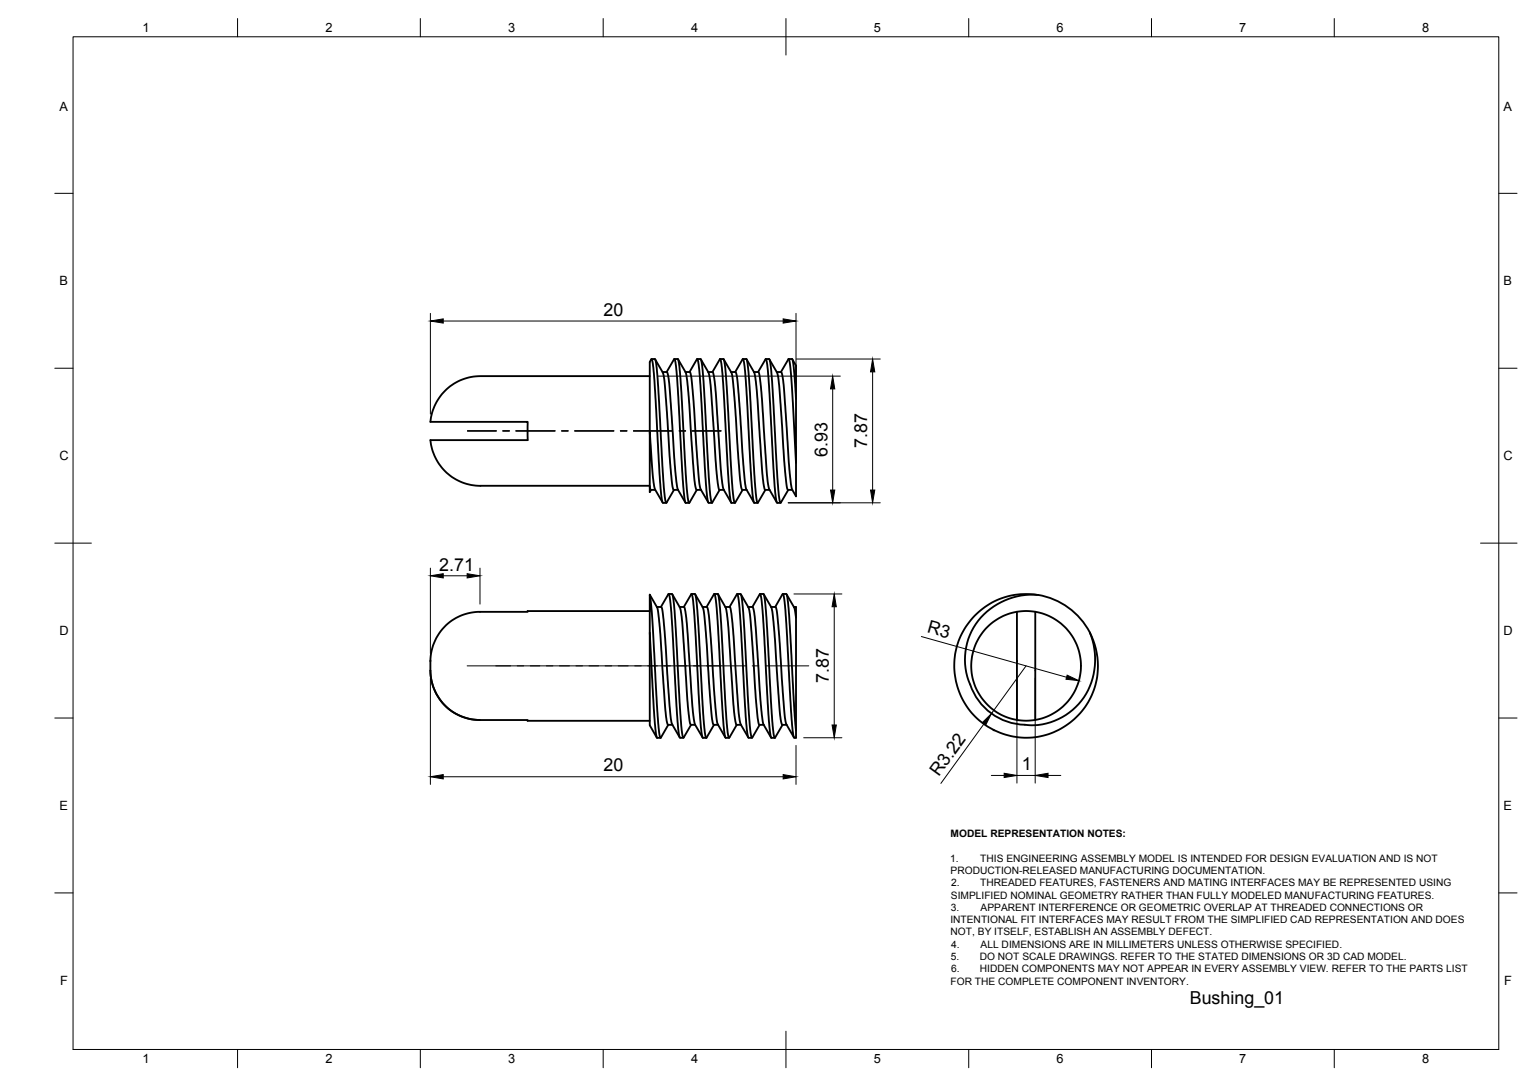
ISO-10303-21;
HEADER;
/* Generated by software containing ST-Developer
 * from STEP Tools, Inc. (www.steptools.com) 
 */

FILE_DESCRIPTION(
/* description */ (''),
/* implementation_level */ '2;1');

FILE_NAME(
/* name */ 'Bushing_01.step',
/* time_stamp */ '2026-10-06T12:52:28-07:00',
/* author */ (''),
/* organization */ (''),
/* preprocessor_version */ 'ST-DEVELOPER v20.2',
/* originating_system */ 'Autodesk Translation Framework v15.15.0.0',
/* authorisation */ '');

FILE_SCHEMA (('AUTOMOTIVE_DESIGN { 1 0 10303 214 3 1 1 }'));
ENDSEC;

DATA;
#10=MECHANICAL_DESIGN_GEOMETRIC_PRESENTATION_REPRESENTATION('',(#77),#34403);
#47=B_SPLINE_SURFACE_WITH_KNOTS('',3,3,((#18145,#18146,#18147,#18148,#18149,
#18150,#18151,#18152,#18153),(#18154,#18155,#18156,#18157,#18158,#18159,
#18160,#18161,#18162),(#18163,#18164,#18165,#18166,#18167,#18168,#18169,
#18170,#18171),(#18172,#18173,#18174,#18175,#18176,#18177,#18178,#18179,
#18180),(#18181,#18182,#18183,#18184,#18185,#18186,#18187,#18188,#18189)),
 .UNSPECIFIED.,.F.,.F.,.F.,(4,1,4),(4,1,1,1,1,1,4),(-2.31295147948379E-5,
0.571428571428571,1.),(-0.0392722280793192,-0.0280568740573752,-0.00562616601348723,
0.00558918800845676,0.0168045420304008,0.0280198960523448,0.0392352500742888),
 .UNSPECIFIED.);
#48=B_SPLINE_SURFACE_WITH_KNOTS('',3,3,((#18360,#18361,#18362,#18363,#18364,
#18365,#18366,#18367,#18368,#18369),(#18370,#18371,#18372,#18373,#18374,
#18375,#18376,#18377,#18378,#18379),(#18380,#18381,#18382,#18383,#18384,
#18385,#18386,#18387,#18388,#18389),(#18390,#18391,#18392,#18393,#18394,
#18395,#18396,#18397,#18398,#18399),(#18400,#18401,#18402,#18403,#18404,
#18405,#18406,#18407,#18408,#18409)),.UNSPECIFIED.,.F.,.F.,.F.,(4,1,4),
(4,1,1,1,1,1,1,4),(-2.35337788502184E-5,0.571428571428571,1.),(-0.0392722280793192,
-0.0280568740573752,-0.0168415200354311,-0.00562616601348712,0.0055891880084569,
0.0168045420304009,0.0280198960523449,0.0392352500742889),.UNSPECIFIED.);
#49=B_SPLINE_SURFACE_WITH_KNOTS('',3,3,((#18444,#18445,#18446,#18447,#18448,
#18449,#18450,#18451,#18452,#18453,#18454,#18455,#18456,#18457,#18458,#18459,
#18460,#18461,#18462,#18463,#18464,#18465,#18466,#18467,#18468,#18469,#18470,
#18471,#18472,#18473,#18474,#18475,#18476,#18477,#18478,#18479,#18480,#18481,
#18482,#18483,#18484,#18485,#18486,#18487,#18488,#18489),(#18490,#18491,
#18492,#18493,#18494,#18495,#18496,#18497,#18498,#18499,#18500,#18501,#18502,
#18503,#18504,#18505,#18506,#18507,#18508,#18509,#18510,#18511,#18512,#18513,
#18514,#18515,#18516,#18517,#18518,#18519,#18520,#18521,#18522,#18523,#18524,
#18525,#18526,#18527,#18528,#18529,#18530,#18531,#18532,#18533,#18534,#18535),
(#18536,#18537,#18538,#18539,#18540,#18541,#18542,#18543,#18544,#18545,
#18546,#18547,#18548,#18549,#18550,#18551,#18552,#18553,#18554,#18555,#18556,
#18557,#18558,#18559,#18560,#18561,#18562,#18563,#18564,#18565,#18566,#18567,
#18568,#18569,#18570,#18571,#18572,#18573,#18574,#18575,#18576,#18577,#18578,
#18579,#18580,#18581),(#18582,#18583,#18584,#18585,#18586,#18587,#18588,
#18589,#18590,#18591,#18592,#18593,#18594,#18595,#18596,#18597,#18598,#18599,
#18600,#18601,#18602,#18603,#18604,#18605,#18606,#18607,#18608,#18609,#18610,
#18611,#18612,#18613,#18614,#18615,#18616,#18617,#18618,#18619,#18620,#18621,
#18622,#18623,#18624,#18625,#18626,#18627)),.UNSPECIFIED.,.F.,.F.,.F.,(4,
4),(4,1,1,1,1,1,1,1,1,1,1,1,1,1,1,1,1,1,1,1,1,1,1,1,1,1,1,1,1,1,1,1,1,1,
1,1,1,1,1,1,1,1,1,4),(-0.000633807887895752,0.0823317564776454),(8.31473274985803,
9.29783943738047,10.2809461249029,11.2640528124254,12.2471594999478,13.2302661874702,
14.2133728749927,15.1964795625151,16.1795862500376,17.16269293756,18.1457996250825,
19.1289063126049,20.1120130001274,21.0951196876498,22.0782263751723,23.0613330626947,
24.0444397502171,25.0275464377396,26.010653125262,26.9937598127845,27.9768665003069,
28.9599731878294,29.9430798753518,30.9261865628743,31.9092932503967,32.8923999379191,
33.8755066254416,34.858613312964,35.8417200004865,36.8248266880089,37.8079333755314,
38.7910400630538,39.7741467505763,40.7572534380987,41.7403601256211,42.7234668131436,
43.706573500666,44.6896801881885,45.6727868757109,46.6558935632334,47.6390002507558,
48.6221069382783,49.6052136258007,50.5889541212111),.UNSPECIFIED.);
#50=B_SPLINE_SURFACE_WITH_KNOTS('',3,3,((#18809,#18810,#18811,#18812,#18813,
#18814,#18815,#18816,#18817,#18818,#18819,#18820,#18821,#18822,#18823,#18824,
#18825,#18826,#18827,#18828,#18829,#18830,#18831,#18832,#18833,#18834,#18835,
#18836,#18837,#18838,#18839,#18840,#18841,#18842,#18843,#18844,#18845,#18846,
#18847,#18848,#18849,#18850,#18851,#18852,#18853,#18854),(#18855,#18856,
#18857,#18858,#18859,#18860,#18861,#18862,#18863,#18864,#18865,#18866,#18867,
#18868,#18869,#18870,#18871,#18872,#18873,#18874,#18875,#18876,#18877,#18878,
#18879,#18880,#18881,#18882,#18883,#18884,#18885,#18886,#18887,#18888,#18889,
#18890,#18891,#18892,#18893,#18894,#18895,#18896,#18897,#18898,#18899,#18900),
(#18901,#18902,#18903,#18904,#18905,#18906,#18907,#18908,#18909,#18910,
#18911,#18912,#18913,#18914,#18915,#18916,#18917,#18918,#18919,#18920,#18921,
#18922,#18923,#18924,#18925,#18926,#18927,#18928,#18929,#18930,#18931,#18932,
#18933,#18934,#18935,#18936,#18937,#18938,#18939,#18940,#18941,#18942,#18943,
#18944,#18945,#18946),(#18947,#18948,#18949,#18950,#18951,#18952,#18953,
#18954,#18955,#18956,#18957,#18958,#18959,#18960,#18961,#18962,#18963,#18964,
#18965,#18966,#18967,#18968,#18969,#18970,#18971,#18972,#18973,#18974,#18975,
#18976,#18977,#18978,#18979,#18980,#18981,#18982,#18983,#18984,#18985,#18986,
#18987,#18988,#18989,#18990,#18991,#18992)),.UNSPECIFIED.,.F.,.F.,.F.,(4,
4),(4,1,1,1,1,1,1,1,1,1,1,1,1,1,1,1,1,1,1,1,1,1,1,1,1,1,1,1,1,1,1,1,1,1,
1,1,1,1,1,1,1,1,1,4),(-0.000319018948610172,0.0826465308545402),(11.6145803026385,
12.5983209152772,13.5814276027996,14.564534290322,15.5476409778445,16.5307476653669,
17.5138543528894,18.4969610404118,19.4800677279343,20.4631744154567,21.4462811029792,
22.4293877905016,23.4124944780241,24.3956011655465,25.3787078530689,26.3618145405914,
27.3449212281138,28.3280279156363,29.3111346031587,30.2942412906812,31.2773479782036,
32.2604546657261,33.2435613532485,34.226668040771,35.2097747282934,36.1928814158158,
37.1759881033383,38.1590947908607,39.1422014783832,40.1253081659056,41.1084148534281,
42.0915215409505,43.074628228473,44.0577349159954,45.0408416035178,46.0239482910403,
47.0070549785627,47.9901616660852,48.9732683536076,49.9563750411301,50.9394817286525,
51.922588416175,52.9056951036974,53.8888017912198),.UNSPECIFIED.);
#61=SHAPE_REPRESENTATION_RELATIONSHIP('SRR','None',#34439,#69);
#69=ADVANCED_BREP_SHAPE_REPRESENTATION('',(#85),#34399);
#77=STYLED_ITEM('',(#34484),#85);
#85=MANIFOLD_SOLID_BREP('Body1',#4386);
#100=FACE_BOUND('',#818,.T.);
#135=PLANE('',#4570);
#136=PLANE('',#4574);
#137=PLANE('',#4577);
#138=PLANE('',#4578);
#192=CIRCLE('',#4559,3.22275);
#193=CIRCLE('',#4566,3.933);
#194=CIRCLE('',#4567,3.933);
#195=CIRCLE('',#4569,3.22275);
#196=CIRCLE('',#4571,24.5);
#197=CIRCLE('',#4573,3.);
#198=CIRCLE('',#4575,24.5);
#559=FACE_OUTER_BOUND('',#801,.T.);
#560=FACE_OUTER_BOUND('',#802,.T.);
#561=FACE_OUTER_BOUND('',#803,.T.);
#562=FACE_OUTER_BOUND('',#804,.T.);
#563=FACE_OUTER_BOUND('',#805,.T.);
#564=FACE_OUTER_BOUND('',#806,.T.);
#565=FACE_OUTER_BOUND('',#807,.T.);
#566=FACE_OUTER_BOUND('',#808,.T.);
#567=FACE_OUTER_BOUND('',#809,.T.);
#568=FACE_OUTER_BOUND('',#810,.T.);
#569=FACE_OUTER_BOUND('',#811,.T.);
#570=FACE_OUTER_BOUND('',#812,.T.);
#571=FACE_OUTER_BOUND('',#813,.T.);
#572=FACE_OUTER_BOUND('',#814,.T.);
#573=FACE_OUTER_BOUND('',#815,.T.);
#574=FACE_OUTER_BOUND('',#816,.T.);
#575=FACE_OUTER_BOUND('',#817,.T.);
#576=FACE_OUTER_BOUND('',#819,.T.);
#801=EDGE_LOOP('',(#2953,#2954,#2955,#2956));
#802=EDGE_LOOP('',(#2957,#2958,#2959,#2960));
#803=EDGE_LOOP('',(#2961,#2962,#2963,#2964));
#804=EDGE_LOOP('',(#2965,#2966,#2967,#2968));
#805=EDGE_LOOP('',(#2969,#2970,#2971,#2972));
#806=EDGE_LOOP('',(#2973,#2974,#2975,#2976));
#807=EDGE_LOOP('',(#2977,#2978,#2979,#2980,#2981,#2982,#2983,#2984,#2985,
#2986,#2987,#2988,#2989,#2990,#2991,#2992,#2993,#2994));
#808=EDGE_LOOP('',(#2995,#2996,#2997,#2998));
#809=EDGE_LOOP('',(#2999,#3000,#3001,#3002));
#810=EDGE_LOOP('',(#3003,#3004,#3005,#3006,#3007,#3008));
#811=EDGE_LOOP('',(#3009,#3010,#3011,#3012,#3013,#3014,#3015,#3016,#3017,
#3018,#3019,#3020));
#812=EDGE_LOOP('',(#3021,#3022,#3023,#3024,#3025));
#813=EDGE_LOOP('',(#3026,#3027,#3028,#3029,#3030,#3031));
#814=EDGE_LOOP('',(#3032,#3033,#3034,#3035));
#815=EDGE_LOOP('',(#3036,#3037,#3038,#3039,#3040,#3041,#3042,#3043,#3044,
#3045,#3046,#3047,#3048,#3049,#3050,#3051,#3052,#3053));
#816=EDGE_LOOP('',(#3054,#3055,#3056,#3057,#3058,#3059,#3060,#3061,#3062,
#3063,#3064,#3065,#3066,#3067,#3068,#3069,#3070,#3071));
#817=EDGE_LOOP('',(#3072,#3073,#3074,#3075,#3076));
#818=EDGE_LOOP('',(#3077));
#819=EDGE_LOOP('',(#3078,#3079,#3080,#3081,#3082));
#1040=LINE('',#13648,#1177);
#1041=LINE('',#13847,#1178);
#1042=LINE('',#14169,#1179);
#1043=LINE('',#14491,#1180);
#1044=LINE('',#14817,#1181);
#1045=LINE('',#15137,#1182);
#1046=LINE('',#18231,#1183);
#1047=LINE('',#18234,#1184);
#1048=LINE('',#18237,#1185);
#1049=LINE('',#18291,#1186);
#1050=LINE('',#18307,#1187);
#1051=LINE('',#18358,#1188);
#1052=LINE('',#18440,#1189);
#1177=VECTOR('',#5189,3.22275);
#1178=VECTOR('',#5194,3.22275);
#1179=VECTOR('',#5197,3.22275);
#1180=VECTOR('',#5200,3.22275);
#1181=VECTOR('',#5203,3.22275);
#1182=VECTOR('',#5206,3.22275);
#1183=VECTOR('',#5217,10.);
#1184=VECTOR('',#5220,10.);
#1185=VECTOR('',#5223,10.);
#1186=VECTOR('',#5226,10.);
#1187=VECTOR('',#5227,10.);
#1188=VECTOR('',#5228,3.);
#1189=VECTOR('',#5231,10.);
#1365=B_SPLINE_CURVE_WITH_KNOTS('',3,(#13650,#13651,#13652,#13653,#13654,
#13655,#13656,#13657,#13658,#13659,#13660,#13661,#13662,#13663,#13664,#13665,
#13666,#13667,#13668,#13669,#13670,#13671,#13672,#13673,#13674,#13675,#13676,
#13677,#13678,#13679,#13680,#13681,#13682,#13683,#13684,#13685,#13686,#13687,
#13688,#13689,#13690,#13691,#13692,#13693,#13694,#13695,#13696,#13697,#13698,
#13699,#13700,#13701,#13702,#13703,#13704,#13705,#13706,#13707,#13708,#13709,
#13710,#13711,#13712,#13713,#13714,#13715,#13716,#13717,#13718,#13719,#13720,
#13721,#13722,#13723,#13724,#13725,#13726,#13727,#13728,#13729,#13730,#13731,
#13732,#13733,#13734,#13735,#13736,#13737,#13738,#13739,#13740,#13741,#13742,
#13743,#13744,#13745,#13746,#13747,#13748,#13749,#13750,#13751,#13752,#13753,
#13754,#13755,#13756,#13757,#13758,#13759),.UNSPECIFIED.,.F.,.F.,(4,2,2,
2,2,2,2,2,2,2,2,2,2,2,2,2,2,2,2,2,2,2,2,2,2,2,2,2,2,2,2,2,2,2,2,2,2,2,2,
2,2,2,2,2,2,2,2,2,2,2,2,2,2,2,4),(-1.46839216655186,-1.42833493122557,-1.40983960309952,
-1.39649008476235,-1.38192245258612,-1.35595026682801,-1.32006579388245,
-1.25739415958123,-1.24599994074249,-1.23838263735435,-1.2292335836828,
-1.20895486413597,-1.17609120945209,-1.11172712552003,-1.09300158666968,
-1.07960228916858,-1.06507837657971,-1.03947664653156,-1.00445705495045,
-0.941126403182701,-0.929252655631959,-0.921667552812672,-0.912906557233483,
-0.894754745947669,-0.867289011584784,-0.789797140050929,-0.772858151395854,
-0.759724672664605,-0.744718751329267,-0.715589302934294,-0.671818863481682,
-0.624725490925685,-0.612046960332389,-0.605030943441965,-0.596793484943762,
-0.581814683947116,-0.521809333456173,-0.475770727809289,-0.456880324092417,
-0.443431024636274,-0.428912818539185,-0.40347690482787,-0.368790757052006,
-0.305998460037176,-0.293741810698422,-0.286007401773675,-0.277001834303914,
-0.2582504497825,-0.229364741447431,-0.158963286891711,-0.141351957341446,
-0.127920650801248,-0.112746328135276,-0.0837659472426957,-0.00482640158894297),
 .UNSPECIFIED.);
#1366=B_SPLINE_CURVE_WITH_KNOTS('',3,(#13762,#13763,#13764,#13765,#13766,
#13767,#13768,#13769,#13770,#13771,#13772,#13773,#13774,#13775,#13776,#13777,
#13778,#13779,#13780,#13781,#13782,#13783,#13784,#13785,#13786,#13787,#13788,
#13789,#13790,#13791,#13792,#13793,#13794,#13795,#13796,#13797,#13798,#13799,
#13800,#13801,#13802,#13803,#13804,#13805,#13806,#13807,#13808,#13809,#13810,
#13811,#13812,#13813,#13814,#13815,#13816,#13817,#13818,#13819,#13820,#13821,
#13822,#13823,#13824,#13825,#13826,#13827,#13828,#13829,#13830,#13831,#13832,
#13833,#13834,#13835,#13836,#13837,#13838,#13839,#13840,#13841,#13842,#13843),
 .UNSPECIFIED.,.F.,.F.,(4,2,2,2,2,2,2,2,2,2,2,2,2,2,2,2,2,2,2,2,2,2,2,2,
2,2,2,2,2,2,2,2,2,2,2,2,2,2,2,2,4),(-12.9928680261101,-12.9859224043785,
-12.9767663441379,-12.9317684829387,-12.8787491107298,-12.8585962440726,
-12.843864647075,-12.8272831513426,-12.7952673642781,-12.7272779370865,
-12.7034734144216,-12.6867491934808,-12.6781417326004,-12.6706722689398,
-12.6588036168692,-12.5925791120038,-12.559965517409,-12.5357561764214,
-12.5219312356032,-12.5092183047936,-12.4916768823375,-12.4031982185048,
-12.3811372405126,-12.3655143239889,-12.3574349585401,-12.3497117864246,
-12.3373035405743,-12.2745292128648,-12.239536256517,-12.2138553471672,
-12.1992108316161,-12.185635321062,-12.1695331810739,-12.0996377675633,
-12.0705351122928,-12.0517005184064,-12.0426844314299,-12.034958762972,
-12.0227451090155,-11.9599676349854,-11.9265167435349),.UNSPECIFIED.);
#1367=B_SPLINE_CURVE_WITH_KNOTS('',3,(#13848,#13849,#13850,#13851,#13852,
#13853,#13854,#13855,#13856,#13857,#13858,#13859,#13860,#13861,#13862,#13863,
#13864,#13865,#13866,#13867,#13868,#13869,#13870,#13871,#13872,#13873,#13874,
#13875,#13876,#13877,#13878,#13879,#13880,#13881,#13882,#13883,#13884,#13885,
#13886,#13887,#13888,#13889,#13890,#13891,#13892,#13893,#13894,#13895,#13896,
#13897,#13898,#13899,#13900,#13901,#13902,#13903,#13904,#13905,#13906,#13907,
#13908,#13909,#13910,#13911,#13912,#13913,#13914,#13915,#13916,#13917,#13918,
#13919,#13920,#13921,#13922,#13923,#13924,#13925,#13926,#13927,#13928,#13929,
#13930,#13931,#13932,#13933,#13934,#13935,#13936,#13937,#13938,#13939,#13940,
#13941,#13942,#13943,#13944,#13945,#13946,#13947,#13948,#13949,#13950,#13951,
#13952,#13953,#13954,#13955,#13956,#13957,#13958,#13959,#13960,#13961,#13962,
#13963,#13964,#13965,#13966,#13967,#13968,#13969,#13970,#13971,#13972,#13973,
#13974,#13975,#13976,#13977,#13978,#13979,#13980,#13981,#13982,#13983,#13984,
#13985,#13986,#13987,#13988,#13989,#13990,#13991,#13992,#13993,#13994,#13995,
#13996,#13997,#13998,#13999,#14000,#14001,#14002,#14003,#14004,#14005,#14006,
#14007),.UNSPECIFIED.,.F.,.F.,(4,2,2,2,2,2,2,2,2,2,2,2,2,2,2,2,2,2,2,2,
2,2,2,2,2,2,2,2,2,2,2,2,2,2,2,2,2,2,2,2,2,2,2,2,2,2,2,2,2,2,2,2,2,2,2,2,
2,2,2,2,2,2,2,2,2,2,2,2,2,2,2,2,2,2,2,2,2,2,2,4),(-3.49867878100114,-3.48078195894374,
-3.46955972522698,-3.46197286794586,-3.45277159842556,-3.43205243267988,
-3.39797610063354,-3.33546990288741,-3.31654806244602,-3.30313938427867,
-3.28872610459223,-3.263693666223,-3.22988764964021,-3.16560395356786,-3.15313346501676,
-3.14544256963846,-3.13683534548366,-3.11979450354527,-3.09492308948557,
-3.01527193149294,-2.99739186424985,-2.98411787341524,-2.96928256762587,
-2.94165310746421,-2.90187154715814,-2.84744108782649,-2.83519835180177,
-2.82754492556646,-2.81885783486495,-2.80134935179091,-2.77541919752302,
-2.69874979137671,-2.68038057439865,-2.66704941358868,-2.65243562926348,
-2.6261741549808,-2.58964121940858,-2.52834010486826,-2.51679218417816,
-2.50916638327307,-2.50014259245465,-2.48058056285362,-2.44963644828718,
-2.38085364722827,-2.36257423529482,-2.3492540741215,-2.33460217519332,
-2.30810824640674,-2.27103873044209,-2.21095127043577,-2.19926909881182,
-2.19162334288848,-2.18265751788382,-2.1634770024513,-2.13351351801827,
-2.06259963370997,-2.04459412536108,-2.03130461939912,-2.016525598512,-1.98925576826921,
-1.95035384678123,-1.89421291245162,-1.88210670171816,-1.87447641278316,
-1.86574577853761,-1.84795589000478,-1.82136965309309,-1.74647395934031,
-1.72781643493424,-1.71445588254354,-1.69997280638284,-1.67445876507744,
-1.6395921546019,-1.57666462581832,-1.56449569108919,-1.55685831797228,
-1.54815224960004,-1.53052436699322,-1.50432028007254,-1.46839216655186),
 .UNSPECIFIED.);
#1368=B_SPLINE_CURVE_WITH_KNOTS('',3,(#14008,#14009,#14010,#14011,#14012,
#14013,#14014,#14015,#14016,#14017,#14018,#14019,#14020,#14021,#14022,#14023,
#14024,#14025,#14026,#14027,#14028,#14029,#14030,#14031,#14032,#14033,#14034,
#14035,#14036,#14037,#14038,#14039,#14040,#14041,#14042,#14043,#14044,#14045,
#14046,#14047,#14048,#14049,#14050,#14051,#14052,#14053,#14054,#14055,#14056,
#14057,#14058,#14059,#14060,#14061,#14062,#14063,#14064,#14065,#14066,#14067,
#14068,#14069,#14070,#14071,#14072,#14073,#14074,#14075,#14076,#14077,#14078,
#14079,#14080,#14081,#14082,#14083,#14084,#14085,#14086,#14087,#14088,#14089,
#14090,#14091,#14092,#14093,#14094,#14095,#14096,#14097,#14098,#14099,#14100,
#14101,#14102,#14103,#14104,#14105,#14106,#14107,#14108,#14109,#14110,#14111,
#14112,#14113,#14114,#14115,#14116,#14117,#14118,#14119,#14120,#14121,#14122,
#14123,#14124,#14125,#14126,#14127,#14128,#14129,#14130,#14131,#14132,#14133,
#14134,#14135,#14136,#14137,#14138,#14139,#14140,#14141,#14142,#14143,#14144,
#14145,#14146,#14147,#14148,#14149,#14150,#14151,#14152,#14153,#14154,#14155,
#14156,#14157,#14158,#14159,#14160,#14161,#14162,#14163,#14164,#14165),
 .UNSPECIFIED.,.F.,.F.,(4,2,2,2,2,2,2,2,2,2,2,2,2,2,2,2,2,2,2,2,2,2,2,2,
2,2,2,2,2,2,2,2,2,2,2,2,2,2,2,2,2,2,2,2,2,2,2,2,2,2,2,2,2,2,2,2,2,2,2,2,
2,2,2,2,2,2,2,2,2,2,2,2,2,2,2,2,2,2,4),(-11.9265167435349,-11.9253010671319,
-11.8998775010244,-11.8853659903058,-11.8719222083261,-11.853038636317,
-11.8070670854776,-11.7469950171144,-11.732009875923,-11.7237734567874,
-11.7167614908132,-11.7040962421554,-11.657144644663,-11.613348594958,-11.5842158731154,
-11.5692140131739,-11.5560858712183,-11.5391563059077,-11.4616146846684,
-11.4341620971523,-11.4160188349624,-11.4072614323029,-11.3996791529454,
-11.3878096466355,-11.3295052301493,-11.2916491109299,-11.2648076084194,
-11.2500856128337,-11.2367575434473,-11.2185487998283,-11.1495201728474,
-11.1188782881042,-11.0994366818601,-11.0904187427783,-11.0827715924609,
-11.0711299783697,-11.0108006877799,-10.9739293014615,-10.9475272769351,
-10.9328929903791,-10.919570571438,-10.9012581537384,-10.8241647393242,
-10.7983532562927,-10.7808988714022,-10.7722242463342,-10.7645771798208,
-10.7523362255452,-10.6981722958883,-10.6583176476268,-10.6306685501689,
-10.6158432715508,-10.602589118057,-10.5847552249583,-10.5125151252235,
-10.4830685178717,-10.4640972285704,-10.4551729237098,-10.4475245495813,
-10.4357933954727,-10.3762476656135,-10.3389794411438,-10.3124002139746,
-10.2977349418755,-10.2844183959626,-10.2661684350075,-10.1971897108364,
-10.1663518150652,-10.1468330124204,-10.137815162146,-10.1301865446066,
-10.1186200205451,-10.057586096903,-10.0209901905299,-9.99470377217364,
-9.98008828052383,-9.96676098275258,-9.94840609177415,-9.89731205748756),
 .UNSPECIFIED.);
#1369=B_SPLINE_CURVE_WITH_KNOTS('',3,(#14170,#14171,#14172,#14173,#14174,
#14175,#14176,#14177,#14178,#14179,#14180,#14181,#14182,#14183,#14184,#14185,
#14186,#14187,#14188,#14189,#14190,#14191,#14192,#14193,#14194,#14195,#14196,
#14197,#14198,#14199,#14200,#14201,#14202,#14203,#14204,#14205,#14206,#14207,
#14208,#14209,#14210,#14211,#14212,#14213,#14214,#14215,#14216,#14217,#14218,
#14219,#14220,#14221,#14222,#14223,#14224,#14225,#14226,#14227,#14228,#14229,
#14230,#14231,#14232,#14233,#14234,#14235,#14236,#14237,#14238,#14239,#14240,
#14241,#14242,#14243,#14244,#14245,#14246,#14247,#14248,#14249,#14250,#14251,
#14252,#14253,#14254,#14255,#14256,#14257,#14258,#14259,#14260,#14261,#14262,
#14263,#14264,#14265,#14266,#14267,#14268,#14269,#14270,#14271,#14272,#14273,
#14274,#14275,#14276,#14277,#14278,#14279,#14280,#14281,#14282,#14283,#14284,
#14285,#14286,#14287,#14288,#14289,#14290,#14291,#14292,#14293,#14294,#14295,
#14296,#14297,#14298,#14299,#14300,#14301,#14302,#14303,#14304,#14305,#14306,
#14307,#14308,#14309,#14310,#14311,#14312,#14313,#14314,#14315,#14316,#14317,
#14318,#14319,#14320,#14321,#14322,#14323,#14324,#14325,#14326,#14327),
 .UNSPECIFIED.,.F.,.F.,(4,2,2,2,2,2,2,2,2,2,2,2,2,2,2,2,2,2,2,2,2,2,2,2,
2,2,2,2,2,2,2,2,2,2,2,2,2,2,2,2,2,2,2,2,2,2,2,2,2,2,2,2,2,2,2,2,2,2,2,2,
2,2,2,2,2,2,2,2,2,2,2,2,2,2,2,2,2,2,4),(-5.52967993174404,-5.52746103895827,
-5.51301726605171,-5.48781751392462,-5.45365608075187,-5.39023974331564,
-5.37763154077627,-5.37060511658607,-5.36232751823559,-5.34710774761743,
-5.32609931402627,-5.2862261887768,-5.24174894981634,-5.22298786851781,
-5.2095987033326,-5.19512334302082,-5.16973497836552,-5.13516395069695,
-5.07314639039331,-5.06018581576942,-5.05310310809778,-5.04492307594188,
-5.03021949666535,-5.01023868726809,-4.94186884287386,-4.91337098939853,
-4.89839769785815,-4.88514869317986,-4.86752871096216,-4.80838931035308,
-4.75396056823127,-4.74171236882094,-4.734055979712,-4.72536542702825,-4.70785112905183,
-4.68191322298387,-4.60521466097691,-4.58683882554718,-4.57350193498445,
-4.5588808435482,-4.53260225217019,-4.49603942555881,-4.43475512973231,
-4.42319834572813,-4.41556866284627,-4.40654243879864,-4.38698036174205,
-4.35604271661056,-4.28721316259916,-4.26893202003434,-4.25560773622987,
-4.24094857896087,-4.21443280452239,-4.17732242330325,-4.11726652960083,
-4.10557436659351,-4.0979264437805,-4.08896619952871,-4.06982003452643,
-4.03994975453202,-3.96871964483552,-3.95074163312683,-3.93745485665172,
-3.92266291296092,-3.89531644100836,-3.85623277292381,-3.80042416657247,
-3.7882820156738,-3.78064331846076,-3.7719145791267,-3.75417031696167,-3.7276991511797,
-3.65248254650758,-3.63386775502272,-3.62050141253184,-3.60597794025483,
-3.58028256336171,-3.54503001769459,-3.49867878100114),.UNSPECIFIED.);
#1370=B_SPLINE_CURVE_WITH_KNOTS('',3,(#14328,#14329,#14330,#14331,#14332,
#14333,#14334,#14335,#14336,#14337,#14338,#14339,#14340,#14341,#14342,#14343,
#14344,#14345,#14346,#14347,#14348,#14349,#14350,#14351,#14352,#14353,#14354,
#14355,#14356,#14357,#14358,#14359,#14360,#14361,#14362,#14363,#14364,#14365,
#14366,#14367,#14368,#14369,#14370,#14371,#14372,#14373,#14374,#14375,#14376,
#14377,#14378,#14379,#14380,#14381,#14382,#14383,#14384,#14385,#14386,#14387,
#14388,#14389,#14390,#14391,#14392,#14393,#14394,#14395,#14396,#14397,#14398,
#14399,#14400,#14401,#14402,#14403,#14404,#14405,#14406,#14407,#14408,#14409,
#14410,#14411,#14412,#14413,#14414,#14415,#14416,#14417,#14418,#14419,#14420,
#14421,#14422,#14423,#14424,#14425,#14426,#14427,#14428,#14429,#14430,#14431,
#14432,#14433,#14434,#14435,#14436,#14437,#14438,#14439,#14440,#14441,#14442,
#14443,#14444,#14445,#14446,#14447,#14448,#14449,#14450,#14451,#14452,#14453,
#14454,#14455,#14456,#14457,#14458,#14459,#14460,#14461,#14462,#14463,#14464,
#14465,#14466,#14467,#14468,#14469,#14470,#14471,#14472,#14473,#14474,#14475,
#14476,#14477,#14478,#14479,#14480,#14481,#14482,#14483,#14484,#14485,#14486,
#14487),.UNSPECIFIED.,.F.,.F.,(4,2,2,2,2,2,2,2,2,2,2,2,2,2,2,2,2,2,2,2,
2,2,2,2,2,2,2,2,2,2,2,2,2,2,2,2,2,2,2,2,2,2,2,2,2,2,2,2,2,2,2,2,2,2,2,2,
2,2,2,2,2,2,2,2,2,2,2,2,2,2,2,2,2,2,2,2,2,2,2,4),(-9.89731205748756,-9.87162361382395,
-9.84571672148278,-9.8282203325955,-9.81953673147491,-9.81188557016175,
-9.79964504010395,-9.7453353927449,-9.68588701052147,-9.66840892468634,
-9.65518233720158,-9.64014951983856,-9.61121679086927,-9.54710288205336,
-9.52518442005323,-9.50952273187202,-9.50116641415943,-9.49323726967608,
-9.47984096142707,-9.41841483438956,-9.38405272533443,-9.35876460570814,
-9.34431150527036,-9.33092351702992,-9.31213081036045,-9.26682809174202,
-9.20592344878349,-9.19124586497382,-9.18307356778884,-9.17599233018182,
-9.16302464101464,-9.1010926825414,-9.06656652339253,-9.04120314257779,
-9.02673764776751,-9.0133547716598,-8.99459796382821,-8.93015897051987,
-8.89709054613671,-8.87673519280996,-8.86758962770716,-8.85999320107415,
-8.84867813277258,-8.7853386484155,-8.7497414683527,-8.72389307464899,-8.70934690228895,
-8.69599256884213,-8.67745006654022,-8.61089742105274,-8.57888085009621,
-8.5589128575847,-8.5498257876899,-8.54221504342842,-8.53078833786196,-8.46843943241757,
-8.43240433177706,-8.40636060077543,-8.39178154341029,-8.37843687642808,
-8.35997416897036,-8.29268815485724,-8.26101887053062,-8.24118064506504,
-8.23211306100547,-8.22449675695535,-8.21303015286522,-8.1510306685194,
-8.11483687606373,-8.08872245947601,-8.07413118823732,-8.06078943327742,
-8.04235415192669,-7.96600531183447,-7.93992674806435,-7.92235335104717,
-7.91365413696589,-7.90600425157219,-7.89378828854135,-7.86715098468372),
 .UNSPECIFIED.);
#1371=B_SPLINE_CURVE_WITH_KNOTS('',3,(#14492,#14493,#14494,#14495,#14496,
#14497,#14498,#14499,#14500,#14501,#14502,#14503,#14504,#14505,#14506,#14507,
#14508,#14509,#14510,#14511,#14512,#14513,#14514,#14515,#14516,#14517,#14518,
#14519,#14520,#14521,#14522,#14523,#14524,#14525,#14526,#14527,#14528,#14529,
#14530,#14531,#14532,#14533,#14534,#14535,#14536,#14537,#14538,#14539,#14540,
#14541,#14542,#14543,#14544,#14545,#14546,#14547,#14548,#14549,#14550,#14551,
#14552,#14553,#14554,#14555,#14556,#14557,#14558,#14559,#14560,#14561,#14562,
#14563,#14564,#14565,#14566,#14567,#14568,#14569,#14570,#14571,#14572,#14573,
#14574,#14575,#14576,#14577,#14578,#14579,#14580,#14581,#14582,#14583,#14584,
#14585,#14586,#14587,#14588,#14589,#14590,#14591,#14592,#14593,#14594,#14595,
#14596,#14597,#14598,#14599,#14600,#14601,#14602,#14603,#14604,#14605,#14606,
#14607,#14608,#14609,#14610,#14611,#14612,#14613,#14614,#14615,#14616,#14617,
#14618,#14619,#14620,#14621,#14622,#14623,#14624,#14625,#14626,#14627,#14628,
#14629,#14630,#14631,#14632,#14633,#14634,#14635,#14636,#14637,#14638,#14639,
#14640,#14641,#14642,#14643,#14644,#14645,#14646,#14647,#14648,#14649,#14650,
#14651),.UNSPECIFIED.,.F.,.F.,(4,2,2,2,2,2,2,2,2,2,2,2,2,2,2,2,2,2,2,2,
2,2,2,2,2,2,2,2,2,2,2,2,2,2,2,2,2,2,2,2,2,2,2,2,2,2,2,2,2,2,2,2,2,2,2,2,
2,2,2,2,2,2,2,2,2,2,2,2,2,2,2,2,2,2,2,2,2,2,2,4),(-7.56063401821517,-7.51326854468081,
-7.47889664780859,-7.45359951190156,-7.43914016392443,-7.42574589017486,
-7.40694368778009,-7.36161669798204,-7.30067761794024,-7.28599267208735,
-7.27781655497411,-7.27073204834674,-7.25775916081779,-7.19579411210642,
-7.16124964460926,-7.13587298253407,-7.12140006118494,-7.10801038971074,
-7.0892441541453,-7.04472824612105,-7.00474258976706,-6.98378365646472,
-6.96858944035981,-6.96031683320164,-6.95328802084185,-6.94066412593651,
-6.89833220805518,-6.85135167914178,-6.82105128320064,-6.80580836526909,
-6.79260293075702,-6.77574081761993,-6.7276501901097,-6.67999965453028,
-6.65519724829239,-6.6454479770827,-6.63792609692965,-6.62749571660404,
-6.59724519229377,-6.55192602821455,-6.52190715245824,-6.49871346520397,
-6.48460762258951,-6.47103373223388,-6.45103494619549,-6.42691901801644,
-6.36458802981141,-6.33838427503928,-6.32835459325203,-6.32083982459997,
-6.31089899367771,-6.28442624894019,-6.22954117660892,-6.19013440566297,
-6.17337352547654,-6.16019510881402,-6.14468271966448,-6.11247320760936,
-6.05940469690626,-6.02237763351456,-6.01146819552367,-6.00391204078825,
-5.99451476760146,-5.97243911025324,-5.934347640682,-5.87826230434033,-5.8590946363509,
-5.84564737810772,-5.83130860327909,-5.80673925540333,-5.77392186465499,
-5.70696579358409,-5.69491545313696,-5.6872895397492,-5.67852107487172,
-5.66054991806525,-5.63355162912398,-5.55971108181309,-5.54086217272583,
-5.52967993174404),.UNSPECIFIED.);
#1372=B_SPLINE_CURVE_WITH_KNOTS('',3,(#14652,#14653,#14654,#14655,#14656,
#14657,#14658,#14659,#14660,#14661,#14662,#14663,#14664,#14665,#14666,#14667,
#14668,#14669,#14670,#14671,#14672,#14673,#14674,#14675,#14676,#14677,#14678,
#14679,#14680,#14681,#14682,#14683,#14684,#14685,#14686,#14687,#14688,#14689,
#14690,#14691,#14692,#14693,#14694,#14695,#14696,#14697,#14698,#14699,#14700,
#14701,#14702,#14703,#14704,#14705,#14706,#14707,#14708,#14709,#14710,#14711,
#14712,#14713,#14714,#14715,#14716,#14717,#14718,#14719,#14720,#14721,#14722,
#14723,#14724,#14725,#14726,#14727,#14728,#14729,#14730,#14731,#14732,#14733,
#14734,#14735,#14736,#14737,#14738,#14739,#14740,#14741,#14742,#14743,#14744,
#14745,#14746,#14747,#14748,#14749,#14750,#14751,#14752,#14753,#14754,#14755,
#14756,#14757,#14758,#14759,#14760,#14761,#14762,#14763,#14764,#14765,#14766,
#14767,#14768,#14769,#14770,#14771,#14772,#14773,#14774,#14775,#14776,#14777,
#14778,#14779,#14780,#14781,#14782,#14783,#14784,#14785,#14786,#14787,#14788,
#14789,#14790,#14791,#14792,#14793,#14794,#14795,#14796,#14797,#14798,#14799,
#14800,#14801,#14802,#14803,#14804,#14805,#14806,#14807,#14808,#14809,#14810,
#14811,#14812,#14813),.UNSPECIFIED.,.F.,.F.,(4,2,2,2,2,2,2,2,2,2,2,2,2,
2,2,2,2,2,2,2,2,2,2,2,2,2,2,2,2,2,2,2,2,2,2,2,2,2,2,2,2,2,2,2,2,2,2,2,2,
2,2,2,2,2,2,2,2,2,2,2,2,2,2,2,2,2,2,2,2,2,2,2,2,2,2,2,2,2,2,2,4),(-7.86715098468372,
-7.83898087228045,-7.78036523028166,-7.76270811402096,-7.74945801760986,
-7.73451003250844,-7.7061622897504,-7.64100143095205,-7.61912747923954,
-7.60348526415976,-7.59513008643648,-7.58719446284538,-7.57377389478597,
-7.51234747555771,-7.47797998449431,-7.4526860930357,-7.43822860083035,
-7.42483604689371,-7.40603626000087,-7.36071512949483,-7.29978382107827,
-7.28510076359162,-7.27692569673354,-7.26984209924926,-7.2568708750197,
-7.19491378304418,-7.16037375065132,-7.13500034646873,-7.12052928309533,
-7.10714133050446,-7.08837750399718,-7.04386731040103,-7.00388678657383,
-6.98293054409437,-6.96773827864045,-6.95946673348263,-6.95243882343748,
-6.9398165490823,-6.89749006702733,-6.85051556770418,-6.82021906099846,
-6.80497809979182,-6.79177436055578,-6.77491441228576,-6.72682997282342,
-6.67918554233254,-6.65438631699614,-6.6446382969746,-6.63711738248382,
-6.62668834169425,-6.59644170944388,-6.55112836224944,-6.52111333499541,
-6.49792262259055,-6.48381859038211,-6.47024644290493,-6.45025022617551,
-6.4261373973076,-6.36381443577044,-6.33761401890689,-6.32758562157956,
-6.32007181758678,-6.31013226586847,-6.28366294746204,-6.22878505339136,
-6.18938319510126,-6.17262445838086,-6.15944773303133,-6.14393734139516,
-6.11173200926431,-6.05867046731735,-6.02164794627707,-6.0107399037768,
-6.00318471861087,-5.99378865514142,-5.97171585586828,-5.93362935164501,
-5.87755110729914,-5.85838589921919,-5.84494036718781,-5.83652165962026),
 .UNSPECIFIED.);
#1373=B_SPLINE_CURVE_WITH_KNOTS('',3,(#14818,#14819,#14820,#14821,#14822,
#14823,#14824,#14825,#14826,#14827,#14828,#14829,#14830,#14831,#14832,#14833,
#14834,#14835,#14836,#14837,#14838,#14839,#14840,#14841,#14842,#14843,#14844,
#14845,#14846,#14847,#14848,#14849,#14850,#14851,#14852,#14853,#14854,#14855,
#14856,#14857,#14858,#14859,#14860,#14861,#14862,#14863,#14864,#14865,#14866,
#14867,#14868,#14869,#14870,#14871,#14872,#14873,#14874,#14875,#14876,#14877,
#14878,#14879,#14880,#14881,#14882,#14883,#14884,#14885,#14886,#14887,#14888,
#14889,#14890,#14891,#14892,#14893,#14894,#14895,#14896,#14897,#14898,#14899,
#14900,#14901,#14902,#14903,#14904,#14905,#14906,#14907,#14908,#14909,#14910,
#14911,#14912,#14913,#14914,#14915,#14916,#14917,#14918,#14919,#14920,#14921,
#14922,#14923,#14924,#14925,#14926,#14927,#14928,#14929,#14930,#14931,#14932,
#14933,#14934,#14935,#14936,#14937,#14938,#14939,#14940,#14941,#14942,#14943,
#14944,#14945,#14946,#14947,#14948,#14949,#14950,#14951,#14952,#14953,#14954,
#14955,#14956,#14957,#14958,#14959,#14960,#14961,#14962,#14963,#14964,#14965,
#14966,#14967,#14968,#14969,#14970,#14971,#14972,#14973,#14974,#14975,#14976,
#14977),.UNSPECIFIED.,.F.,.F.,(4,2,2,2,2,2,2,2,2,2,2,2,2,2,2,2,2,2,2,2,
2,2,2,2,2,2,2,2,2,2,2,2,2,2,2,2,2,2,2,2,2,2,2,2,2,2,2,2,2,2,2,2,2,2,2,2,
2,2,2,2,2,2,2,2,2,2,2,2,2,2,2,2,2,2,2,2,2,2,2,4),(-9.59119486853264,-9.58541564180725,
-9.52523893204322,-9.51025654432291,-9.5020268834422,-9.49498036148374,
-9.4822289724785,-9.42003528946424,-9.38542265606388,-9.36001906526512,
-9.34554610572673,-9.33216453009469,-9.31342338369265,-9.23896129598912,
-9.2121968184616,-9.19432872957706,-9.18558001225223,-9.17795125516359,
-9.16586597797127,-9.10284839040491,-9.06796227981513,-9.04243355334127,
-9.02793938930535,-9.01456504120352,-8.99588000116821,-8.93066991415714,
-8.897985785038,-8.87776988980236,-8.86864464204234,-8.86104243199963,-8.84968637140788,
-8.78669234038215,-8.75093656094561,-8.72501619065484,-8.71045688641074,
-8.69710474869477,-8.67858913676088,-8.61176188924848,-8.57986951364058,
-8.55994698529019,-8.55086613385593,-8.54325261244276,-8.53181028274389,
-8.46958134221792,-8.43348518380628,-8.4074131814244,-8.3928281755799,-8.37948315628326,
-8.36102841711493,-8.29364283440822,-8.26201257185328,-8.24218805362476,
-8.23312181778317,-8.22550390479095,-8.2140309399148,-8.15206774802931,
-8.11584972015261,-8.0897233252304,-8.0751287711885,-8.06178576659132,-8.04335166011119,
-7.96697159462565,-7.94089749951307,-7.92332524642048,-7.91462549803555,
-7.90697438989995,-7.89475533014395,-7.83996309845466,-7.78132113063378,
-7.76366158402324,-7.75040976924443,-7.73545995014024,-7.70710911882736,
-7.6419389417069,-7.62006223008889,-7.60441803022939,-7.59606178413817,
-7.5881251385117,-7.57470283031182,-7.56063401821517),.UNSPECIFIED.);
#1374=B_SPLINE_CURVE_WITH_KNOTS('',3,(#14978,#14979,#14980,#14981,#14982,
#14983,#14984,#14985,#14986,#14987,#14988,#14989,#14990,#14991,#14992,#14993,
#14994,#14995,#14996,#14997,#14998,#14999,#15000,#15001,#15002,#15003,#15004,
#15005,#15006,#15007,#15008,#15009,#15010,#15011,#15012,#15013,#15014,#15015,
#15016,#15017,#15018,#15019,#15020,#15021,#15022,#15023,#15024,#15025,#15026,
#15027,#15028,#15029,#15030,#15031,#15032,#15033,#15034,#15035,#15036,#15037,
#15038,#15039,#15040,#15041,#15042,#15043,#15044,#15045,#15046,#15047,#15048,
#15049,#15050,#15051,#15052,#15053,#15054,#15055,#15056,#15057,#15058,#15059,
#15060,#15061,#15062,#15063,#15064,#15065,#15066,#15067,#15068,#15069,#15070,
#15071,#15072,#15073,#15074,#15075,#15076,#15077,#15078,#15079,#15080,#15081,
#15082,#15083,#15084,#15085,#15086,#15087,#15088,#15089,#15090,#15091,#15092,
#15093,#15094,#15095,#15096,#15097,#15098,#15099,#15100,#15101,#15102,#15103,
#15104,#15105,#15106,#15107,#15108,#15109,#15110,#15111,#15112,#15113,#15114,
#15115,#15116,#15117,#15118,#15119,#15120,#15121,#15122,#15123,#15124,#15125,
#15126,#15127,#15128,#15129,#15130,#15131,#15132,#15133),.UNSPECIFIED.,
 .F.,.F.,(4,2,2,2,2,2,2,2,2,2,2,2,2,2,2,2,2,2,2,2,2,2,2,2,2,2,2,2,2,2,2,
2,2,2,2,2,2,2,2,2,2,2,2,2,2,2,2,2,2,2,2,2,2,2,2,2,2,2,2,2,2,2,2,2,2,2,2,
2,2,2,2,2,2,2,2,2,2,4),(-5.83652165962026,-5.83060343340443,-5.8060372413055,
-5.77322406706544,-5.70627658063711,-5.69422778881706,-5.68660285467254,
-5.6778355148271,-5.65986666135426,-5.63287182961994,-5.55904078349039,
-5.54019429035759,-5.52679487644636,-5.51235295912005,-5.48715645013475,
-5.45299942006476,-5.38959117828366,-5.37698460102786,-5.36995907990201,
-5.36168254220858,-5.34646471494091,-5.32545895718013,-5.28559098159306,
-5.24111945894058,-5.222360786364,-5.2089733400481,-5.19449983792018,-5.16911473199233,
-5.13454814136845,-5.07253854000887,-5.05957963095843,-5.052497832828,-5.04431885043112,
-5.0296171566623,-5.00963890823567,-4.94127780057389,-4.91278363515482,
-4.89781227043409,-4.88456496582494,-4.86694723725331,-4.80768516548306,
-4.75340874619768,-4.74115445050499,-4.73349783007157,-4.72481128240199,
-4.70731604880015,-4.68141997733795,-4.60462511885929,-4.58626917723554,
-4.57293625961703,-4.55830990177338,-4.53199081093302,-4.49533213249982,
-4.43428099082099,-4.42270076548914,-4.41506872556729,-4.40605598142384,
-4.38657495756673,-4.3558452426953,-4.28657456568634,-4.26835071020849,
-4.25503506367867,-4.24035457830638,-4.21369863751306,-4.17625873129053,
-4.11695049216103,-4.10517752401883,-4.0975189451925,-4.08859798365488,
-4.0696917481748,-4.04042240445074,-3.96779854382722,-3.95000734383667,
-3.93674340072654,-3.92186493432069,-3.89396043893714,-3.85349346320142,
-3.8056948071301),.UNSPECIFIED.);
#1375=B_SPLINE_CURVE_WITH_KNOTS('',3,(#15138,#15139,#15140,#15141,#15142,
#15143,#15144,#15145,#15146,#15147,#15148,#15149,#15150,#15151,#15152,#15153,
#15154,#15155,#15156,#15157,#15158,#15159,#15160,#15161,#15162,#15163,#15164,
#15165,#15166,#15167,#15168,#15169,#15170,#15171,#15172,#15173,#15174,#15175,
#15176,#15177,#15178,#15179,#15180,#15181,#15182,#15183,#15184,#15185,#15186,
#15187,#15188,#15189,#15190,#15191,#15192,#15193,#15194,#15195,#15196,#15197,
#15198,#15199,#15200,#15201,#15202,#15203,#15204,#15205,#15206,#15207,#15208,
#15209,#15210,#15211,#15212,#15213,#15214,#15215,#15216,#15217,#15218,#15219,
#15220,#15221,#15222,#15223,#15224,#15225,#15226,#15227,#15228,#15229,#15230,
#15231,#15232,#15233,#15234,#15235,#15236,#15237,#15238,#15239,#15240,#15241,
#15242,#15243,#15244,#15245,#15246,#15247,#15248,#15249,#15250,#15251,#15252,
#15253,#15254,#15255,#15256,#15257,#15258,#15259,#15260,#15261,#15262,#15263,
#15264,#15265,#15266,#15267,#15268,#15269,#15270,#15271,#15272,#15273,#15274,
#15275,#15276,#15277,#15278,#15279,#15280,#15281,#15282,#15283,#15284,#15285,
#15286,#15287,#15288,#15289,#15290,#15291,#15292,#15293,#15294,#15295,#15296,
#15297),.UNSPECIFIED.,.F.,.F.,(4,2,2,2,2,2,2,2,2,2,2,2,2,2,2,2,2,2,2,2,
2,2,2,2,2,2,2,2,2,2,2,2,2,2,2,2,2,2,2,2,2,2,2,2,2,2,2,2,2,2,2,2,2,2,2,2,
2,2,2,2,2,2,2,2,2,2,2,2,2,2,2,2,2,2,2,2,2,2,2,4),(-11.6209589861144,-11.6133663359858,
-11.5852202047392,-11.5703672184993,-11.5572093879312,-11.5400129782168,
-11.464398022885,-11.4361708524617,-11.4177042261508,-11.4088922037687,
-11.4013266147797,-11.3895760285217,-11.3301634015277,-11.2927997434517,
-11.2661659157797,-11.2514752888791,-11.2381345274991,-11.219841790701,
-11.1430208500536,-11.1172871252356,-11.0998648553724,-11.0911784686328,
-11.0835012274409,-11.0711532604214,-11.0062095874946,-10.972740506592,
-10.9478705224309,-10.9334867383894,-10.9200686462429,-10.9040990587281,
-10.823947907962,-10.7990659565336,-10.7820221778567,-10.7734176075462,
-10.7657368334286,-10.7532945913264,-10.6889548590096,-10.6552225995426,
-10.6302305583084,-10.6158350801731,-10.6024410804383,-10.5835395256831,
-10.5100727904326,-10.4829237501559,-10.4648948869758,-10.456124201246,
-10.4485096159138,-10.4365045995646,-10.3794275399521,-10.3220511806881,
-10.3046514616701,-10.291427296354,-10.2763383060808,-10.2470588104962,
-10.1797595888859,-10.1598889683449,-10.1452444038481,-10.1370765514168,
-10.1299892092107,-10.1169877524896,-10.0550984426467,-10.0205884526424,
-9.9952329698693,-9.9807689227846,-9.96738569180286,-9.94862557158994,-9.90407365533332,
-9.86387149170127,-9.84308018808439,-9.82797182578637,-9.81971851594382,
-9.8126863720025,-9.80002170106756,-9.73711779038159,-9.70281440939386,
-9.67755370248871,-9.66310615132511,-9.64971811400841,-9.63091686560303,
-9.59119486853264),.UNSPECIFIED.);
#1376=B_SPLINE_CURVE_WITH_KNOTS('',3,(#15298,#15299,#15300,#15301,#15302,
#15303,#15304,#15305,#15306,#15307,#15308,#15309,#15310,#15311,#15312,#15313,
#15314,#15315,#15316,#15317,#15318,#15319,#15320,#15321,#15322,#15323,#15324,
#15325,#15326,#15327,#15328,#15329,#15330,#15331,#15332,#15333,#15334,#15335,
#15336,#15337,#15338,#15339,#15340,#15341,#15342,#15343,#15344,#15345,#15346,
#15347,#15348,#15349,#15350,#15351,#15352,#15353,#15354,#15355,#15356,#15357,
#15358,#15359,#15360,#15361,#15362,#15363,#15364,#15365,#15366,#15367,#15368,
#15369,#15370,#15371,#15372,#15373,#15374,#15375,#15376,#15377,#15378,#15379,
#15380,#15381,#15382,#15383,#15384,#15385,#15386,#15387,#15388,#15389,#15390,
#15391,#15392,#15393,#15394,#15395,#15396,#15397,#15398,#15399,#15400,#15401,
#15402,#15403,#15404,#15405,#15406,#15407,#15408,#15409,#15410,#15411,#15412,
#15413,#15414,#15415,#15416,#15417,#15418,#15419,#15420,#15421,#15422,#15423,
#15424,#15425,#15426,#15427,#15428,#15429,#15430,#15431,#15432,#15433,#15434,
#15435,#15436,#15437,#15438,#15439,#15440,#15441,#15442,#15443,#15444,#15445,
#15446,#15447,#15448,#15449,#15450,#15451,#15452,#15453,#15454,#15455),
 .UNSPECIFIED.,.F.,.F.,(4,2,2,2,2,2,2,2,2,2,2,2,2,2,2,2,2,2,2,2,2,2,2,2,
2,2,2,2,2,2,2,2,2,2,2,2,2,2,2,2,2,2,2,2,2,2,2,2,2,2,2,2,2,2,2,2,2,2,2,2,
2,2,2,2,2,2,2,2,2,2,2,2,2,2,2,2,2,2,4),(-3.8056948071301,-3.80026512065085,
-3.78798078993115,-3.78032053900756,-3.77164794451955,-3.75422693301958,
-3.72849750768735,-3.65127124070465,-3.6329928362497,-3.6196721167688,-3.60501834921775,
-3.57851720427146,-3.5414337801098,-3.48135807784409,-3.46967337759391,
-3.46202830157603,-3.4530690061614,-3.43391762282551,-3.40402884300443,
-3.33287805624423,-3.31489714895829,-3.30161332184237,-3.28682956744793,
-3.25951532681412,-3.22050188869135,-3.16459009453224,-3.15246220625848,
-3.14482720911384,-3.13609588845081,-3.11832893183051,-3.09180103978626,
-3.0167851423361,-2.9981465663304,-2.98477948336773,-2.97026967862569,-2.94464264621276,
-2.90953613609495,-2.84588683766129,-2.83427738927482,-2.82664347352911,
-2.81765054826228,-2.79828026756363,-2.76782943230424,-2.69797861537475,
-2.6798361108054,-2.66653513878977,-2.65182902775769,-2.62498780633035,
-2.58710332986536,-2.52881489031045,-2.51693541097618,-2.50933909085913,
-2.50050925903385,-2.4821469123443,-2.45420680869822,-2.37835411535174,
-2.36119191747364,-2.34796592085046,-2.33292479198953,-2.30393982971893,
-2.26064819060926,-2.21286864464054,-2.20013602211377,-2.19309246466381,
-2.1848533004922,-2.16983066704586,-2.09396879350949,-2.05799234407928,
-2.04167922521324,-2.02852484453212,-2.01265975205705,-1.97766511097321,
-1.91336405211699,-1.8890958007975,-1.87935274463646,-1.87184594941125,
-1.86162981250708,-1.83234117395985,-1.77559603949032),.UNSPECIFIED.);
#1377=B_SPLINE_CURVE_WITH_KNOTS('',3,(#15459,#15460,#15461,#15462,#15463,
#15464),.UNSPECIFIED.,.F.,.F.,(4,1,1,4),(-4.09274904019425,-3.93242675008978,
-2.94932006256733,-2.06169017104378),.UNSPECIFIED.);
#1378=B_SPLINE_CURVE_WITH_KNOTS('',3,(#15468,#15469,#15470,#15471,#15472),
 .UNSPECIFIED.,.F.,.F.,(4,1,4),(0.,0.983106687522444,1.11004521091135),
 .UNSPECIFIED.);
#1379=B_SPLINE_CURVE_WITH_KNOTS('',3,(#15474,#15475,#15476,#15477,#15478,
#15479,#15480,#15481,#15482,#15483,#15484,#15485,#15486,#15487,#15488,#15489,
#15490,#15491,#15492,#15493,#15494,#15495,#15496,#15497,#15498,#15499,#15500,
#15501,#15502,#15503,#15504,#15505,#15506,#15507,#15508,#15509,#15510,#15511,
#15512,#15513,#15514,#15515,#15516,#15517,#15518,#15519,#15520,#15521,#15522,
#15523,#15524,#15525,#15526,#15527,#15528,#15529,#15530,#15531,#15532,#15533,
#15534,#15535,#15536,#15537,#15538,#15539,#15540,#15541,#15542,#15543,#15544,
#15545,#15546,#15547,#15548,#15549,#15550,#15551,#15552,#15553,#15554,#15555,
#15556,#15557,#15558,#15559,#15560,#15561,#15562,#15563,#15564,#15565,#15566,
#15567,#15568,#15569,#15570,#15571,#15572,#15573,#15574,#15575,#15576,#15577,
#15578,#15579,#15580,#15581,#15582,#15583,#15584,#15585,#15586,#15587,#15588,
#15589,#15590,#15591,#15592,#15593,#15594,#15595,#15596,#15597,#15598,#15599,
#15600,#15601,#15602,#15603,#15604,#15605,#15606,#15607,#15608,#15609,#15610,
#15611,#15612,#15613,#15614,#15615,#15616,#15617,#15618,#15619,#15620,#15621,
#15622,#15623,#15624,#15625,#15626,#15627,#15628,#15629,#15630,#15631,#15632,
#15633,#15634,#15635,#15636,#15637,#15638,#15639,#15640,#15641,#15642,#15643,
#15644,#15645,#15646,#15647,#15648,#15649,#15650,#15651,#15652,#15653,#15654,
#15655,#15656,#15657,#15658,#15659,#15660,#15661,#15662,#15663,#15664,#15665,
#15666,#15667,#15668,#15669,#15670,#15671,#15672,#15673,#15674,#15675,#15676,
#15677,#15678,#15679,#15680,#15681,#15682,#15683,#15684,#15685,#15686,#15687),
 .UNSPECIFIED.,.F.,.F.,(4,3,3,3,3,3,3,3,3,3,3,3,3,3,3,3,3,3,3,3,3,3,3,3,
3,3,3,3,3,3,3,3,3,3,3,3,3,3,3,3,3,3,3,3,3,3,3,3,3,3,3,3,3,3,3,3,3,3,3,3,
3,3,3,3,3,3,3,3,3,3,3,4),(1.11004521091135,1.19678975220784,1.28343491823949,
1.37000463720176,1.45653382267758,1.5430452412911,1.62956163882972,1.71615883137897,
1.80279632295003,1.88957177193842,1.96621337504489,2.05504161319154,2.14375845460894,
2.23238732145028,2.32200391408991,2.41053563202563,2.49905481643986,2.58758250555964,
2.67801689481156,2.76667099136226,2.8579955269648,2.94932006256733,3.0381928086099,
3.12695687505772,3.21563561039046,3.30523450285287,3.39382229827685,3.48239979811089,
3.57098798371731,3.66134767531043,3.75006715623379,3.84124695316178,3.93242675008978,
4.02106908933155,4.10959899246734,4.19804013238219,4.28772679553595,4.37607010743289,
4.46440098087566,4.55274067520436,4.64343886580633,4.73190750732771,4.82372047246997,
4.91553343761222,5.00429084893833,5.09293715563453,5.18149587482453,5.2711389061133,
5.35960192849135,5.44805309718548,5.5365135366545,5.62704518377454,5.71563458423383,
5.80713735468425,5.89864012513467,5.9873917216973,6.07603240737187,6.16458570587497,
6.25423084422274,6.34268897955531,6.43113547147725,6.51959145102956,6.61013029143644,
6.69871581619304,6.79023131442508,6.88174681265711,6.97411288160619,7.06632853394111,
7.15835923647718,7.25027958940315,7.3420698192528,7.39323051809094),
 .UNSPECIFIED.);
#1380=B_SPLINE_CURVE_WITH_KNOTS('',3,(#15689,#15690,#15691,#15692,#15693,
#15694,#15695,#15696,#15697,#15698,#15699,#15700,#15701,#15702,#15703,#15704,
#15705,#15706,#15707,#15708,#15709,#15710,#15711,#15712,#15713,#15714,#15715,
#15716,#15717,#15718,#15719,#15720,#15721,#15722,#15723,#15724,#15725,#15726,
#15727,#15728,#15729,#15730,#15731,#15732,#15733,#15734,#15735,#15736,#15737,
#15738,#15739,#15740,#15741,#15742,#15743,#15744,#15745,#15746,#15747,#15748,
#15749,#15750,#15751,#15752,#15753,#15754,#15755,#15756,#15757,#15758,#15759,
#15760,#15761,#15762,#15763,#15764,#15765,#15766,#15767,#15768,#15769,#15770,
#15771,#15772,#15773,#15774,#15775,#15776,#15777,#15778,#15779,#15780,#15781,
#15782,#15783,#15784,#15785,#15786,#15787,#15788,#15789,#15790,#15791,#15792,
#15793,#15794,#15795,#15796,#15797,#15798,#15799,#15800,#15801,#15802,#15803,
#15804,#15805,#15806,#15807,#15808,#15809,#15810,#15811,#15812,#15813,#15814,
#15815,#15816,#15817,#15818,#15819,#15820,#15821,#15822,#15823,#15824,#15825,
#15826,#15827,#15828,#15829,#15830,#15831,#15832,#15833,#15834,#15835,#15836,
#15837,#15838,#15839,#15840,#15841,#15842,#15843,#15844,#15845,#15846,#15847,
#15848,#15849,#15850,#15851,#15852,#15853,#15854,#15855,#15856,#15857,#15858,
#15859,#15860,#15861,#15862,#15863,#15864,#15865,#15866,#15867,#15868,#15869,
#15870,#15871,#15872,#15873,#15874,#15875,#15876,#15877,#15878,#15879,#15880,
#15881,#15882,#15883,#15884,#15885,#15886,#15887,#15888,#15889,#15890,#15891,
#15892,#15893,#15894,#15895,#15896,#15897,#15898,#15899,#15900,#15901,#15902),
 .UNSPECIFIED.,.F.,.F.,(4,3,3,3,3,3,3,3,3,3,3,3,3,3,3,3,3,3,3,3,3,3,3,3,
3,3,3,3,3,3,3,3,3,3,3,3,3,3,3,3,3,3,3,3,3,3,3,3,3,3,3,3,3,3,3,3,3,3,3,3,
3,3,3,3,3,3,3,3,3,3,3,4),(7.39323051828195,7.48652054956581,7.58110378721925,
7.67478982599243,7.76982166308599,7.86485350017956,7.95359508066845,8.04222550164844,
8.13076830134049,8.22041728713568,8.30886441436785,8.39729972657984,8.48574436695792,
8.57629832214394,8.66487221403951,8.75641620087076,8.84796018770201,8.9366994182996,
9.02532749057653,9.11386794582422,9.20351781199924,9.29196262122918,9.38039562969083,
9.46883798332746,9.55939520630171,9.64796687526505,9.73951687524475,9.83106687522445,
9.91980333279088,10.0084285796802,10.0969661610973,10.1866170863035,10.2750589210137,
10.3634889224932,10.4519282400123,10.5424895706959,10.6310581587922,10.7226158607695,
10.8141735627469,10.9029121693186,10.9915395941898,11.0800793795962,11.1697294884303,
11.2581735767141,11.3466058462972,11.4350474438882,11.5256056454835,11.6141765224489,
11.7057283863591,11.7972802502693,11.8860183603648,11.974645285871,12.0631845696889,
12.1528348657018,12.241278450278,12.329710216285,12.418151311018,12.5087102177114,
12.5972805982841,12.688833768038,12.7803869377918,12.8681225266378,12.9557475363413,
13.0458310724326,13.1333091513524,13.22075795565,13.3081996293495,13.4002536782799,
13.4877923470092,13.5753806118336,13.6630807303213,13.6764158250714),
 .UNSPECIFIED.);
#1381=B_SPLINE_CURVE_WITH_KNOTS('',3,(#15904,#15905,#15906,#15907,#15908,
#15909,#15910,#15911,#15912,#15913,#15914,#15915,#15916,#15917,#15918,#15919,
#15920,#15921,#15922,#15923,#15924,#15925,#15926,#15927,#15928,#15929,#15930,
#15931,#15932,#15933,#15934,#15935,#15936,#15937,#15938,#15939,#15940,#15941,
#15942,#15943,#15944,#15945,#15946,#15947,#15948,#15949,#15950,#15951,#15952,
#15953,#15954,#15955,#15956,#15957,#15958,#15959,#15960,#15961,#15962,#15963,
#15964,#15965,#15966,#15967,#15968,#15969,#15970,#15971,#15972,#15973,#15974,
#15975,#15976,#15977,#15978,#15979,#15980,#15981,#15982,#15983,#15984,#15985,
#15986,#15987,#15988,#15989,#15990,#15991,#15992,#15993,#15994,#15995,#15996,
#15997,#15998,#15999,#16000,#16001,#16002,#16003,#16004,#16005,#16006,#16007,
#16008,#16009,#16010,#16011,#16012,#16013,#16014,#16015,#16016,#16017,#16018,
#16019,#16020,#16021,#16022,#16023,#16024,#16025,#16026,#16027,#16028,#16029,
#16030,#16031,#16032,#16033,#16034,#16035,#16036,#16037,#16038,#16039,#16040,
#16041,#16042,#16043,#16044,#16045,#16046,#16047,#16048,#16049,#16050,#16051,
#16052,#16053,#16054,#16055,#16056,#16057,#16058,#16059,#16060,#16061,#16062,
#16063,#16064,#16065,#16066,#16067,#16068,#16069,#16070,#16071,#16072,#16073,
#16074,#16075,#16076,#16077,#16078,#16079,#16080,#16081,#16082,#16083,#16084,
#16085,#16086,#16087,#16088,#16089,#16090,#16091,#16092,#16093,#16094,#16095,
#16096,#16097,#16098,#16099,#16100,#16101,#16102,#16103,#16104,#16105,#16106,
#16107,#16108,#16109,#16110,#16111,#16112,#16113,#16114),.UNSPECIFIED.,
 .F.,.F.,(4,3,3,3,3,3,3,3,3,3,3,3,3,3,3,3,3,3,3,3,3,3,3,3,3,3,3,3,3,3,3,
3,3,3,3,3,3,3,3,3,3,3,3,3,3,3,3,3,3,3,3,3,3,3,3,3,3,3,3,3,3,3,3,3,3,3,3,
3,3,3,4),(13.6764158252705,13.7634936253142,13.8522317431468,13.9408586745873,
14.0293979625368,14.1190482563242,14.2074918405328,14.2959236044768,14.3843646954449,
14.4749235997929,14.5634939723758,14.6550471426062,14.7466003128367,14.8353383442683,
14.9239651885601,15.01250438873,15.1021547151836,15.190598210643,15.2790298856361,
15.3674708875542,15.4580299157554,15.5466001998664,15.6381536001127,15.7297070003591,
15.8184450096981,15.9070718313089,15.9956110082415,16.0852613431965,16.1737048141959,
16.2621364643134,16.350577440967,16.4411365026957,16.5297067608031,16.6212602243424,
16.7128136878816,16.801551731529,16.8901785879679,16.9787178002004,17.0683681221008,
17.1568116293316,17.2452433159646,17.3336843293769,17.4242433408836,17.5128136360172,
17.6043670057106,17.695920375404,17.7846584054267,17.8732852480993,17.9618244464429,
18.0514747735033,18.1399182666344,18.2283499391144,18.3167909383364,18.4073499694839,
18.495920250466,18.5874736566962,18.6790270629265,18.7677650921009,18.8563919338726,
18.944931131264,19.0345814586621,19.1230249507207,19.2114566220848,19.2998976201488,
19.3904566527238,19.4790269324526,19.5705803414507,19.6621337504489,19.7691043504165,
19.8748949960292,19.9596009710764),.UNSPECIFIED.);
#1382=B_SPLINE_CURVE_WITH_KNOTS('',3,(#16116,#16117,#16118,#16119,#16120,
#16121,#16122,#16123,#16124,#16125),.UNSPECIFIED.,.F.,.F.,(4,1,1,1,1,1,
1,4),(19.9596011324501,20.6452404379713,21.6283471254938,22.6114538130162,
23.5945605005387,24.5776671880611,25.5607738755836,26.2427864396297),
 .UNSPECIFIED.);
#1383=B_SPLINE_CURVE_WITH_KNOTS('',3,(#16127,#16128,#16129,#16130,#16131,
#16132,#16133,#16134,#16135,#16136,#16137,#16138,#16139,#16140,#16141,#16142,
#16143,#16144,#16145,#16146,#16147,#16148,#16149,#16150,#16151,#16152,#16153,
#16154,#16155,#16156,#16157,#16158,#16159,#16160,#16161,#16162,#16163,#16164,
#16165,#16166,#16167,#16168,#16169,#16170,#16171,#16172,#16173,#16174,#16175,
#16176,#16177,#16178,#16179,#16180,#16181,#16182,#16183,#16184,#16185,#16186,
#16187,#16188,#16189,#16190,#16191,#16192,#16193,#16194,#16195,#16196,#16197,
#16198,#16199,#16200,#16201,#16202,#16203,#16204,#16205,#16206,#16207,#16208,
#16209,#16210,#16211,#16212,#16213,#16214,#16215,#16216,#16217,#16218,#16219,
#16220,#16221,#16222,#16223,#16224,#16225,#16226,#16227,#16228,#16229,#16230,
#16231,#16232,#16233,#16234,#16235,#16236,#16237,#16238,#16239,#16240,#16241,
#16242,#16243,#16244,#16245,#16246,#16247,#16248,#16249,#16250,#16251,#16252,
#16253,#16254,#16255,#16256,#16257,#16258,#16259,#16260,#16261,#16262,#16263,
#16264,#16265,#16266,#16267,#16268,#16269,#16270,#16271,#16272,#16273,#16274,
#16275,#16276,#16277,#16278,#16279,#16280,#16281,#16282,#16283,#16284,#16285,
#16286,#16287,#16288,#16289,#16290,#16291,#16292,#16293,#16294,#16295,#16296,
#16297,#16298,#16299,#16300,#16301,#16302,#16303,#16304,#16305,#16306,#16307,
#16308,#16309,#16310,#16311,#16312,#16313,#16314,#16315,#16316,#16317,#16318,
#16319,#16320,#16321,#16322,#16323,#16324,#16325,#16326,#16327,#16328,#16329,
#16330,#16331,#16332,#16333,#16334,#16335,#16336,#16337),.UNSPECIFIED.,
 .F.,.F.,(4,3,3,3,3,3,3,3,3,3,3,3,3,3,3,3,3,3,3,3,3,3,3,3,3,3,3,3,3,3,3,
3,3,3,3,3,3,3,3,3,3,3,3,3,3,3,3,3,3,3,3,3,3,3,3,3,3,3,3,3,3,3,3,3,3,3,3,
3,3,3,4),(26.2427866070854,26.3479545531162,26.4543084236402,26.543880563106,
26.6326185967606,26.7212454428436,26.8097846443747,26.8994349701564,26.9878784659124,
27.0763101408029,27.1647511422193,27.2553101693216,27.3438804519463,27.4354338512874,
27.5269872506285,27.6157253715144,27.7043523054151,27.7928915952337,27.8825418880984,
27.9709854727142,28.059417236517,28.147858326796,28.2384172296347,28.3269876001762,
28.4185407691635,28.5100939381509,28.5988317636565,28.6874584018148,28.7759973958981,
28.86564779962,28.9540910904238,29.0425225616604,29.1309633609485,29.2215226771297,
29.3100927632426,29.4016466944579,29.4932006256733,29.5819387577266,29.6705657009244,
29.759104998185,29.8487552875613,29.9371988750663,30.0256306400592,30.1140717298361,
30.204630625676,30.2932009915689,30.3847541523824,30.4763073131958,30.5650459322033,
30.6536733670943,30.742213160114,30.8318632651896,30.920307355132,31.0087396241407,
31.0971812189247,31.187739414373,31.2763102830244,31.3678621418713,31.4594140007182,
31.5481503446818,31.6367755000393,31.7253130119065,31.8149639714483,31.9034057910051,
31.9918357977297,32.0802751408886,32.1708365277266,32.2594051917707,32.3509629400057,
32.4425206882407,32.5259717468093),.UNSPECIFIED.);
#1384=B_SPLINE_CURVE_WITH_KNOTS('',3,(#16339,#16340,#16341,#16342,#16343,
#16344,#16345,#16346,#16347,#16348,#16349,#16350,#16351,#16352,#16353,#16354,
#16355,#16356,#16357,#16358,#16359,#16360,#16361,#16362,#16363,#16364,#16365,
#16366,#16367,#16368,#16369,#16370,#16371,#16372,#16373,#16374,#16375,#16376,
#16377,#16378,#16379,#16380,#16381,#16382,#16383,#16384,#16385,#16386,#16387,
#16388,#16389,#16390,#16391,#16392,#16393,#16394,#16395,#16396,#16397,#16398,
#16399,#16400,#16401,#16402,#16403,#16404,#16405,#16406,#16407,#16408,#16409,
#16410,#16411,#16412,#16413,#16414,#16415,#16416,#16417,#16418,#16419,#16420,
#16421,#16422,#16423,#16424,#16425,#16426,#16427,#16428,#16429,#16430,#16431,
#16432,#16433,#16434,#16435,#16436,#16437,#16438,#16439,#16440,#16441,#16442,
#16443,#16444,#16445,#16446,#16447,#16448,#16449,#16450,#16451,#16452,#16453,
#16454,#16455,#16456,#16457,#16458,#16459,#16460,#16461,#16462,#16463,#16464,
#16465,#16466,#16467,#16468,#16469,#16470,#16471,#16472,#16473,#16474,#16475,
#16476,#16477,#16478,#16479,#16480,#16481,#16482,#16483,#16484,#16485,#16486,
#16487,#16488,#16489,#16490,#16491,#16492,#16493,#16494,#16495,#16496,#16497,
#16498,#16499,#16500,#16501,#16502,#16503,#16504,#16505,#16506,#16507,#16508,
#16509,#16510,#16511,#16512,#16513,#16514,#16515,#16516,#16517,#16518,#16519,
#16520,#16521,#16522,#16523,#16524,#16525,#16526,#16527,#16528,#16529,#16530,
#16531,#16532,#16533,#16534,#16535,#16536,#16537,#16538,#16539,#16540,#16541,
#16542,#16543,#16544,#16545,#16546,#16547,#16548,#16549,#16550,#16551,#16552),
 .UNSPECIFIED.,.F.,.F.,(4,3,3,3,3,3,3,3,3,3,3,3,3,3,3,3,3,3,3,3,3,3,3,3,
3,3,3,3,3,3,3,3,3,3,3,3,3,3,3,3,3,3,3,3,3,3,3,3,3,3,3,3,3,3,3,3,3,3,3,3,
3,3,3,3,3,3,3,3,3,3,3,4),(32.5259717470035,32.6136980930916,32.701321678818,
32.7918598909362,32.8793558979929,32.9668299162081,33.0543040619837,33.141800447384,
33.2293879776738,33.3170302208598,33.4047956094643,33.4256273757631,33.5143689611472,
33.6029993860714,33.6915421887604,33.781191173076,33.869638300961,33.9580736129468,
34.0465182522196,34.1370722049861,34.2256460936089,34.3171900784472,34.4087340632856,
34.4974587852672,34.5860723001678,34.6745981676636,34.7642534905566,34.8526837311237,
34.9411022040174,35.02953007149,35.1201077413195,35.2086651786023,35.3002529647052,
35.391840750808,35.4805940901191,35.5692361798978,35.6577905452261,35.7474351568642,
35.8358935245118,35.9243399357615,36.0127955217129,36.1033335008673,36.1919178603191,
36.2834326493248,36.3749474383305,36.4637041692099,36.5523499276875,36.640908230355,
36.7305514672923,36.819014398981,36.9074655991963,36.9959261923746,37.0864581757442,
37.1750480312141,37.2665510785335,37.3580541258529,37.4466911686978,37.5352168033682,
37.6236546985531,37.7133429629058,37.8016855655941,37.8900166797626,37.9783575645755,
38.0690583767754,38.1575305552665,38.2493456843209,38.3411608133753,38.4356542346234,
38.5298819648782,38.6239500559712,38.7177816411047,38.8091570537371),
 .UNSPECIFIED.);
#1385=B_SPLINE_CURVE_WITH_KNOTS('',3,(#16554,#16555,#16556,#16557,#16558,
#16559,#16560,#16561,#16562,#16563,#16564,#16565,#16566,#16567,#16568,#16569,
#16570,#16571,#16572,#16573,#16574,#16575,#16576,#16577,#16578,#16579,#16580,
#16581,#16582,#16583,#16584,#16585,#16586,#16587,#16588,#16589,#16590,#16591,
#16592,#16593,#16594,#16595,#16596,#16597,#16598,#16599,#16600,#16601,#16602),
 .UNSPECIFIED.,.F.,.F.,(4,3,3,3,3,3,3,3,3,3,3,3,3,3,3,3,4),(38.8091570539889,
38.9008783254566,38.9926880493904,39.0846744010417,39.1767552641066,39.2690206125089,
39.3242675008978,39.4119600362523,39.4995435474641,39.5886488497747,39.6760895585896,
39.7635022245041,39.8509090171825,39.9412782543742,40.0287830710683,40.1205845185088,
40.2123859659494),.UNSPECIFIED.);
#1386=B_SPLINE_CURVE_WITH_KNOTS('',3,(#16606,#16607,#16608,#16609),
 .UNSPECIFIED.,.F.,.F.,(4,4),(-42.2735875634651,-41.7918885049275),
 .UNSPECIFIED.);
#1387=B_SPLINE_CURVE_WITH_KNOTS('',3,(#16611,#16612,#16613,#16614,#16615,
#16616,#16617,#16618,#16619,#16620,#16621,#16622,#16623,#16624,#16625,#16626,
#16627,#16628,#16629,#16630,#16631,#16632,#16633,#16634,#16635,#16636,#16637,
#16638,#16639,#16640,#16641,#16642,#16643,#16644,#16645,#16646,#16647,#16648,
#16649,#16650,#16651,#16652,#16653,#16654,#16655,#16656,#16657,#16658,#16659,
#16660,#16661,#16662,#16663,#16664,#16665,#16666,#16667,#16668,#16669,#16670,
#16671,#16672,#16673,#16674,#16675,#16676,#16677,#16678,#16679,#16680,#16681,
#16682,#16683,#16684,#16685,#16686,#16687,#16688,#16689,#16690,#16691,#16692,
#16693,#16694,#16695,#16696,#16697,#16698,#16699,#16700,#16701,#16702,#16703,
#16704,#16705,#16706,#16707,#16708,#16709,#16710,#16711,#16712,#16713,#16714,
#16715,#16716,#16717,#16718,#16719,#16720,#16721,#16722,#16723,#16724,#16725,
#16726,#16727,#16728,#16729,#16730,#16731,#16732,#16733,#16734,#16735,#16736,
#16737,#16738,#16739,#16740,#16741,#16742,#16743,#16744,#16745,#16746,#16747,
#16748,#16749,#16750,#16751,#16752,#16753,#16754,#16755,#16756,#16757,#16758,
#16759,#16760,#16761,#16762,#16763,#16764,#16765,#16766,#16767,#16768,#16769,
#16770,#16771,#16772,#16773,#16774,#16775,#16776,#16777,#16778,#16779,#16780,
#16781,#16782,#16783,#16784,#16785,#16786,#16787,#16788,#16789,#16790,#16791,
#16792,#16793,#16794,#16795,#16796,#16797,#16798,#16799,#16800,#16801,#16802,
#16803,#16804,#16805,#16806,#16807,#16808,#16809,#16810,#16811,#16812,#16813,
#16814,#16815,#16816,#16817,#16818,#16819,#16820,#16821,#16822,#16823,#16824,
#16825,#16826,#16827),.UNSPECIFIED.,.F.,.F.,(4,3,3,3,3,3,3,3,3,3,3,3,3,
3,3,3,3,3,3,3,3,3,3,3,3,3,3,3,3,3,3,3,3,3,3,3,3,3,3,3,3,3,3,3,3,3,3,3,3,
3,3,3,3,3,3,3,3,3,3,3,3,3,3,3,3,3,3,3,3,3,3,3,4),(-41.7918608832718,-41.6963680489168,
-41.6006510282217,-41.5046149620455,-41.4084115456498,-41.3119771500066,
-41.2904808759427,-41.2025196790987,-41.1146804894366,-41.0269387856156,
-40.9369932109662,-40.8493667994677,-40.7617582010694,-40.6741454427343,
-40.5824526291558,-40.4947162756479,-40.406921130202,-40.3190026549469,
-40.3073741884202,-40.218546539833,-40.1298302953959,-40.041202032106,-39.951585215705,
-39.8630541133568,-39.7745355478778,-39.6860084803038,-39.5955732354523,
-39.5069197610933,-39.4155936309956,-39.3242675008978,-39.2353948206761,
-39.1466308219898,-39.0579521562669,-38.9683532384055,-38.8797655167199,
-38.7911880920509,-38.7025999829601,-38.6122401905639,-38.5235207888384,
-38.4323408011069,-38.3411608133753,-38.2525182595748,-38.1639881390155,
-38.075546779094,-37.9858601974389,-37.8975166605352,-37.8091855605984,
-37.7208456385293,-37.6301477603602,-37.5416788900287,-37.4498665079408,
-37.3580541258529,-37.2692968116588,-37.180650603046,-37.0920919827586,
-37.0024489147051,-36.9139859925937,-36.8255349244951,-36.7370745858353,
-36.6465427989591,-36.5579534989103,-36.4664504686204,-36.3749474383305,
-36.2873765264958,-36.1999158891338,-36.1125489134617,-36.0252336577821,
-35.9379478187613,-35.8506691225993,-35.7633296057599,-35.6759609642527,
-35.5884727859879,-35.5086755762926),.UNSPECIFIED.);
#1388=B_SPLINE_CURVE_WITH_KNOTS('',3,(#16829,#16830,#16831,#16832,#16833,
#16834,#16835,#16836,#16837,#16838,#16839,#16840,#16841,#16842,#16843,#16844,
#16845,#16846,#16847,#16848,#16849,#16850,#16851,#16852,#16853,#16854,#16855,
#16856,#16857,#16858,#16859,#16860,#16861,#16862,#16863,#16864,#16865,#16866,
#16867,#16868,#16869,#16870,#16871,#16872,#16873,#16874,#16875,#16876,#16877,
#16878,#16879,#16880,#16881,#16882,#16883,#16884,#16885,#16886,#16887,#16888,
#16889,#16890,#16891,#16892,#16893,#16894,#16895,#16896,#16897,#16898,#16899,
#16900,#16901,#16902,#16903,#16904,#16905,#16906,#16907,#16908,#16909,#16910,
#16911,#16912,#16913,#16914,#16915,#16916,#16917,#16918,#16919,#16920,#16921,
#16922,#16923,#16924,#16925,#16926,#16927,#16928,#16929,#16930,#16931,#16932,
#16933,#16934,#16935,#16936,#16937,#16938,#16939,#16940,#16941,#16942,#16943,
#16944,#16945,#16946,#16947,#16948,#16949,#16950,#16951,#16952,#16953,#16954,
#16955,#16956,#16957,#16958,#16959,#16960,#16961,#16962,#16963,#16964,#16965,
#16966,#16967,#16968,#16969,#16970,#16971,#16972,#16973,#16974,#16975,#16976,
#16977,#16978,#16979,#16980,#16981,#16982,#16983,#16984,#16985,#16986,#16987,
#16988,#16989,#16990,#16991,#16992,#16993,#16994,#16995,#16996,#16997,#16998,
#16999,#17000,#17001,#17002,#17003,#17004,#17005,#17006,#17007,#17008,#17009,
#17010,#17011,#17012,#17013,#17014,#17015,#17016,#17017,#17018,#17019,#17020,
#17021,#17022,#17023,#17024,#17025,#17026,#17027,#17028,#17029,#17030,#17031,
#17032,#17033,#17034,#17035,#17036,#17037,#17038,#17039),.UNSPECIFIED.,
 .F.,.F.,(4,3,3,3,3,3,3,3,3,3,3,3,3,3,3,3,3,3,3,3,3,3,3,3,3,3,3,3,3,3,3,
3,3,3,3,3,3,3,3,3,3,3,3,3,3,3,3,3,3,3,3,3,3,3,3,3,3,3,3,3,3,3,3,3,3,3,3,
3,3,3,4),(-35.5086755760922,-35.391840750808,-35.3031151892389,-35.2145009894124,
-35.1259745910799,-35.0363195251056,-34.9478891353215,-34.8594706563773,
-34.7710429260415,-34.6804657103525,-34.5919087638597,-34.5003214135726,
-34.4087340632856,-34.3199925014802,-34.231362099372,-34.1428193187148,
-34.0531703258458,-33.9647232179249,-33.8762879250928,-33.7878433041413,
-33.6972893220468,-33.6087154495152,-33.5171714126391,-33.4256273757631,
-33.3368881467887,-33.2482600762056,-33.1597196227201,-33.0700697559102,
-32.9816249486,-32.8931919421141,-32.8047495905072,-32.7141923649406,-32.6256206981239,
-32.5340706931823,-32.4425206882407,-32.3537842240172,-32.2651589703713,
-32.1766213821072,-32.0869704594336,-31.998528617698,-31.9100986091387,
-31.8216592844933,-31.7310979635495,-31.6425293682761,-31.5509716844972,
-31.4594140007182,-31.3706753975655,-31.2820479761503,-31.1935081942323,
-31.1038580841028,-31.0154139993643,-30.9269817333416,-30.8385401393217,
-30.7479819327903,-30.6594110593904,-30.5678591862931,-30.4763073131958,
-30.3875692030748,-30.2989422775513,-30.2104029937242,-30.1207526977179,
-30.0323091131527,-29.9438773471645,-29.8554362524577,-29.7648773457616,
-29.6763069652342,-29.5847537954538,-29.4932006256734,-29.3821251371914,
-29.2726971433069,-29.2254902691016),.UNSPECIFIED.);
#1389=B_SPLINE_CURVE_WITH_KNOTS('',3,(#17041,#17042,#17043,#17044,#17045,
#17046,#17047,#17048,#17049,#17050,#17051,#17052,#17053,#17054,#17055,#17056,
#17057,#17058,#17059,#17060,#17061,#17062,#17063,#17064,#17065,#17066,#17067,
#17068,#17069,#17070,#17071,#17072,#17073,#17074,#17075,#17076,#17077,#17078,
#17079,#17080,#17081,#17082,#17083,#17084,#17085,#17086,#17087,#17088,#17089,
#17090,#17091,#17092,#17093,#17094,#17095,#17096,#17097,#17098,#17099,#17100,
#17101,#17102,#17103,#17104,#17105,#17106,#17107,#17108,#17109,#17110,#17111,
#17112,#17113,#17114,#17115,#17116,#17117,#17118,#17119,#17120,#17121,#17122,
#17123,#17124,#17125,#17126,#17127,#17128,#17129,#17130,#17131,#17132,#17133,
#17134,#17135,#17136,#17137,#17138,#17139,#17140,#17141,#17142,#17143,#17144,
#17145,#17146,#17147,#17148,#17149,#17150,#17151,#17152,#17153,#17154,#17155,
#17156,#17157,#17158,#17159,#17160,#17161,#17162,#17163,#17164,#17165,#17166,
#17167,#17168,#17169,#17170,#17171,#17172,#17173,#17174,#17175,#17176,#17177,
#17178,#17179,#17180,#17181,#17182,#17183,#17184,#17185,#17186,#17187,#17188,
#17189,#17190,#17191,#17192,#17193,#17194,#17195,#17196,#17197,#17198,#17199,
#17200,#17201,#17202,#17203,#17204,#17205,#17206,#17207,#17208,#17209,#17210,
#17211,#17212,#17213,#17214,#17215,#17216,#17217,#17218,#17219,#17220,#17221,
#17222,#17223,#17224,#17225,#17226,#17227,#17228,#17229,#17230,#17231,#17232,
#17233,#17234,#17235,#17236,#17237,#17238,#17239,#17240,#17241,#17242,#17243,
#17244,#17245,#17246,#17247,#17248,#17249,#17250,#17251,#17252,#17253,#17254),
 .UNSPECIFIED.,.F.,.F.,(4,3,3,3,3,3,3,3,3,3,3,3,3,3,3,3,3,3,3,3,3,3,3,3,
3,3,3,3,3,3,3,3,3,3,3,3,3,3,3,3,3,3,3,3,3,3,3,3,3,3,3,3,3,3,3,3,3,3,3,3,
3,3,3,3,3,3,3,3,3,3,3,4),(-29.2254902689126,-29.1360657275674,-29.0484146342724,
-28.9607809341787,-28.8731426670707,-28.7823804848408,-28.694619127601,
-28.602356532876,-28.5100939381509,-28.4213558209058,-28.3327288900596,
-28.2441896027105,-28.1545393087003,-28.0660957251031,-27.9776639617736,
-27.8892228714222,-27.7986639662237,-27.7100935942577,-27.6185404224431,
-27.5269872506285,-27.4382492191399,-27.3496223747916,-27.261083174566,
-27.1714328481335,-27.0829893526203,-26.9945576775742,-26.906116675604,
-26.8155576474795,-26.7269873633194,-26.6354339632127,-26.543880563106,
-26.455142553632,-26.3665157318838,-26.2779765548121,-26.1883262199085,
-26.0998827487654,-26.0114510985026,-25.9230101217026,-25.8324510601728,
-25.7438808019172,-25.6523273387504,-25.5607738755836,-25.4720358320312,
-25.3834089756885,-25.2948697635533,-25.2052194416168,-25.1167759344851,
-25.0283442479519,-24.9399032346396,-24.849344222995,-24.7607739279617,
-24.6692205580114,-24.5776671880611,-24.4889291580206,-24.40030231533,-24.3117631169686,
-24.2221127899148,-24.133669296766,-24.0452376242682,-23.9567966250287,
-23.8662375939062,-23.7776673129069,-23.6861139067228,-23.5945605005387,
-23.5058251646571,-23.4171988003756,-23.3286601402729,-23.2401879892028,
-23.1517561322677,-23.0633474767187,-22.9749248609848,-22.942304961733),
 .UNSPECIFIED.);
#1390=B_SPLINE_CURVE_WITH_KNOTS('',3,(#17256,#17257,#17258,#17259,#17260,
#17261,#17262,#17263,#17264,#17265,#17266,#17267,#17268,#17269,#17270,#17271,
#17272,#17273,#17274,#17275,#17276,#17277,#17278,#17279,#17280,#17281,#17282,
#17283,#17284,#17285,#17286,#17287,#17288,#17289,#17290,#17291,#17292,#17293,
#17294,#17295,#17296,#17297,#17298,#17299,#17300,#17301,#17302,#17303,#17304,
#17305,#17306,#17307,#17308,#17309,#17310,#17311,#17312,#17313,#17314,#17315,
#17316,#17317,#17318,#17319,#17320,#17321,#17322,#17323,#17324,#17325,#17326,
#17327,#17328,#17329,#17330,#17331,#17332,#17333,#17334,#17335,#17336,#17337,
#17338,#17339,#17340,#17341,#17342,#17343,#17344,#17345,#17346,#17347,#17348,
#17349,#17350,#17351,#17352,#17353,#17354,#17355,#17356,#17357,#17358,#17359,
#17360,#17361,#17362,#17363,#17364,#17365,#17366,#17367,#17368,#17369,#17370,
#17371,#17372,#17373,#17374,#17375,#17376,#17377,#17378,#17379,#17380,#17381,
#17382,#17383,#17384,#17385,#17386,#17387,#17388,#17389,#17390,#17391,#17392,
#17393,#17394,#17395,#17396,#17397,#17398,#17399,#17400,#17401,#17402,#17403,
#17404,#17405,#17406,#17407,#17408,#17409,#17410,#17411,#17412,#17413,#17414,
#17415,#17416,#17417,#17418,#17419,#17420,#17421,#17422,#17423,#17424,#17425,
#17426,#17427,#17428,#17429,#17430,#17431,#17432,#17433,#17434,#17435,#17436,
#17437,#17438,#17439,#17440,#17441,#17442,#17443,#17444,#17445,#17446,#17447,
#17448,#17449,#17450,#17451,#17452,#17453,#17454,#17455,#17456,#17457,#17458,
#17459,#17460,#17461,#17462,#17463,#17464,#17465,#17466,#17467,#17468,#17469),
 .UNSPECIFIED.,.F.,.F.,(4,3,3,3,3,3,3,3,3,3,3,3,3,3,3,3,3,3,3,3,3,3,3,3,
3,3,3,3,3,3,3,3,3,3,3,3,3,3,3,3,3,3,3,3,3,3,3,3,3,3,3,3,3,3,3,3,3,3,3,3,
3,3,3,3,3,3,3,3,3,3,3,4),(-22.9423049615399,-22.8400783057738,-22.7372890055352,
-22.6338727274574,-22.6114538130162,-22.522715780268,-22.4340889348564,
-22.3455497337639,-22.2558994077301,-22.1674559118441,-22.0790242366121,
-21.9905832346442,-21.9000242073566,-21.8114539236697,-21.7199005245817,
-21.6283471254938,-21.5396090947594,-21.4509822513892,-21.3624430523631,
-21.2727927255641,-21.1843492317921,-21.095917558688,-21.0074765588595,
-20.9169175286375,-20.8283472470988,-20.736793842535,-20.6452404379713,
-20.5565024051013,-20.4678755595915,-20.3793363584244,-20.2896860324275,
-20.2012425365252,-20.1128108612988,-20.0243698593582,-19.9338108321309,
-19.8452405485253,-19.7536871494871,-19.6621337504489,-19.5733957215263,
-19.4847688799543,-19.3962296827109,-19.3065793552378,-19.2181358631989,
-19.1297041918064,-19.0412631936662,-18.9507041609813,-18.8621338810578,
-18.7705804719922,-18.6790270629265,-18.5902890326888,-18.5016621898394,
-18.4131229913573,-18.3234726643631,-18.235029171188,-18.1465974986995,
-18.0581564995045,-17.9675974684794,-17.879027187612,-17.787473781508,-17.695920375404,
-17.6071823312881,-17.5185554744915,-17.4300162620112,-17.340365940245,
-17.2519224330382,-17.1634907465309,-17.0750497333459,-16.9844907219798,
-16.8959204273232,-16.8043670576024,-16.7128136878816,-16.6591196545534),
 .UNSPECIFIED.);
#1391=B_SPLINE_CURVE_WITH_KNOTS('',3,(#17471,#17472,#17473,#17474,#17475,
#17476,#17477,#17478,#17479,#17480,#17481,#17482,#17483,#17484,#17485,#17486,
#17487,#17488,#17489,#17490,#17491,#17492,#17493,#17494,#17495,#17496,#17497,
#17498,#17499,#17500,#17501,#17502,#17503,#17504,#17505,#17506,#17507,#17508,
#17509,#17510,#17511,#17512,#17513,#17514,#17515,#17516,#17517,#17518,#17519,
#17520,#17521,#17522,#17523,#17524,#17525,#17526,#17527,#17528,#17529,#17530,
#17531,#17532,#17533,#17534,#17535,#17536,#17537,#17538,#17539,#17540,#17541,
#17542,#17543,#17544,#17545,#17546,#17547,#17548,#17549,#17550,#17551,#17552,
#17553,#17554,#17555,#17556,#17557,#17558,#17559,#17560,#17561,#17562,#17563,
#17564,#17565,#17566,#17567,#17568,#17569,#17570,#17571,#17572,#17573,#17574,
#17575,#17576,#17577,#17578,#17579,#17580,#17581,#17582,#17583,#17584,#17585,
#17586,#17587,#17588,#17589,#17590,#17591,#17592,#17593,#17594,#17595,#17596,
#17597,#17598,#17599,#17600,#17601,#17602,#17603,#17604,#17605,#17606,#17607,
#17608,#17609,#17610,#17611,#17612,#17613,#17614,#17615,#17616,#17617,#17618,
#17619,#17620,#17621,#17622,#17623,#17624,#17625,#17626,#17627,#17628,#17629,
#17630,#17631,#17632,#17633,#17634,#17635,#17636,#17637,#17638,#17639,#17640,
#17641,#17642,#17643,#17644,#17645,#17646,#17647,#17648,#17649,#17650,#17651,
#17652,#17653,#17654,#17655,#17656,#17657,#17658,#17659,#17660,#17661,#17662,
#17663,#17664,#17665,#17666,#17667,#17668,#17669,#17670,#17671,#17672,#17673,
#17674,#17675,#17676,#17677,#17678,#17679,#17680,#17681,#17682,#17683,#17684),
 .UNSPECIFIED.,.F.,.F.,(4,3,3,3,3,3,3,3,3,3,3,3,3,3,3,3,3,3,3,3,3,3,3,3,
3,3,3,3,3,3,3,3,3,3,3,3,3,3,3,3,3,3,3,3,3,3,3,3,3,3,3,3,3,3,3,3,3,3,3,3,
3,3,3,3,3,3,3,3,3,3,3,4),(-16.6591196543998,-16.5711052143565,-16.4831981162794,
-16.3953740081479,-16.3076047990417,-16.2198631460269,-16.1321271600137,
-16.0443749611132,-15.9565340199988,-15.868644220512,-15.7806226675453,
-15.7297070003591,-15.6409689666578,-15.5523421205266,-15.4638029189464,
-15.3741525931827,-15.2857090973743,-15.1972774224304,-15.1088364209597,
-15.0182773939289,-14.9297071112482,-14.8381537120424,-14.7466003128367,
-14.657862192562,-14.5692352592747,-14.4806959700712,-14.3910456769766,
-14.3026020929753,-14.2141703297856,-14.1257292401177,-14.0351703364169,
-13.9465999664761,-13.8550467958951,-13.7634936253142,-13.6747557987345,
-13.5861291595026,-13.4975901643472,-13.4079397610277,-13.3194964691629,
-13.2310649968712,-13.1426241965351,-13.0520648818493,-12.9634947947155,
-12.8719408662536,-12.7803869377918,-12.6916488057979,-12.6030218626512,
-12.5144825654337,-12.4248322760381,-12.3363886885555,-12.2479569235773,
-12.1595158338075,-12.068956937923,-11.9803865720187,-11.888833411144,-11.7972802502693,
-11.7085416347909,-11.6199142034448,-11.5313744139808,-11.4417243075765,
-11.3532802211941,-11.2648479557407,-11.1764063645028,-11.0858481640638,
-10.9972772989043,-10.9057254308256,-10.8141735627469,-10.7185150588642,
-10.6231617411537,-10.5279991843888,-10.4331223296681,-10.3759343476128),
 .UNSPECIFIED.);
#1392=B_SPLINE_CURVE_WITH_KNOTS('',3,(#17685,#17686,#17687,#17688,#17689,
#17690,#17691,#17692,#17693,#17694,#17695,#17696,#17697,#17698,#17699,#17700,
#17701,#17702,#17703,#17704,#17705,#17706,#17707,#17708,#17709,#17710,#17711,
#17712,#17713,#17714,#17715,#17716,#17717,#17718,#17719,#17720,#17721,#17722,
#17723,#17724,#17725,#17726,#17727,#17728,#17729,#17730,#17731,#17732,#17733,
#17734,#17735,#17736,#17737,#17738,#17739,#17740,#17741,#17742,#17743,#17744,
#17745,#17746,#17747,#17748,#17749,#17750,#17751,#17752,#17753,#17754,#17755,
#17756,#17757,#17758,#17759,#17760,#17761,#17762,#17763,#17764,#17765,#17766,
#17767,#17768,#17769,#17770,#17771,#17772,#17773,#17774,#17775,#17776,#17777,
#17778,#17779,#17780,#17781,#17782,#17783,#17784,#17785,#17786,#17787,#17788,
#17789,#17790,#17791,#17792,#17793,#17794,#17795,#17796,#17797,#17798,#17799,
#17800,#17801,#17802,#17803,#17804,#17805,#17806,#17807,#17808,#17809,#17810,
#17811,#17812,#17813,#17814,#17815,#17816,#17817,#17818,#17819,#17820,#17821,
#17822,#17823,#17824,#17825,#17826,#17827,#17828,#17829,#17830,#17831,#17832,
#17833,#17834,#17835,#17836,#17837,#17838,#17839,#17840,#17841,#17842,#17843,
#17844,#17845,#17846,#17847,#17848,#17849,#17850,#17851,#17852,#17853,#17854,
#17855,#17856,#17857,#17858,#17859,#17860,#17861,#17862,#17863,#17864,#17865,
#17866,#17867,#17868,#17869,#17870,#17871,#17872,#17873,#17874,#17875,#17876,
#17877,#17878,#17879,#17880,#17881,#17882,#17883,#17884,#17885,#17886,#17887,
#17888,#17889,#17890,#17891,#17892,#17893,#17894,#17895,#17896,#17897,#17898),
 .UNSPECIFIED.,.F.,.F.,(4,3,3,3,3,3,3,3,3,3,3,3,3,3,3,3,3,3,3,3,3,3,3,3,
3,3,3,3,3,3,3,3,3,3,3,3,3,3,3,3,3,3,3,3,3,3,3,3,3,3,3,3,3,3,3,3,3,3,3,3,
3,3,3,3,3,3,3,3,3,3,3,4),(-10.3759343473738,-10.2851902025472,-10.1943848714136,
-10.1034269336437,-10.0123921171029,-9.92117043902683,-9.83106687522445,
-9.74232744591289,-9.65369921391586,-9.56515863778241,-9.47550883152236,
-9.38706399749244,-9.29863100026054,-9.2101886938749,-9.11963156733168,
-9.03106003445256,-8.93951011107729,-8.84796018770201,-8.75921862146023,
-8.67058821577755,-8.58204543240453,-8.49239644087641,-8.40394933236375,
-8.3155140397366,-8.22706941978681,-8.136515439885,-8.04794157031955,-7.95639753524956,
-7.86485350017956,-7.77612873502284,-7.68751517689834,-7.59898926618254,
-7.50933395949186,-7.42090367598821,-7.33248516033964,-7.2440572503412,
-7.15347964092018,-7.06492216206265,-6.97333448735988,-6.88174681265711,
-6.79299349255972,-6.70435142178096,-6.61579707521975,-6.52615245645912,
-6.43769410689579,-6.34924771344436,-6.2607921449874,-6.17025414002422,
-6.08166979716281,-5.99015496114874,-5.89864012513467,-5.80988349345781,
-5.721237834732,-5.6326796322351,-5.54303635790724,-5.45457352676152,-5.36612242704649,
-5.27766193421025,-5.18712981006075,-5.09854005361742,-5.00703674561482,
-4.91553343761222,-4.82816672719067,-4.74091103291585,-4.65375084014162,
-4.56664302899291,-4.47956514860665,-4.39249477953229,-4.30537257831964,
-4.21822093231598,-4.13097249351553,-4.09274904019425),.UNSPECIFIED.);
#1393=B_SPLINE_CURVE_WITH_KNOTS('',3,(#17901,#17902,#17903,#17904,#17905,
#17906,#17907,#17908,#17909,#17910,#17911,#17912,#17913,#17914,#17915,#17916,
#17917,#17918,#17919,#17920,#17921,#17922,#17923,#17924,#17925,#17926,#17927,
#17928,#17929,#17930,#17931,#17932,#17933,#17934,#17935,#17936,#17937,#17938,
#17939,#17940,#17941,#17942,#17943,#17944,#17945,#17946,#17947,#17948,#17949,
#17950,#17951,#17952,#17953,#17954,#17955,#17956,#17957,#17958,#17959,#17960,
#17961,#17962,#17963,#17964,#17965,#17966,#17967,#17968,#17969,#17970,#17971,
#17972,#17973,#17974,#17975,#17976,#17977,#17978,#17979,#17980,#17981,#17982,
#17983,#17984,#17985,#17986,#17987,#17988,#17989,#17990,#17991,#17992,#17993,
#17994,#17995,#17996,#17997,#17998,#17999,#18000,#18001,#18002,#18003,#18004,
#18005,#18006,#18007,#18008,#18009,#18010,#18011,#18012,#18013,#18014,#18015,
#18016,#18017,#18018,#18019,#18020,#18021,#18022,#18023,#18024,#18025,#18026,
#18027,#18028,#18029,#18030,#18031,#18032,#18033,#18034,#18035,#18036),
 .UNSPECIFIED.,.F.,.F.,(4,2,2,2,2,2,2,2,2,2,2,2,2,2,2,2,2,2,2,2,2,2,2,2,
2,2,2,2,2,2,2,2,2,2,2,2,2,2,2,2,2,2,2,2,2,2,2,2,2,2,2,2,2,2,2,2,2,2,2,2,
2,2,2,2,2,2,2,4),(-1.77559603949032,-1.76123154608128,-1.7347774998451,
-1.72014143363947,-1.7068339629146,-1.68857155834236,-1.63315424891479,
-1.57627821739527,-1.56425230882687,-1.556637450491,-1.54787596729481,-1.52991828878332,
-1.50294441993861,-1.42904210726485,-1.41020593191291,-1.39681096212694,
-1.38237120796975,-1.35716756233058,-1.32297978190903,-1.25979963496362,
-1.24717229379129,-1.24013906968697,-1.23183624951668,-1.21654647058489,
-1.13819900867779,-1.10478593438375,-1.0886994354341,-1.07552469652321,
-1.05938339279416,-1.0221529379589,-0.945373097674644,-0.931168721675339,
-0.923086896639897,-0.914980731472239,-0.900470464774507,-0.829383392842492,
-0.788686358912283,-0.771942396221659,-0.758847828752075,-0.743525574560414,
-0.712224269767771,-0.662032602029656,-0.624325944085348,-0.611799382621773,
-0.604806613441647,-0.596524834506089,-0.581312003040091,-0.560333974050935,
-0.520212979478024,-0.475549380629993,-0.456720884664485,-0.443279701400228,
-0.428738464622379,-0.403165689810354,-0.368178944476579,-0.303773218212403,
-0.292552367632876,-0.284863377728665,-0.27529201983579,-0.252724455737363,
-0.21291224578363,-0.161665817941933,-0.142706624100451,-0.129150343477715,
-0.114427133356919,-0.0883041265988544,-0.0523412071009701,-0.00482582262840578),
 .UNSPECIFIED.);
#1394=B_SPLINE_CURVE_WITH_KNOTS('',3,(#18039,#18040,#18041,#18042,#18043,
#18044,#18045,#18046,#18047,#18048,#18049,#18050,#18051,#18052,#18053,#18054,
#18055,#18056,#18057,#18058,#18059,#18060,#18061,#18062,#18063,#18064,#18065,
#18066,#18067,#18068,#18069,#18070,#18071,#18072,#18073,#18074,#18075,#18076,
#18077,#18078,#18079,#18080,#18081,#18082,#18083,#18084,#18085,#18086,#18087,
#18088,#18089,#18090,#18091,#18092,#18093,#18094,#18095,#18096,#18097,#18098,
#18099,#18100,#18101,#18102,#18103,#18104,#18105,#18106,#18107,#18108,#18109,
#18110,#18111,#18112,#18113,#18114,#18115,#18116,#18117,#18118,#18119,#18120,
#18121,#18122,#18123,#18124,#18125,#18126,#18127,#18128,#18129,#18130,#18131,
#18132,#18133,#18134,#18135,#18136,#18137,#18138,#18139,#18140,#18141,#18142,
#18143,#18144),.UNSPECIFIED.,.F.,.F.,(4,2,2,2,2,2,2,2,2,2,2,2,2,2,2,2,2,
2,2,2,2,2,2,2,2,2,2,2,2,2,2,2,2,2,2,2,2,2,2,2,2,2,2,2,2,2,2,2,2,2,2,2,4),
(-12.994627603384,-12.9875915521804,-12.9782754205316,-12.91699009307,-12.8731839129498,
-12.8557803975354,-12.8411540685734,-12.8227464552579,-12.7725470591221,
-12.7193211253437,-12.7007430540061,-12.686661419049,-12.6785554299798,
-12.6716500633205,-12.6589777049455,-12.5974421893282,-12.5499643410219,
-12.5317837785489,-12.5189811364405,-12.5053727543902,-12.4824936301464,
-12.4029450770898,-12.3819658998937,-12.366872420079,-12.3588855294487,
-12.3510968527962,-12.3383610505868,-12.2890655093762,-12.2464093533266,
-12.2175336782031,-12.2023791798903,-12.1889491752564,-12.1713159235955,
-12.1010906625992,-12.0721209918708,-12.0533384615127,-12.0443296945605,
-12.0365996637125,-12.024361864911,-11.9695325441213,-11.9302485028225,
-11.9028319644802,-11.8879963913662,-11.874653921784,-11.8565653989144,
-11.7774418205882,-11.7521961895244,-11.7349780097399,-11.7263341382877,
-11.7186941679461,-11.7064021195052,-11.654545056237,-11.6209589861144),
 .UNSPECIFIED.);
#1395=B_SPLINE_CURVE_WITH_KNOTS('',3,(#18192,#18193,#18194,#18195,#18196,
#18197,#18198,#18199,#18200,#18201,#18202,#18203,#18204,#18205),
 .UNSPECIFIED.,.F.,.F.,(4,2,2,2,2,2,4),(-0.00536726278181953,-2.59148391548031E-9,
0.103199421735768,0.207237881907438,0.325153852544771,0.397240462561985,
0.468984198664975),.UNSPECIFIED.);
#1396=B_SPLINE_CURVE_WITH_KNOTS('',3,(#18207,#18208,#18209,#18210,#18211,
#18212,#18213,#18214,#18215),.UNSPECIFIED.,.F.,.F.,(4,1,1,1,1,1,4),(-0.0350009593777651,
-0.0280198960523448,-0.0168045420304008,-0.00558918800845676,0.00562616601348723,
0.0280568740573752,0.0350536102859934),.UNSPECIFIED.);
#1397=B_SPLINE_CURVE_WITH_KNOTS('',3,(#18217,#18218,#18219,#18220,#18221,
#18222,#18223,#18224,#18225,#18226,#18227,#18228,#18229,#18230),
 .UNSPECIFIED.,.F.,.F.,(4,2,2,2,2,2,4),(0.,0.0545964532303548,0.109457297997855,
0.199283875927555,0.278528214008273,0.35702335445668,0.361102531747097),
 .UNSPECIFIED.);
#1398=B_SPLINE_CURVE_WITH_KNOTS('',3,(#18241,#18242,#18243,#18244,#18245,
#18246,#18247,#18248,#18249,#18250,#18251,#18252,#18253,#18254,#18255,#18256,
#18257,#18258,#18259,#18260,#18261,#18262,#18263,#18264,#18265,#18266,#18267,
#18268,#18269,#18270,#18271,#18272,#18273,#18274,#18275,#18276,#18277,#18278,
#18279,#18280,#18281,#18282,#18283,#18284,#18285,#18286,#18287,#18288,#18289),
 .UNSPECIFIED.,.F.,.F.,(4,3,3,3,3,3,3,3,3,3,3,3,3,3,3,3,4),(-0.0350029182876339,
-0.0326784274410288,-0.0303491617466868,-0.0280198960523449,-0.0254680708026916,
-0.0229201060834388,-0.020374904247847,-0.017833637297367,-0.0168045420304009,
-0.0144744225215027,-0.0121456147918491,-0.00981763946125116,-0.00748894401297814,
-0.0055891880084569,-0.00301831184103368,-0.00044459753078153,-5.93799746765259E-12),
 .UNSPECIFIED.);
#1399=B_SPLINE_CURVE_WITH_KNOTS('',3,(#18292,#18293,#18294,#18295,#18296,
#18297,#18298),.UNSPECIFIED.,.F.,.F.,(4,3,4),(-0.0490510097259757,0.,0.0490510097259755),
 .UNSPECIFIED.);
#1400=B_SPLINE_CURVE_WITH_KNOTS('',3,(#18300,#18301,#18302,#18303,#18304,
#18305),.UNSPECIFIED.,.F.,.F.,(4,2,4),(-0.954074778386005,-0.905023768660029,
-0.855972758934053),.UNSPECIFIED.);
#1401=B_SPLINE_CURVE_WITH_KNOTS('',3,(#18308,#18309,#18310,#18311,#18312,
#18313,#18314,#18315,#18316,#18317,#18318,#18319,#18320,#18321,#18322,#18323,
#18324,#18325,#18326,#18327,#18328,#18329,#18330,#18331,#18332,#18333,#18334,
#18335,#18336,#18337,#18338,#18339,#18340,#18341,#18342,#18343,#18344,#18345,
#18346,#18347,#18348,#18349,#18350,#18351,#18352,#18353,#18354,#18355,#18356),
 .UNSPECIFIED.,.F.,.F.,(4,3,3,3,3,3,3,3,3,3,3,3,3,3,3,3,4),(0.,0.00256903263786249,
0.00514025172138199,0.00562616601348712,0.0081513990320383,0.0106763832495211,
0.0132007965397256,0.0157247404553983,0.0168415200354311,0.0191777542451066,
0.0215147787392673,0.0238521408034104,0.026192082316959,0.0280568740573752,
0.030597682690626,0.033145701984153,0.0350439206609343),.UNSPECIFIED.);
#1402=B_SPLINE_CURVE_WITH_KNOTS('',3,(#18411,#18412,#18413,#18414,#18415,
#18416,#18417,#18418,#18419,#18420,#18421,#18422,#18423,#18424),
 .UNSPECIFIED.,.F.,.F.,(4,2,2,2,2,2,4),(-0.361103617303379,-0.357017748906342,
-0.278455831096292,-0.199256530150916,-0.109493107705783,-0.0546164016226888,
-6.26706830986201E-7),.UNSPECIFIED.);
#1403=B_SPLINE_CURVE_WITH_KNOTS('',3,(#18426,#18427,#18428,#18429,#18430,
#18431,#18432,#18433,#18434,#18435,#18436,#18437,#18438,#18439),
 .UNSPECIFIED.,.F.,.F.,(4,2,2,2,2,2,4),(-0.469007914525735,-0.397274254527166,
-0.325193332432218,-0.207246009609002,-0.103181568409207,0.,0.00535948636125596),
 .UNSPECIFIED.);
#1404=B_SPLINE_CURVE_WITH_KNOTS('',3,(#18628,#18629,#18630,#18631,#18632,
#18633,#18634,#18635,#18636,#18637,#18638,#18639,#18640,#18641,#18642,#18643,
#18644,#18645,#18646,#18647,#18648,#18649,#18650,#18651,#18652,#18653,#18654,
#18655,#18656,#18657,#18658,#18659,#18660,#18661,#18662,#18663,#18664,#18665,
#18666,#18667,#18668,#18669,#18670,#18671,#18672,#18673,#18674,#18675,#18676,
#18677,#18678,#18679,#18680,#18681,#18682,#18683,#18684,#18685,#18686,#18687,
#18688,#18689,#18690,#18691,#18692,#18693,#18694,#18695,#18696,#18697,#18698,
#18699,#18700,#18701,#18702,#18703,#18704,#18705,#18706,#18707,#18708,#18709,
#18710,#18711,#18712),.UNSPECIFIED.,.F.,.F.,(4,3,3,3,3,3,3,3,3,3,3,3,3,
3,3,3,3,3,3,3,3,3,3,3,3,3,3,3,4),(5.93772547493953E-5,0.0374260888262869,
0.0738564267296499,0.110770159938098,0.147683893146547,0.154011688621638,
0.189882099992678,0.225711180046048,0.260784282188391,0.292370020163279,
0.299381408876867,0.333941591811059,0.367613151733489,0.401093479558722,
0.407459990826463,0.436280771759322,0.441113261645755,0.474765163706684,
0.50871732282195,0.542418769600373,0.567449717218624,0.575264939175507,
0.60833260900008,0.640763136698678,0.657717726095142,0.662787221699447,
0.694639312545765,0.725626255150186,0.744397949170602),.UNSPECIFIED.);
#1405=B_SPLINE_CURVE_WITH_KNOTS('',3,(#18714,#18715,#18716,#18717,#18718,
#18719,#18720,#18721,#18722,#18723,#18724,#18725,#18726,#18727,#18728,#18729,
#18730,#18731,#18732,#18733,#18734,#18735,#18736,#18737,#18738,#18739,#18740,
#18741,#18742,#18743,#18744,#18745,#18746,#18747,#18748,#18749,#18750,#18751,
#18752,#18753,#18754,#18755,#18756,#18757,#18758,#18759,#18760,#18761,#18762,
#18763,#18764,#18765,#18766,#18767,#18768,#18769,#18770,#18771,#18772,#18773,
#18774,#18775,#18776,#18777,#18778,#18779,#18780,#18781,#18782,#18783,#18784,
#18785,#18786,#18787,#18788,#18789,#18790,#18791,#18792,#18793,#18794,#18795,
#18796,#18797,#18798,#18799,#18800,#18801,#18802,#18803,#18804),
 .UNSPECIFIED.,.F.,.F.,(4,3,3,3,3,3,3,3,3,3,3,3,3,3,3,3,3,3,3,3,3,3,3,3,
3,3,3,3,3,3,4),(0.,0.0309970440507718,0.0619955277647955,0.0939113023789225,
0.122434839440515,0.12758455026797,0.132227190796814,0.164899763317829,
0.198101502938401,0.231586044786447,0.259311605376256,0.263977965982227,
0.298334414351843,0.333236562478584,0.368138710605325,0.370114527877473,
0.398052464733428,0.403189970392264,0.437098301742969,0.471632442026652,
0.506863545933039,0.53577203760693,0.541093903690208,0.546417846440992,
0.582336732445268,0.618540903512682,0.634760608889732,0.641019432752641,
0.67784978911133,0.714258333683681,0.74127076840638),.UNSPECIFIED.);
#1406=B_SPLINE_CURVE_WITH_KNOTS('',3,(#18805,#18806,#18807,#18808),
 .UNSPECIFIED.,.F.,.F.,(4,4),(-0.0121139156679117,0.),.UNSPECIFIED.);
#1407=B_SPLINE_CURVE_WITH_KNOTS('',3,(#18994,#18995,#18996,#18997,#18998,
#18999,#19000,#19001,#19002,#19003,#19004,#19005,#19006,#19007,#19008,#19009,
#19010,#19011,#19012,#19013,#19014,#19015,#19016,#19017,#19018,#19019,#19020,
#19021,#19022,#19023,#19024,#19025,#19026,#19027,#19028,#19029,#19030,#19031,
#19032,#19033,#19034,#19035,#19036,#19037,#19038,#19039,#19040,#19041,#19042,
#19043,#19044,#19045,#19046,#19047,#19048,#19049,#19050,#19051,#19052,#19053,
#19054,#19055,#19056,#19057,#19058,#19059,#19060,#19061,#19062,#19063,#19064,
#19065,#19066,#19067,#19068,#19069,#19070,#19071,#19072,#19073,#19074,#19075,
#19076,#19077,#19078,#19079,#19080,#19081,#19082,#19083,#19084,#19085,#19086,
#19087,#19088,#19089,#19090),.UNSPECIFIED.,.F.,.F.,(4,3,3,3,3,3,3,3,3,3,
3,3,3,3,3,3,3,3,3,3,3,3,3,3,3,3,3,3,3,3,3,3,4),(0.,0.0309970440507677,0.0619181010064114,
0.0937144809078779,0.110912695544682,0.122435055735921,0.127584942037278,
0.132227280497855,0.1648998786022,0.198101629608467,0.231586168644273,0.259311708386001,
0.263978079994448,0.298334530993182,0.333236654183239,0.368138777373297,
0.370114527877469,0.393311792910526,0.398370229703331,0.403189968677661,
0.437098316226467,0.471632477527816,0.506863596722405,0.535772077628709,
0.541093944718474,0.546417849114959,0.582336753940169,0.618540921884149,
0.634760639680576,0.641019471053442,0.677849826923293,0.714258330886494,
0.741270768406381),.UNSPECIFIED.);
#1408=B_SPLINE_CURVE_WITH_KNOTS('',3,(#19091,#19092,#19093,#19094),
 .UNSPECIFIED.,.F.,.F.,(4,4),(0.,0.0121134590555018),.UNSPECIFIED.);
#1409=B_SPLINE_CURVE_WITH_KNOTS('',3,(#19095,#19096,#19097,#19098,#19099,
#19100,#19101,#19102,#19103,#19104,#19105,#19106,#19107,#19108,#19109,#19110,
#19111,#19112,#19113,#19114,#19115,#19116,#19117,#19118,#19119,#19120,#19121,
#19122,#19123,#19124,#19125,#19126,#19127,#19128,#19129,#19130,#19131,#19132,
#19133,#19134,#19135,#19136,#19137,#19138,#19139,#19140,#19141,#19142,#19143,
#19144,#19145,#19146,#19147,#19148,#19149,#19150,#19151,#19152,#19153,#19154,
#19155,#19156,#19157,#19158,#19159,#19160,#19161,#19162,#19163,#19164,#19165,
#19166,#19167,#19168,#19169,#19170,#19171,#19172,#19173,#19174,#19175,#19176,
#19177,#19178,#19179,#19180,#19181,#19182,#19183,#19184,#19185,#19186,#19187,
#19188),.UNSPECIFIED.,.F.,.F.,(4,3,3,3,3,3,3,3,3,3,3,3,3,3,3,3,3,3,3,3,
3,3,3,3,3,3,3,3,3,3,3,4),(0.,0.0374260888263008,0.0738564290320547,0.110770162397625,
0.147683895763195,0.154011692627707,0.189882104065088,0.225711192227168,
0.260784326226137,0.292370154409116,0.299381403642943,0.333917720960345,
0.36795450999486,0.401093586298063,0.407459990826479,0.428518613222987,
0.434552801562352,0.439572347501266,0.441113258225818,0.474677870938634,
0.508628197894967,0.54247978601399,0.558802088782934,0.568708698403076,
0.576616421709766,0.609674167629691,0.642088946178112,0.657717694151321,
0.662787189531987,0.694639229192994,0.725626103462853,0.744397949170599),
 .UNSPECIFIED.);
#1641=VERTEX_POINT('',#13646);
#1642=VERTEX_POINT('',#13647);
#1643=VERTEX_POINT('',#13649);
#1644=VERTEX_POINT('',#13760);
#1645=VERTEX_POINT('',#13845);
#1646=VERTEX_POINT('',#13846);
#1647=VERTEX_POINT('',#14167);
#1648=VERTEX_POINT('',#14168);
#1649=VERTEX_POINT('',#14489);
#1650=VERTEX_POINT('',#14490);
#1651=VERTEX_POINT('',#14815);
#1652=VERTEX_POINT('',#14816);
#1653=VERTEX_POINT('',#15135);
#1654=VERTEX_POINT('',#15136);
#1655=VERTEX_POINT('',#15457);
#1656=VERTEX_POINT('',#15458);
#1657=VERTEX_POINT('',#15465);
#1658=VERTEX_POINT('',#15467);
#1659=VERTEX_POINT('',#15473);
#1660=VERTEX_POINT('',#15688);
#1661=VERTEX_POINT('',#15903);
#1662=VERTEX_POINT('',#16115);
#1663=VERTEX_POINT('',#16126);
#1664=VERTEX_POINT('',#16338);
#1665=VERTEX_POINT('',#16553);
#1666=VERTEX_POINT('',#16603);
#1667=VERTEX_POINT('',#16605);
#1668=VERTEX_POINT('',#16610);
#1669=VERTEX_POINT('',#16828);
#1670=VERTEX_POINT('',#17040);
#1671=VERTEX_POINT('',#17255);
#1672=VERTEX_POINT('',#17470);
#1673=VERTEX_POINT('',#17900);
#1674=VERTEX_POINT('',#18037);
#1675=VERTEX_POINT('',#18190);
#1676=VERTEX_POINT('',#18191);
#1677=VERTEX_POINT('',#18206);
#1678=VERTEX_POINT('',#18216);
#1679=VERTEX_POINT('',#18233);
#1680=VERTEX_POINT('',#18235);
#1681=VERTEX_POINT('',#18239);
#1682=VERTEX_POINT('',#18240);
#1683=VERTEX_POINT('',#18290);
#1684=VERTEX_POINT('',#18299);
#1685=VERTEX_POINT('',#18306);
#1686=VERTEX_POINT('',#18357);
#1687=VERTEX_POINT('',#18410);
#1688=VERTEX_POINT('',#18425);
#1689=VERTEX_POINT('',#18713);
#1690=VERTEX_POINT('',#18993);
#2141=EDGE_CURVE('',#1641,#1642,#1040,.T.);
#2142=EDGE_CURVE('',#1643,#1641,#1365,.F.);
#2143=EDGE_CURVE('',#1644,#1643,#192,.T.);
#2144=EDGE_CURVE('',#1644,#1642,#1366,.T.);
#2145=EDGE_CURVE('',#1645,#1646,#1041,.T.);
#2146=EDGE_CURVE('',#1641,#1645,#1367,.F.);
#2147=EDGE_CURVE('',#1642,#1646,#1368,.T.);
#2148=EDGE_CURVE('',#1647,#1648,#1042,.T.);
#2149=EDGE_CURVE('',#1645,#1647,#1369,.F.);
#2150=EDGE_CURVE('',#1646,#1648,#1370,.T.);
#2151=EDGE_CURVE('',#1649,#1650,#1043,.T.);
#2152=EDGE_CURVE('',#1647,#1649,#1371,.F.);
#2153=EDGE_CURVE('',#1648,#1650,#1372,.T.);
#2154=EDGE_CURVE('',#1651,#1652,#1044,.T.);
#2155=EDGE_CURVE('',#1649,#1651,#1373,.F.);
#2156=EDGE_CURVE('',#1650,#1652,#1374,.T.);
#2157=EDGE_CURVE('',#1653,#1654,#1045,.T.);
#2158=EDGE_CURVE('',#1651,#1653,#1375,.F.);
#2159=EDGE_CURVE('',#1652,#1654,#1376,.T.);
#2160=EDGE_CURVE('',#1655,#1656,#1377,.T.);
#2161=EDGE_CURVE('',#1657,#1656,#193,.F.);
#2162=EDGE_CURVE('',#1657,#1658,#1378,.T.);
#2163=EDGE_CURVE('',#1658,#1659,#1379,.T.);
#2164=EDGE_CURVE('',#1659,#1660,#1380,.T.);
#2165=EDGE_CURVE('',#1660,#1661,#1381,.T.);
#2166=EDGE_CURVE('',#1661,#1662,#1382,.T.);
#2167=EDGE_CURVE('',#1662,#1663,#1383,.T.);
#2168=EDGE_CURVE('',#1663,#1664,#1384,.T.);
#2169=EDGE_CURVE('',#1664,#1665,#1385,.T.);
#2170=EDGE_CURVE('',#1666,#1665,#194,.T.);
#2171=EDGE_CURVE('',#1666,#1667,#1386,.T.);
#2172=EDGE_CURVE('',#1667,#1668,#1387,.T.);
#2173=EDGE_CURVE('',#1668,#1669,#1388,.T.);
#2174=EDGE_CURVE('',#1669,#1670,#1389,.T.);
#2175=EDGE_CURVE('',#1670,#1671,#1390,.T.);
#2176=EDGE_CURVE('',#1671,#1672,#1391,.T.);
#2177=EDGE_CURVE('',#1672,#1655,#1392,.T.);
#2178=EDGE_CURVE('',#1654,#1673,#1393,.T.);
#2179=EDGE_CURVE('',#1674,#1673,#195,.T.);
#2180=EDGE_CURVE('',#1653,#1674,#1394,.F.);
#2181=EDGE_CURVE('',#1675,#1676,#1395,.T.);
#2182=EDGE_CURVE('',#1676,#1677,#1396,.T.);
#2183=EDGE_CURVE('',#1677,#1678,#1397,.T.);
#2184=EDGE_CURVE('',#1678,#1675,#1046,.T.);
#2185=EDGE_CURVE('',#1679,#1677,#1047,.T.);
#2186=EDGE_CURVE('',#1680,#1679,#196,.T.);
#2187=EDGE_CURVE('',#1676,#1680,#1048,.T.);
#2188=EDGE_CURVE('',#1681,#1682,#1398,.T.);
#2189=EDGE_CURVE('',#1681,#1683,#1049,.T.);
#2190=EDGE_CURVE('',#1683,#1679,#1399,.T.);
#2191=EDGE_CURVE('',#1680,#1684,#1400,.T.);
#2192=EDGE_CURVE('',#1684,#1685,#1050,.T.);
#2193=EDGE_CURVE('',#1682,#1685,#1401,.T.);
#2194=EDGE_CURVE('',#1682,#1686,#1051,.T.);
#2195=EDGE_CURVE('',#1686,#1686,#197,.T.);
#2196=EDGE_CURVE('',#1687,#1681,#1402,.T.);
#2197=EDGE_CURVE('',#1685,#1688,#1403,.T.);
#2198=EDGE_CURVE('',#1688,#1687,#1052,.T.);
#2199=EDGE_CURVE('',#1683,#1684,#198,.T.);
#2200=EDGE_CURVE('',#1665,#1674,#1404,.T.);
#2201=EDGE_CURVE('',#1689,#1657,#1405,.T.);
#2202=EDGE_CURVE('',#1689,#1643,#1406,.T.);
#2203=EDGE_CURVE('',#1690,#1666,#1407,.T.);
#2204=EDGE_CURVE('',#1673,#1690,#1408,.T.);
#2205=EDGE_CURVE('',#1656,#1644,#1409,.T.);
#2953=ORIENTED_EDGE('',*,*,#2141,.F.);
#2954=ORIENTED_EDGE('',*,*,#2142,.F.);
#2955=ORIENTED_EDGE('',*,*,#2143,.F.);
#2956=ORIENTED_EDGE('',*,*,#2144,.T.);
#2957=ORIENTED_EDGE('',*,*,#2145,.F.);
#2958=ORIENTED_EDGE('',*,*,#2146,.F.);
#2959=ORIENTED_EDGE('',*,*,#2141,.T.);
#2960=ORIENTED_EDGE('',*,*,#2147,.T.);
#2961=ORIENTED_EDGE('',*,*,#2148,.F.);
#2962=ORIENTED_EDGE('',*,*,#2149,.F.);
#2963=ORIENTED_EDGE('',*,*,#2145,.T.);
#2964=ORIENTED_EDGE('',*,*,#2150,.T.);
#2965=ORIENTED_EDGE('',*,*,#2151,.F.);
#2966=ORIENTED_EDGE('',*,*,#2152,.F.);
#2967=ORIENTED_EDGE('',*,*,#2148,.T.);
#2968=ORIENTED_EDGE('',*,*,#2153,.T.);
#2969=ORIENTED_EDGE('',*,*,#2154,.F.);
#2970=ORIENTED_EDGE('',*,*,#2155,.F.);
#2971=ORIENTED_EDGE('',*,*,#2151,.T.);
#2972=ORIENTED_EDGE('',*,*,#2156,.T.);
#2973=ORIENTED_EDGE('',*,*,#2157,.F.);
#2974=ORIENTED_EDGE('',*,*,#2158,.F.);
#2975=ORIENTED_EDGE('',*,*,#2154,.T.);
#2976=ORIENTED_EDGE('',*,*,#2159,.T.);
#2977=ORIENTED_EDGE('',*,*,#2160,.T.);
#2978=ORIENTED_EDGE('',*,*,#2161,.F.);
#2979=ORIENTED_EDGE('',*,*,#2162,.T.);
#2980=ORIENTED_EDGE('',*,*,#2163,.T.);
#2981=ORIENTED_EDGE('',*,*,#2164,.T.);
#2982=ORIENTED_EDGE('',*,*,#2165,.T.);
#2983=ORIENTED_EDGE('',*,*,#2166,.T.);
#2984=ORIENTED_EDGE('',*,*,#2167,.T.);
#2985=ORIENTED_EDGE('',*,*,#2168,.T.);
#2986=ORIENTED_EDGE('',*,*,#2169,.T.);
#2987=ORIENTED_EDGE('',*,*,#2170,.F.);
#2988=ORIENTED_EDGE('',*,*,#2171,.T.);
#2989=ORIENTED_EDGE('',*,*,#2172,.T.);
#2990=ORIENTED_EDGE('',*,*,#2173,.T.);
#2991=ORIENTED_EDGE('',*,*,#2174,.T.);
#2992=ORIENTED_EDGE('',*,*,#2175,.T.);
#2993=ORIENTED_EDGE('',*,*,#2176,.T.);
#2994=ORIENTED_EDGE('',*,*,#2177,.T.);
#2995=ORIENTED_EDGE('',*,*,#2157,.T.);
#2996=ORIENTED_EDGE('',*,*,#2178,.T.);
#2997=ORIENTED_EDGE('',*,*,#2179,.F.);
#2998=ORIENTED_EDGE('',*,*,#2180,.F.);
#2999=ORIENTED_EDGE('',*,*,#2181,.T.);
#3000=ORIENTED_EDGE('',*,*,#2182,.T.);
#3001=ORIENTED_EDGE('',*,*,#2183,.T.);
#3002=ORIENTED_EDGE('',*,*,#2184,.T.);
#3003=ORIENTED_EDGE('',*,*,#2183,.F.);
#3004=ORIENTED_EDGE('',*,*,#2185,.F.);
#3005=ORIENTED_EDGE('',*,*,#2186,.F.);
#3006=ORIENTED_EDGE('',*,*,#2187,.F.);
#3007=ORIENTED_EDGE('',*,*,#2181,.F.);
#3008=ORIENTED_EDGE('',*,*,#2184,.F.);
#3009=ORIENTED_EDGE('',*,*,#2188,.F.);
#3010=ORIENTED_EDGE('',*,*,#2189,.T.);
#3011=ORIENTED_EDGE('',*,*,#2190,.T.);
#3012=ORIENTED_EDGE('',*,*,#2185,.T.);
#3013=ORIENTED_EDGE('',*,*,#2182,.F.);
#3014=ORIENTED_EDGE('',*,*,#2187,.T.);
#3015=ORIENTED_EDGE('',*,*,#2191,.T.);
#3016=ORIENTED_EDGE('',*,*,#2192,.T.);
#3017=ORIENTED_EDGE('',*,*,#2193,.F.);
#3018=ORIENTED_EDGE('',*,*,#2194,.T.);
#3019=ORIENTED_EDGE('',*,*,#2195,.T.);
#3020=ORIENTED_EDGE('',*,*,#2194,.F.);
#3021=ORIENTED_EDGE('',*,*,#2196,.T.);
#3022=ORIENTED_EDGE('',*,*,#2188,.T.);
#3023=ORIENTED_EDGE('',*,*,#2193,.T.);
#3024=ORIENTED_EDGE('',*,*,#2197,.T.);
#3025=ORIENTED_EDGE('',*,*,#2198,.T.);
#3026=ORIENTED_EDGE('',*,*,#2197,.F.);
#3027=ORIENTED_EDGE('',*,*,#2192,.F.);
#3028=ORIENTED_EDGE('',*,*,#2199,.F.);
#3029=ORIENTED_EDGE('',*,*,#2189,.F.);
#3030=ORIENTED_EDGE('',*,*,#2196,.F.);
#3031=ORIENTED_EDGE('',*,*,#2198,.F.);
#3032=ORIENTED_EDGE('',*,*,#2191,.F.);
#3033=ORIENTED_EDGE('',*,*,#2186,.T.);
#3034=ORIENTED_EDGE('',*,*,#2190,.F.);
#3035=ORIENTED_EDGE('',*,*,#2199,.T.);
#3036=ORIENTED_EDGE('',*,*,#2200,.F.);
#3037=ORIENTED_EDGE('',*,*,#2169,.F.);
#3038=ORIENTED_EDGE('',*,*,#2168,.F.);
#3039=ORIENTED_EDGE('',*,*,#2167,.F.);
#3040=ORIENTED_EDGE('',*,*,#2166,.F.);
#3041=ORIENTED_EDGE('',*,*,#2165,.F.);
#3042=ORIENTED_EDGE('',*,*,#2164,.F.);
#3043=ORIENTED_EDGE('',*,*,#2163,.F.);
#3044=ORIENTED_EDGE('',*,*,#2162,.F.);
#3045=ORIENTED_EDGE('',*,*,#2201,.F.);
#3046=ORIENTED_EDGE('',*,*,#2202,.T.);
#3047=ORIENTED_EDGE('',*,*,#2142,.T.);
#3048=ORIENTED_EDGE('',*,*,#2146,.T.);
#3049=ORIENTED_EDGE('',*,*,#2149,.T.);
#3050=ORIENTED_EDGE('',*,*,#2152,.T.);
#3051=ORIENTED_EDGE('',*,*,#2155,.T.);
#3052=ORIENTED_EDGE('',*,*,#2158,.T.);
#3053=ORIENTED_EDGE('',*,*,#2180,.T.);
#3054=ORIENTED_EDGE('',*,*,#2203,.F.);
#3055=ORIENTED_EDGE('',*,*,#2204,.F.);
#3056=ORIENTED_EDGE('',*,*,#2178,.F.);
#3057=ORIENTED_EDGE('',*,*,#2159,.F.);
#3058=ORIENTED_EDGE('',*,*,#2156,.F.);
#3059=ORIENTED_EDGE('',*,*,#2153,.F.);
#3060=ORIENTED_EDGE('',*,*,#2150,.F.);
#3061=ORIENTED_EDGE('',*,*,#2147,.F.);
#3062=ORIENTED_EDGE('',*,*,#2144,.F.);
#3063=ORIENTED_EDGE('',*,*,#2205,.F.);
#3064=ORIENTED_EDGE('',*,*,#2160,.F.);
#3065=ORIENTED_EDGE('',*,*,#2177,.F.);
#3066=ORIENTED_EDGE('',*,*,#2176,.F.);
#3067=ORIENTED_EDGE('',*,*,#2175,.F.);
#3068=ORIENTED_EDGE('',*,*,#2174,.F.);
#3069=ORIENTED_EDGE('',*,*,#2173,.F.);
#3070=ORIENTED_EDGE('',*,*,#2172,.F.);
#3071=ORIENTED_EDGE('',*,*,#2171,.F.);
#3072=ORIENTED_EDGE('',*,*,#2200,.T.);
#3073=ORIENTED_EDGE('',*,*,#2179,.T.);
#3074=ORIENTED_EDGE('',*,*,#2204,.T.);
#3075=ORIENTED_EDGE('',*,*,#2203,.T.);
#3076=ORIENTED_EDGE('',*,*,#2170,.T.);
#3077=ORIENTED_EDGE('',*,*,#2195,.F.);
#3078=ORIENTED_EDGE('',*,*,#2201,.T.);
#3079=ORIENTED_EDGE('',*,*,#2161,.T.);
#3080=ORIENTED_EDGE('',*,*,#2205,.T.);
#3081=ORIENTED_EDGE('',*,*,#2143,.T.);
#3082=ORIENTED_EDGE('',*,*,#2202,.F.);
#4064=CYLINDRICAL_SURFACE('',#4558,3.22275);
#4065=CYLINDRICAL_SURFACE('',#4560,3.22275);
#4066=CYLINDRICAL_SURFACE('',#4561,3.22275);
#4067=CYLINDRICAL_SURFACE('',#4562,3.22275);
#4068=CYLINDRICAL_SURFACE('',#4563,3.22275);
#4069=CYLINDRICAL_SURFACE('',#4564,3.22275);
#4070=CYLINDRICAL_SURFACE('',#4565,3.933);
#4071=CYLINDRICAL_SURFACE('',#4568,3.22275);
#4072=CYLINDRICAL_SURFACE('',#4572,3.);
#4073=CYLINDRICAL_SURFACE('',#4576,24.5);
#4194=ADVANCED_FACE('',(#559),#4064,.T.);
#4195=ADVANCED_FACE('',(#560),#4065,.T.);
#4196=ADVANCED_FACE('',(#561),#4066,.T.);
#4197=ADVANCED_FACE('',(#562),#4067,.T.);
#4198=ADVANCED_FACE('',(#563),#4068,.T.);
#4199=ADVANCED_FACE('',(#564),#4069,.T.);
#4200=ADVANCED_FACE('',(#565),#4070,.T.);
#4201=ADVANCED_FACE('',(#566),#4071,.T.);
#4202=ADVANCED_FACE('',(#567),#47,.F.);
#4203=ADVANCED_FACE('',(#568),#135,.F.);
#4204=ADVANCED_FACE('',(#569),#4072,.T.);
#4205=ADVANCED_FACE('',(#570),#48,.F.);
#4206=ADVANCED_FACE('',(#571),#136,.T.);
#4207=ADVANCED_FACE('',(#572),#4073,.F.);
#4208=ADVANCED_FACE('',(#573),#49,.F.);
#4209=ADVANCED_FACE('',(#574),#50,.F.);
#4210=ADVANCED_FACE('',(#575,#100),#137,.F.);
#4211=ADVANCED_FACE('',(#576),#138,.T.);
#4386=CLOSED_SHELL('',(#4194,#4195,#4196,#4197,#4198,#4199,#4200,#4201,
#4202,#4203,#4204,#4205,#4206,#4207,#4208,#4209,#4210,#4211));
#4557=AXIS2_PLACEMENT_3D('',#13644,#5185,#5186);
#4558=AXIS2_PLACEMENT_3D('',#13645,#5187,#5188);
#4559=AXIS2_PLACEMENT_3D('',#13761,#5190,#5191);
#4560=AXIS2_PLACEMENT_3D('',#13844,#5192,#5193);
#4561=AXIS2_PLACEMENT_3D('',#14166,#5195,#5196);
#4562=AXIS2_PLACEMENT_3D('',#14488,#5198,#5199);
#4563=AXIS2_PLACEMENT_3D('',#14814,#5201,#5202);
#4564=AXIS2_PLACEMENT_3D('',#15134,#5204,#5205);
#4565=AXIS2_PLACEMENT_3D('',#15456,#5207,#5208);
#4566=AXIS2_PLACEMENT_3D('',#15466,#5209,#5210);
#4567=AXIS2_PLACEMENT_3D('',#16604,#5211,#5212);
#4568=AXIS2_PLACEMENT_3D('',#17899,#5213,#5214);
#4569=AXIS2_PLACEMENT_3D('',#18038,#5215,#5216);
#4570=AXIS2_PLACEMENT_3D('',#18232,#5218,#5219);
#4571=AXIS2_PLACEMENT_3D('',#18236,#5221,#5222);
#4572=AXIS2_PLACEMENT_3D('',#18238,#5224,#5225);
#4573=AXIS2_PLACEMENT_3D('',#18359,#5229,#5230);
#4574=AXIS2_PLACEMENT_3D('',#18441,#5232,#5233);
#4575=AXIS2_PLACEMENT_3D('',#18442,#5234,#5235);
#4576=AXIS2_PLACEMENT_3D('',#18443,#5236,#5237);
#4577=AXIS2_PLACEMENT_3D('',#19189,#5238,#5239);
#4578=AXIS2_PLACEMENT_3D('',#19190,#5240,#5241);
#5185=DIRECTION('axis',(0.,0.,1.));
#5186=DIRECTION('refdir',(1.,0.,0.));
#5187=DIRECTION('center_axis',(0.,0.,1.));
#5188=DIRECTION('ref_axis',(-0.70398889171803,0.71021098297451,0.));
#5189=DIRECTION('',(0.,0.,-1.));
#5190=DIRECTION('center_axis',(0.,0.,-1.));
#5191=DIRECTION('ref_axis',(-1.,-4.63459159752748E-15,0.));
#5192=DIRECTION('center_axis',(0.,0.,1.));
#5193=DIRECTION('ref_axis',(-0.70398889171803,0.71021098297451,0.));
#5194=DIRECTION('',(0.,0.,-1.));
#5195=DIRECTION('center_axis',(0.,0.,1.));
#5196=DIRECTION('ref_axis',(-0.70398889171803,0.71021098297451,0.));
#5197=DIRECTION('',(0.,0.,-1.));
#5198=DIRECTION('center_axis',(0.,0.,1.));
#5199=DIRECTION('ref_axis',(-0.70398889171803,0.71021098297451,0.));
#5200=DIRECTION('',(0.,0.,-1.));
#5201=DIRECTION('center_axis',(0.,0.,1.));
#5202=DIRECTION('ref_axis',(-0.70398889171803,0.71021098297451,0.));
#5203=DIRECTION('',(0.,0.,-1.));
#5204=DIRECTION('center_axis',(0.,0.,1.));
#5205=DIRECTION('ref_axis',(-0.70398889171803,0.71021098297451,0.));
#5206=DIRECTION('',(0.,0.,-1.));
#5207=DIRECTION('center_axis',(0.,0.,1.));
#5208=DIRECTION('ref_axis',(-1.,0.,0.));
#5209=DIRECTION('center_axis',(0.,0.,1.));
#5210=DIRECTION('ref_axis',(-1.,0.,0.));
#5211=DIRECTION('center_axis',(0.,0.,1.));
#5212=DIRECTION('ref_axis',(-1.,0.,0.));
#5213=DIRECTION('center_axis',(0.,0.,1.));
#5214=DIRECTION('ref_axis',(-0.70398889171803,0.71021098297451,0.));
#5215=DIRECTION('center_axis',(0.,0.,1.));
#5216=DIRECTION('ref_axis',(-1.,-4.63459159752748E-15,0.));
#5217=DIRECTION('',(-2.22044604925031E-16,1.,0.));
#5218=DIRECTION('center_axis',(-1.,-2.22044604925031E-16,0.));
#5219=DIRECTION('ref_axis',(-2.22044604925031E-16,1.,0.));
#5220=DIRECTION('',(0.,0.,1.));
#5221=DIRECTION('center_axis',(-1.,-2.22044604925031E-16,0.));
#5222=DIRECTION('ref_axis',(-2.22044604925031E-16,1.,0.));
#5223=DIRECTION('',(0.,0.,-1.));
#5224=DIRECTION('center_axis',(0.,0.,1.));
#5225=DIRECTION('ref_axis',(-1.,0.,0.));
#5226=DIRECTION('',(0.,0.,-1.));
#5227=DIRECTION('',(0.,0.,1.));
#5228=DIRECTION('',(0.,0.,-1.));
#5229=DIRECTION('center_axis',(0.,0.,1.));
#5230=DIRECTION('ref_axis',(-1.,0.,0.));
#5231=DIRECTION('',(2.22044604925031E-16,-1.,0.));
#5232=DIRECTION('center_axis',(-1.,-2.22044604925031E-16,0.));
#5233=DIRECTION('ref_axis',(-2.22044604925031E-16,1.,0.));
#5234=DIRECTION('center_axis',(1.,2.22044604925031E-16,0.));
#5235=DIRECTION('ref_axis',(-2.22044604925031E-16,1.,0.));
#5236=DIRECTION('center_axis',(1.,2.22044604925031E-16,0.));
#5237=DIRECTION('ref_axis',(-2.22044604925031E-16,1.,0.));
#5238=DIRECTION('center_axis',(0.,0.,-1.));
#5239=DIRECTION('ref_axis',(-1.,0.,0.));
#5240=DIRECTION('center_axis',(0.,0.,-1.));
#5241=DIRECTION('ref_axis',(-1.,0.,0.));
#13644=CARTESIAN_POINT('',(0.,0.,0.));
#13645=CARTESIAN_POINT('Origin',(0.,0.,-41.3107734492731));
#13646=CARTESIAN_POINT('',(2.26878001451759,-2.28883263001592,-38.0956657793148));
#13647=CARTESIAN_POINT('',(2.26878020134171,-2.28883244482855,-38.344825298285));
#13648=CARTESIAN_POINT('',(2.26878020078428,-2.2888324453811,-41.3107734492731));
#13649=CARTESIAN_POINT('',(1.84084363913124,2.64526222873462,-39.));
#13650=CARTESIAN_POINT('Ctrl Pts',(2.26878001451759,-2.28883263001592,-38.0956657793148));
#13651=CARTESIAN_POINT('Ctrl Pts',(2.17427930154028,-2.38250541593696,-38.1031821119126));
#13652=CARTESIAN_POINT('Ctrl Pts',(2.07398878675681,-2.47031457822959,-38.1107887399296));
#13653=CARTESIAN_POINT('Ctrl Pts',(1.91972359255967,-2.58931774641987,-38.122253635876));
#13654=CARTESIAN_POINT('Ctrl Pts',(1.869930754377,-2.62550248948013,-38.1259203852923));
#13655=CARTESIAN_POINT('Ctrl Pts',(1.78247137899517,-2.68530931588415,-38.1323246749032));
#13656=CARTESIAN_POINT('Ctrl Pts',(1.74529506510832,-2.70961900969796,-38.1350361091484));
#13657=CARTESIAN_POINT('Ctrl Pts',(1.66652723587141,-2.75883189158207,-38.1407651395205));
#13658=CARTESIAN_POINT('Ctrl Pts',(1.62485268027866,-2.78358039315739,-38.1437873718118));
#13659=CARTESIAN_POINT('Ctrl Pts',(1.50737368546323,-2.84980824849279,-38.152289114961));
#13660=CARTESIAN_POINT('Ctrl Pts',(1.43043989539902,-2.88919055487944,-38.1578375993854));
#13661=CARTESIAN_POINT('Ctrl Pts',(1.24367634917405,-2.97550547877898,-38.1712616004222));
#13662=CARTESIAN_POINT('Ctrl Pts',(1.13264029483711,-3.01951748271545,-38.1792092104411));
#13663=CARTESIAN_POINT('Ctrl Pts',(0.821702195093543,-3.12319787988501,
-38.2012225741584));
#13664=CARTESIAN_POINT('Ctrl Pts',(0.618038901880371,-3.16979441051984,
-38.2154007525052));
#13665=CARTESIAN_POINT('Ctrl Pts',(0.373706171312501,-3.20123374711232,
-38.2312996909552));
#13666=CARTESIAN_POINT('Ctrl Pts',(0.336033961644013,-3.20540719232247,
-38.2337192936363));
#13667=CARTESIAN_POINT('Ctrl Pts',(0.273065766336089,-3.21126060431635,
-38.2377013562446));
#13668=CARTESIAN_POINT('Ctrl Pts',(0.247808888654028,-3.21330834128441,
-38.2392816759083));
#13669=CARTESIAN_POINT('Ctrl Pts',(0.192163688630469,-3.21715978698585,
-38.2427243257972));
#13670=CARTESIAN_POINT('Ctrl Pts',(0.161769713007847,-3.21883126234038,
-38.2445800156828));
#13671=CARTESIAN_POINT('Ctrl Pts',(0.0639424290906524,-3.2228218988923,
-38.2504862289476));
#13672=CARTESIAN_POINT('Ctrl Pts',(-0.00354499632442759,-3.22345440752924,
-38.2544591921075));
#13673=CARTESIAN_POINT('Ctrl Pts',(-0.180335593062599,-3.21955823055032,
-38.2647129799248));
#13674=CARTESIAN_POINT('Ctrl Pts',(-0.289476570193864,-3.21158557147246,
-38.27089041191));
#13675=CARTESIAN_POINT('Ctrl Pts',(-0.610562095813819,-3.17162599647257,
-38.2891052733638));
#13676=CARTESIAN_POINT('Ctrl Pts',(-0.819933794119309,-3.12405146962742,
-38.3010735787721));
#13677=CARTESIAN_POINT('Ctrl Pts',(-1.08212018107994,-3.03628326866418,
-38.3173351951035));
#13678=CARTESIAN_POINT('Ctrl Pts',(-1.14061879793893,-3.01479488427622,
-38.3210459815119));
#13679=CARTESIAN_POINT('Ctrl Pts',(-1.23984078362437,-2.97504622312177,
-38.3275046740137));
#13680=CARTESIAN_POINT('Ctrl Pts',(-1.28087621313628,-2.9576106954346,-38.3302254250328));
#13681=CARTESIAN_POINT('Ctrl Pts',(-1.36560691285732,-2.91951541461419,
-38.3359541594752));
#13682=CARTESIAN_POINT('Ctrl Pts',(-1.40922533877395,-2.898712826262,-38.3389663623536));
#13683=CARTESIAN_POINT('Ctrl Pts',(-1.52838881523734,-2.83855581542678,
-38.3473783120707));
#13684=CARTESIAN_POINT('Ctrl Pts',(-1.60286243813911,-2.79717740831116,
-38.3528443328577));
#13685=CARTESIAN_POINT('Ctrl Pts',(-1.77510703048615,-2.69233749314807,
-38.3659908953008));
#13686=CARTESIAN_POINT('Ctrl Pts',(-1.87124496435387,-2.62642813890307,
-38.3737389737698));
#13687=CARTESIAN_POINT('Ctrl Pts',(-2.13061290652,-2.42713193467413,-38.3956945626229));
#13688=CARTESIAN_POINT('Ctrl Pts',(-2.2846508285143,-2.28273074097921,-38.4100357637933));
#13689=CARTESIAN_POINT('Ctrl Pts',(-2.44953378773206,-2.0946268219425,-38.4262100603979));
#13690=CARTESIAN_POINT('Ctrl Pts',(-2.47501979126649,-2.06445020581086,
-38.4287358608301));
#13691=CARTESIAN_POINT('Ctrl Pts',(-2.51586899692722,-2.01423866107835,
-38.4328169626678));
#13692=CARTESIAN_POINT('Ctrl Pts',(-2.53156252201413,-1.99447876822622,
-38.4343930553287));
#13693=CARTESIAN_POINT('Ctrl Pts',(-2.56488148344358,-1.95149944427592,
-38.4377543381736));
#13694=CARTESIAN_POINT('Ctrl Pts',(-2.58242682080637,-1.92822170973902,
-38.4395344840916));
#13695=CARTESIAN_POINT('Ctrl Pts',(-2.63534880786377,-1.85599075527485,
-38.4449464787116));
#13696=CARTESIAN_POINT('Ctrl Pts',(-2.66966885102523,-1.80627633665412,
-38.4485167828663));
#13697=CARTESIAN_POINT('Ctrl Pts',(-2.75236188219421,-1.67898026072075,
-38.457355493476));
#13698=CARTESIAN_POINT('Ctrl Pts',(-2.79887016946234,-1.60024941733983,
-38.4625516254117));
#13699=CARTESIAN_POINT('Ctrl Pts',(-2.96357549248282,-1.29222487473665,
-38.482258049921));
#13700=CARTESIAN_POINT('Ctrl Pts',(-3.05743459791969,-1.05105193063969,
-38.4965057754337));
#13701=CARTESIAN_POINT('Ctrl Pts',(-3.13556507642905,-0.74667707418331,
-38.5150730985969));
#13702=CARTESIAN_POINT('Ctrl Pts',(-3.14814455250686,-0.691722713896159,
-38.5184431351841));
#13703=CARTESIAN_POINT('Ctrl Pts',(-3.16790661457513,-0.593628696447907,
-38.5245056101752));
#13704=CARTESIAN_POINT('Ctrl Pts',(-3.17566463409302,-0.550618918493252,
-38.52717947519));
#13705=CARTESIAN_POINT('Ctrl Pts',(-3.19040727652036,-0.458161281488515,
-38.5329670697561));
#13706=CARTESIAN_POINT('Ctrl Pts',(-3.19712190130789,-0.408682593610614,
-38.536088398376));
#13707=CARTESIAN_POINT('Ctrl Pts',(-3.21348182352234,-0.262762107780036,
-38.5453712122579));
#13708=CARTESIAN_POINT('Ctrl Pts',(-3.21992891269857,-0.166024689612769,
-38.5516259899797));
#13709=CARTESIAN_POINT('Ctrl Pts',(-3.22513213349805,0.0764132141607757,
-38.5675420461662));
#13710=CARTESIAN_POINT('Ctrl Pts',(-3.21838798756779,0.222012007419459,
-38.577323546392));
#13711=CARTESIAN_POINT('Ctrl Pts',(-3.18400643390368,0.52225814946355,-38.5976867794836));
#13712=CARTESIAN_POINT('Ctrl Pts',(-3.15486494240396,0.676375973455781,
-38.6082464805641));
#13713=CARTESIAN_POINT('Ctrl Pts',(-3.10379610272837,0.868530916512614,
-38.6211444334022));
#13714=CARTESIAN_POINT('Ctrl Pts',(-3.09216399532717,0.909075578314394,
-38.6238495537467));
#13715=CARTESIAN_POINT('Ctrl Pts',(-3.07286290510045,0.971687147383015,
-38.6279894493481));
#13716=CARTESIAN_POINT('Ctrl Pts',(-3.06574461517715,0.993917707105095,
-38.6294518780201));
#13717=CARTESIAN_POINT('Ctrl Pts',(-3.04974423717555,1.04207906636557,-38.6326010065231));
#13718=CARTESIAN_POINT('Ctrl Pts',(-3.04077165134808,1.06797779819059,-38.6342825222027));
#13719=CARTESIAN_POINT('Ctrl Pts',(-3.01455442083262,1.14064157875144,-38.6389747727755));
#13720=CARTESIAN_POINT('Ctrl Pts',(-2.99655318293537,1.18712727360001,-38.6419464813996));
#13721=CARTESIAN_POINT('Ctrl Pts',(-2.9010718496155,1.41766451215537,-38.6566189025427));
#13722=CARTESIAN_POINT('Ctrl Pts',(-2.80767645097417,1.59466540573218,-38.6676942323365));
#13723=CARTESIAN_POINT('Ctrl Pts',(-2.61471693746718,1.89019917412492,-38.6875721856302));
#13724=CARTESIAN_POINT('Ctrl Pts',(-2.52190748015245,2.01235543870383,-38.6962748297064));
#13725=CARTESIAN_POINT('Ctrl Pts',(-2.37926698100997,2.17466280210837,-38.708978581507));
#13726=CARTESIAN_POINT('Ctrl Pts',(-2.33639660435145,2.22065751993029,-38.7127213559991));
#13727=CARTESIAN_POINT('Ctrl Pts',(-2.26075171756163,2.29719876128185,-38.7192227871496));
#13728=CARTESIAN_POINT('Ctrl Pts',(-2.22863445874217,2.32837037958883,-38.7219535599213));
#13729=CARTESIAN_POINT('Ctrl Pts',(-2.16052169967961,2.39177698215744,-38.7276911734426));
#13730=CARTESIAN_POINT('Ctrl Pts',(-2.12442968793483,2.42389134615721,-38.7307019823683));
#13731=CARTESIAN_POINT('Ctrl Pts',(-2.02315964388885,2.51000087189528,-38.7390769872662));
#13732=CARTESIAN_POINT('Ctrl Pts',(-1.95655899876813,2.56225568923481,-38.7445059190418));
#13733=CARTESIAN_POINT('Ctrl Pts',(-1.79446994891085,2.679423335291,-38.757537810221));
#13734=CARTESIAN_POINT('Ctrl Pts',(-1.69739993545653,2.74194488012524,-38.765206115763));
#13735=CARTESIAN_POINT('Ctrl Pts',(-1.41578970221266,2.90263306073517,-38.7869492357482));
#13736=CARTESIAN_POINT('Ctrl Pts',(-1.22474714851479,2.98826727907264,-38.80115617944));
#13737=CARTESIAN_POINT('Ctrl Pts',(-0.988108431002874,3.06780403406154,
-38.8173102259719));
#13738=CARTESIAN_POINT('Ctrl Pts',(-0.949216612935885,3.0800597444351,-38.8199193969883));
#13739=CARTESIAN_POINT('Ctrl Pts',(-0.885417164203674,3.09884108781853,
-38.8241141588516));
#13740=CARTESIAN_POINT('Ctrl Pts',(-0.860646447621111,3.10581189149313,
-38.82572186273));
#13741=CARTESIAN_POINT('Ctrl Pts',(-0.80685420215233,3.12025666910299,-38.8291655931871));
#13742=CARTESIAN_POINT('Ctrl Pts',(-0.77780753709691,3.12762385346042,-38.8309962483499));
#13743=CARTESIAN_POINT('Ctrl Pts',(-0.687972593484296,3.14907994088346,
-38.8365810976268));
#13744=CARTESIAN_POINT('Ctrl Pts',(-0.626871872190585,3.1618101498719,-38.8402717951017));
#13745=CARTESIAN_POINT('Ctrl Pts',(-0.470797425980772,3.18962510812534,
-38.8495130003313));
#13746=CARTESIAN_POINT('Ctrl Pts',(-0.375446345794052,3.20224927869193,
-38.8549865745452));
#13747=CARTESIAN_POINT('Ctrl Pts',(-0.0462376421054875,3.23092610076355,
-38.8736916624537));
#13748=CARTESIAN_POINT('Ctrl Pts',(0.1886962329817,3.22574130191479,-38.8867647878528));
#13749=CARTESIAN_POINT('Ctrl Pts',(0.479095622825629,3.18747865900904,-38.9040671818742));
#13750=CARTESIAN_POINT('Ctrl Pts',(0.536981939125614,3.17823891517948,-38.9075700890541));
#13751=CARTESIAN_POINT('Ctrl Pts',(0.638510243371634,3.15918026514406,-38.9138276720672));
#13752=CARTESIAN_POINT('Ctrl Pts',(0.682260731435794,3.15002147196495,-38.9165618329659));
#13753=CARTESIAN_POINT('Ctrl Pts',(0.77500019524035,3.12858462174404,-38.9224447898967));
#13754=CARTESIAN_POINT('Ctrl Pts',(0.823919025984935,3.1160590549255,-38.9256005523133));
#13755=CARTESIAN_POINT('Ctrl Pts',(0.965343684771793,3.07628454572699,-38.9348854227035));
#13756=CARTESIAN_POINT('Ctrl Pts',(1.05693958008847,3.04602870622226,-38.9411043850465));
#13757=CARTESIAN_POINT('Ctrl Pts',(1.39244536538294,2.91824874149358,-38.9646496396527));
#13758=CARTESIAN_POINT('Ctrl Pts',(1.62542595403343,2.7951718562419,-38.9826478213699));
#13759=CARTESIAN_POINT('Ctrl Pts',(1.84084363913124,2.64526222873462,-39.));
#13760=CARTESIAN_POINT('',(-1.87158653173895,2.62360084935064,-39.));
#13761=CARTESIAN_POINT('Origin',(0.,0.,-39.));
#13762=CARTESIAN_POINT('Ctrl Pts',(-1.87158653173894,2.62360084935064,-39.));
#13763=CARTESIAN_POINT('Ctrl Pts',(-1.89041153088413,2.61017174298758,-38.998572528826));
#13764=CARTESIAN_POINT('Ctrl Pts',(-1.90909197228119,2.59654004106516,-38.9971558584858));
#13765=CARTESIAN_POINT('Ctrl Pts',(-1.95205518984536,2.56447410407947,-38.9938937119439));
#13766=CARTESIAN_POINT('Ctrl Pts',(-1.97622658142679,2.54589385197734,-38.9920554271223));
#13767=CARTESIAN_POINT('Ctrl Pts',(-2.11761273738408,2.43398489791101,-38.9812640905256));
#13768=CARTESIAN_POINT('Ctrl Pts',(-2.22847532036539,2.33291030558068,-38.972638751804));
#13769=CARTESIAN_POINT('Ctrl Pts',(-2.45378047976953,2.09672449385349,-38.9538741497549));
#13770=CARTESIAN_POINT('Ctrl Pts',(-2.56494030377983,1.9591754907227,-38.943761890126));
#13771=CARTESIAN_POINT('Ctrl Pts',(-2.70202935873906,1.75774238346185,-38.9293276413066));
#13772=CARTESIAN_POINT('Ctrl Pts',(-2.73804212889853,1.70110124467118,-38.9253080656617));
#13773=CARTESIAN_POINT('Ctrl Pts',(-2.7972715271659,1.60118566111969,-38.9182533281895));
#13774=CARTESIAN_POINT('Ctrl Pts',(-2.82131635429567,1.55842779260394,-38.9152452891496));
#13775=CARTESIAN_POINT('Ctrl Pts',(-2.87032957175881,1.46641515134169,-38.9087844952294));
#13776=CARTESIAN_POINT('Ctrl Pts',(-2.89502646778123,1.41703438608332,-38.9053243733345));
#13777=CARTESIAN_POINT('Ctrl Pts',(-2.96365280279685,1.27052724868404,-38.8950659041947));
#13778=CARTESIAN_POINT('Ctrl Pts',(-3.00404362508528,1.17183427025286,-38.888162253539));
#13779=CARTESIAN_POINT('Ctrl Pts',(-3.11469824109349,0.857896153677981,
-38.8662091689328));
#13780=CARTESIAN_POINT('Ctrl Pts',(-3.16723264101671,0.637143388502542,
-38.8507362932036));
#13781=CARTESIAN_POINT('Ctrl Pts',(-3.20635666106965,0.334171303476188,
-38.8301398159638));
#13782=CARTESIAN_POINT('Ctrl Pts',(-3.21360260543384,0.255251114411016,
-38.8248382630747));
#13783=CARTESIAN_POINT('Ctrl Pts',(-3.22097521621672,0.120559799427511,
-38.8159668223204));
#13784=CARTESIAN_POINT('Ctrl Pts',(-3.22257723171047,0.0649060951656778,
-38.8123524644896));
#13785=CARTESIAN_POINT('Ctrl Pts',(-3.22281887525591,-0.0194166743170859,
-38.8069780507899));
#13786=CARTESIAN_POINT('Ctrl Pts',(-3.22251888196611,-0.0480697788259077,
-38.8051696340464));
#13787=CARTESIAN_POINT('Ctrl Pts',(-3.22124484231817,-0.101575361005251,
-38.801830260307));
#13788=CARTESIAN_POINT('Ctrl Pts',(-3.22036528638933,-0.126425308028545,
-38.8002950559868));
#13789=CARTESIAN_POINT('Ctrl Pts',(-3.2173435110204,-0.190734249366148,
-38.7963596350244));
#13790=CARTESIAN_POINT('Ctrl Pts',(-3.21476310027856,-0.230168102610655,
-38.7939823101881));
#13791=CARTESIAN_POINT('Ctrl Pts',(-3.19301600015096,-0.489269564107375,
-38.7785383714708));
#13792=CARTESIAN_POINT('Ctrl Pts',(-3.15207109455574,-0.706545733759861,
-38.7663900090102));
#13793=CARTESIAN_POINT('Ctrl Pts',(-3.05831375244858,-1.02207212315941,
-38.7478935118536));
#13794=CARTESIAN_POINT('Ctrl Pts',(-3.02213455571994,-1.12455109747725,
-38.7417495527388));
#13795=CARTESIAN_POINT('Ctrl Pts',(-2.95020911571181,-1.29957030206577,
-38.7308116176625));
#13796=CARTESIAN_POINT('Ctrl Pts',(-2.91678025577592,-1.37295601985905,
-38.7260825036295));
#13797=CARTESIAN_POINT('Ctrl Pts',(-2.85999748547326,-1.48615305518561,
-38.7185078126796));
#13798=CARTESIAN_POINT('Ctrl Pts',(-2.83847941782484,-1.52684995346584,
-38.7157255651867));
#13799=CARTESIAN_POINT('Ctrl Pts',(-2.79551671447219,-1.60405591198758,
-38.7103247828989));
#13800=CARTESIAN_POINT('Ctrl Pts',(-2.77420970383786,-1.64063076723599,
-38.7077116372666));
#13801=CARTESIAN_POINT('Ctrl Pts',(-2.72180549934165,-1.72664491662706,
-38.7014294811597));
#13802=CARTESIAN_POINT('Ctrl Pts',(-2.6900734781015,-1.77567784329784,-38.6977374421781));
#13803=CARTESIAN_POINT('Ctrl Pts',(-2.49035070894802,-2.06664368980951,
-38.675131534682));
#13804=CARTESIAN_POINT('Ctrl Pts',(-2.29119094673413,-2.2854414502584,-38.6549583088328));
#13805=CARTESIAN_POINT('Ctrl Pts',(-2.00881142332894,-2.52114717574195,
-38.6301828262148));
#13806=CARTESIAN_POINT('Ctrl Pts',(-1.95086142283051,-2.56625160460457,
-38.6252772206526));
#13807=CARTESIAN_POINT('Ctrl Pts',(-1.84932298700513,-2.63985324858534,
-38.6170417746014));
#13808=CARTESIAN_POINT('Ctrl Pts',(-1.80649232547213,-2.66934577441787,
-38.6136711242149));
#13809=CARTESIAN_POINT('Ctrl Pts',(-1.74045357961071,-2.71250106297437,
-38.6086503493814));
#13810=CARTESIAN_POINT('Ctrl Pts',(-1.71775850292413,-2.7269298816449,-38.6069555181186));
#13811=CARTESIAN_POINT('Ctrl Pts',(-1.67301805736663,-2.75459417412688,
-38.6036778302482));
#13812=CARTESIAN_POINT('Ctrl Pts',(-1.65099021493799,-2.76785294000404,
-38.6020931929567));
#13813=CARTESIAN_POINT('Ctrl Pts',(-1.59316223246176,-2.80172409973461,
-38.5980022509281));
#13814=CARTESIAN_POINT('Ctrl Pts',(-1.5571193099854,-2.82191488812873,-38.595520372194));
#13815=CARTESIAN_POINT('Ctrl Pts',(-1.33642960592855,-2.9400260537686,-38.580670697332));
#13816=CARTESIAN_POINT('Ctrl Pts',(-1.14298665592021,-3.02049626713358,
-38.5690793358358));
#13817=CARTESIAN_POINT('Ctrl Pts',(-0.831668191154774,-3.1157702891105,
-38.5507599418689));
#13818=CARTESIAN_POINT('Ctrl Pts',(-0.71847800015837,-3.14380083137577,
-38.5441690601075));
#13819=CARTESIAN_POINT('Ctrl Pts',(-0.520026841832245,-3.18166653884345,
-38.532487348396));
#13820=CARTESIAN_POINT('Ctrl Pts',(-0.435431101271444,-3.19434311466749,
-38.5274698152538));
#13821=CARTESIAN_POINT('Ctrl Pts',(-0.301967547722453,-3.20894226469868,
-38.5194351893927));
#13822=CARTESIAN_POINT('Ctrl Pts',(-0.253387136188485,-3.21314323354393,
-38.5164864377643));
#13823=CARTESIAN_POINT('Ctrl Pts',(-0.159628485629201,-3.21911150423433,
-38.5107399795707));
#13824=CARTESIAN_POINT('Ctrl Pts',(-0.114471451348873,-3.2210333903642,
-38.5079476311848));
#13825=CARTESIAN_POINT('Ctrl Pts',(-0.0157008584167212,-3.22315749462958,
-38.5017809707694));
#13826=CARTESIAN_POINT('Ctrl Pts',(0.0379066963205851,-3.22297274489809,
-38.4983959863226));
#13827=CARTESIAN_POINT('Ctrl Pts',(0.324041235736702,-3.21484713055911,
-38.4801171400821));
#13828=CARTESIAN_POINT('Ctrl Pts',(0.555171700199884,-3.18308015954396,
-38.4645356060155));
#13829=CARTESIAN_POINT('Ctrl Pts',(0.874788367132247,-3.10326305727819,
-38.442442416998));
#13830=CARTESIAN_POINT('Ctrl Pts',(0.96764531124071,-3.07557480588518,-38.4359661394279));
#13831=CARTESIAN_POINT('Ctrl Pts',(1.11831641141395,-3.02314650521573,-38.4254823938246));
#13832=CARTESIAN_POINT('Ctrl Pts',(1.17690569238394,-3.00082328775732,-38.421412607669));
#13833=CARTESIAN_POINT('Ctrl Pts',(1.26252884001002,-2.96530589042621,-38.4155107480571));
#13834=CARTESIAN_POINT('Ctrl Pts',(1.29008681005575,-2.95342077414907,-38.4136184429141));
#13835=CARTESIAN_POINT('Ctrl Pts',(1.34094489582743,-2.93063912210334,-38.4101449343738));
#13836=CARTESIAN_POINT('Ctrl Pts',(1.36428579455454,-2.9198464314739,-38.4085588540844));
#13837=CARTESIAN_POINT('Ctrl Pts',(1.42419223168782,-2.8912708217501,-38.4045046193086));
#13838=CARTESIAN_POINT('Ctrl Pts',(1.46055474404909,-2.87307338068009,-38.4020593485357));
#13839=CARTESIAN_POINT('Ctrl Pts',(1.68165533362765,-2.75714165121245,-38.3872298414131));
#13840=CARTESIAN_POINT('Ctrl Pts',(1.85688661530079,-2.64230687976265,-38.375621741074));
#13841=CARTESIAN_POINT('Ctrl Pts',(2.10657127239634,-2.44149166216285,-38.3575681122106));
#13842=CARTESIAN_POINT('Ctrl Pts',(2.1896836487191,-2.36723604007207,-38.3512617948146));
#13843=CARTESIAN_POINT('Ctrl Pts',(2.26878020134171,-2.28883244482855,-38.344825298285));
#13844=CARTESIAN_POINT('Origin',(0.,0.,-41.3107734492731));
#13845=CARTESIAN_POINT('',(2.26877996761345,-2.28883267650912,-36.8483014782414));
#13846=CARTESIAN_POINT('',(2.26878021215172,-2.28883243411325,-37.0933419659928));
#13847=CARTESIAN_POINT('',(2.26878020078428,-2.2888324453811,-41.3107734492731));
#13848=CARTESIAN_POINT('Ctrl Pts',(2.26877996761344,-2.28883267650913,-36.8483014782414));
#13849=CARTESIAN_POINT('Ctrl Pts',(2.22656546202223,-2.33067733628309,-36.8522391846632));
#13850=CARTESIAN_POINT('Ctrl Pts',(2.18317988826702,-2.37136742025256,-36.8561392081494));
#13851=CARTESIAN_POINT('Ctrl Pts',(2.11075868590298,-2.43561231691168,-36.8623833035587));
#13852=CARTESIAN_POINT('Ctrl Pts',(2.08241891546805,-2.45988644521745,-36.8647640214435));
#13853=CARTESIAN_POINT('Ctrl Pts',(2.03422178204832,-2.49973911779116,-36.8687003436139));
#13854=CARTESIAN_POINT('Ctrl Pts',(2.01459232639169,-2.51558578269246,-36.8702729882877));
#13855=CARTESIAN_POINT('Ctrl Pts',(1.97074503194305,-2.55014074084834,-36.8737172375388));
#13856=CARTESIAN_POINT('Ctrl Pts',(1.94644359286332,-2.56873729265205,-36.8755818053609));
#13857=CARTESIAN_POINT('Ctrl Pts',(1.86656824073359,-2.62807694755233,-36.8815809932148));
#13858=CARTESIAN_POINT('Ctrl Pts',(1.80994891970962,-2.66738667634847,-36.8856340353954));
#13859=CARTESIAN_POINT('Ctrl Pts',(1.65698097380178,-2.76647393784538,-36.8961889940548));
#13860=CARTESIAN_POINT('Ctrl Pts',(1.55866343852762,-2.82303646750421,-36.9025792107261));
#13861=CARTESIAN_POINT('Ctrl Pts',(1.27212214763379,-2.96834219976459,-36.9206475149131));
#13862=CARTESIAN_POINT('Ctrl Pts',(1.07802946847273,-3.04420666120054,-36.9322768815636));
#13863=CARTESIAN_POINT('Ctrl Pts',(0.817433353335214,-3.11799315220279,
-36.9481932970282));
#13864=CARTESIAN_POINT('Ctrl Pts',(0.75639125589621,-3.13336083025854,-36.951938746646));
#13865=CARTESIAN_POINT('Ctrl Pts',(0.65139547328786,-3.15654719577191,-36.9584326283996));
#13866=CARTESIAN_POINT('Ctrl Pts',(0.607656632736124,-3.16525818512124,
-36.9611527690314));
#13867=CARTESIAN_POINT('Ctrl Pts',(0.516559441526132,-3.18144329121965,
-36.9668556214862));
#13868=CARTESIAN_POINT('Ctrl Pts',(0.469187086298851,-3.18877377161861,
-36.9698420269909));
#13869=CARTESIAN_POINT('Ctrl Pts',(0.339146236760602,-3.20593610539624,
-36.9781031196637));
#13870=CARTESIAN_POINT('Ctrl Pts',(0.256237029098309,-3.21362523549382,
-36.9834403536453));
#13871=CARTESIAN_POINT('Ctrl Pts',(0.0608915632147329,-3.22413451724012,
-36.9961807350572));
#13872=CARTESIAN_POINT('Ctrl Pts',(-0.0515763266788825,-3.2242964598372,
-37.0036454861312));
#13873=CARTESIAN_POINT('Ctrl Pts',(-0.377242808422039,-3.2077211125975,
-37.0255118287511));
#13874=CARTESIAN_POINT('Ctrl Pts',(-0.589066298771854,-3.17565658689,-37.0400778136248));
#13875=CARTESIAN_POINT('Ctrl Pts',(-0.836336814109508,-3.11261581597723,
-37.0566133944375));
#13876=CARTESIAN_POINT('Ctrl Pts',(-0.876312396007306,-3.1015985284818,
-37.0592700731461));
#13877=CARTESIAN_POINT('Ctrl Pts',(-0.940583574594114,-3.08254343633048,
-37.0635026256295));
#13878=CARTESIAN_POINT('Ctrl Pts',(-0.965014841209167,-3.07498260518654,
-37.0651022753642));
#13879=CARTESIAN_POINT('Ctrl Pts',(-1.01659581645663,-3.05834428457822,
-37.0684566605088));
#13880=CARTESIAN_POINT('Ctrl Pts',(-1.04371917407903,-3.04919452269436,
-37.0702075178538));
#13881=CARTESIAN_POINT('Ctrl Pts',(-1.12417147106392,-3.02085548280124,
-37.0753718167645));
#13882=CARTESIAN_POINT('Ctrl Pts',(-1.17712226169957,-3.00061882444818,
-37.0787324587866));
#13883=CARTESIAN_POINT('Ctrl Pts',(-1.30598297217461,-2.94743438703454,
-37.0868784798277));
#13884=CARTESIAN_POINT('Ctrl Pts',(-1.38121164644181,-2.91293954888571,
-37.0916061304529));
#13885=CARTESIAN_POINT('Ctrl Pts',(-1.69144739912402,-2.75596172690494,
-37.1112983327154));
#13886=CARTESIAN_POINT('Ctrl Pts',(-1.91219153594532,-2.60764988758928,
-37.1258917416526));
#13887=CARTESIAN_POINT('Ctrl Pts',(-2.15721263353127,-2.39501325979633,
-37.1450212180986));
#13888=CARTESIAN_POINT('Ctrl Pts',(-2.20104154479816,-2.35479730056485,
-37.1485710324401));
#13889=CARTESIAN_POINT('Ctrl Pts',(-2.27542291640106,-2.28265575892519,
-37.1548423691386));
#13890=CARTESIAN_POINT('Ctrl Pts',(-2.30647877449684,-2.25127122588317,
-37.1575409291374));
#13891=CARTESIAN_POINT('Ctrl Pts',(-2.37085500912079,-2.18348309534915,
-37.1633142658819));
#13892=CARTESIAN_POINT('Ctrl Pts',(-2.40400336629703,-2.14693253240028,
-37.1663952099519));
#13893=CARTESIAN_POINT('Ctrl Pts',(-2.49644478741192,-2.04017725659565,
-37.1753111672561));
#13894=CARTESIAN_POINT('Ctrl Pts',(-2.55358829565566,-1.96818294426044,
-37.1812270680578));
#13895=CARTESIAN_POINT('Ctrl Pts',(-2.68530530037351,-1.78682661140694,
-37.1958965725635));
#13896=CARTESIAN_POINT('Ctrl Pts',(-2.75636778853909,-1.67512559756117,
-37.2047440612377));
#13897=CARTESIAN_POINT('Ctrl Pts',(-2.90792107484353,-1.40102032046565,
-37.2258238768182));
#13898=CARTESIAN_POINT('Ctrl Pts',(-2.98199181887782,-1.23555487708316,
-37.238074921831));
#13899=CARTESIAN_POINT('Ctrl Pts',(-3.05523282257704,-1.02631719928974,
-37.252428709054));
#13900=CARTESIAN_POINT('Ctrl Pts',(-3.06795312656356,-0.987642927626157,
-37.2550352577364));
#13901=CARTESIAN_POINT('Ctrl Pts',(-3.08743004550622,-0.924413857459189,
-37.2592103671183));
#13902=CARTESIAN_POINT('Ctrl Pts',(-3.09463422985292,-0.900002454551657,
-37.2608015267464));
#13903=CARTESIAN_POINT('Ctrl Pts',(-3.10939766023268,-0.847701861001912,
-37.2641633380954));
#13904=CARTESIAN_POINT('Ctrl Pts',(-3.11687240680839,-0.819791919985914,
-37.2659296063928));
#13905=CARTESIAN_POINT('Ctrl Pts',(-3.13827826839333,-0.735335445456807,
-37.2712013590898));
#13906=CARTESIAN_POINT('Ctrl Pts',(-3.15105372240961,-0.678505717752124,
-37.2746506684513));
#13907=CARTESIAN_POINT('Ctrl Pts',(-3.17891307704552,-0.536720748012749,
-37.2830834212154));
#13908=CARTESIAN_POINT('Ctrl Pts',(-3.19213968603264,-0.451445793672037,
-37.2880036293125));
#13909=CARTESIAN_POINT('Ctrl Pts',(-3.23087576436145,-0.112323534104255,
-37.3073099808694));
#13910=CARTESIAN_POINT('Ctrl Pts',(-3.22963530472755,0.143613498771788,
-37.3213889182298));
#13911=CARTESIAN_POINT('Ctrl Pts',(-3.19071554804759,0.45736858803147,-37.3400006676139));
#13912=CARTESIAN_POINT('Ctrl Pts',(-3.1814701780575,0.517782327082446,-37.3436427334051));
#13913=CARTESIAN_POINT('Ctrl Pts',(-3.16256191119151,0.62151918679783,-37.3500179182935));
#13914=CARTESIAN_POINT('Ctrl Pts',(-3.15371106808167,0.664973792715772,
-37.3527255770841));
#13915=CARTESIAN_POINT('Ctrl Pts',(-3.13328502681066,0.755648800556685,
-37.3584601315694));
#13916=CARTESIAN_POINT('Ctrl Pts',(-3.1215323300654,0.80281734008179,-37.361491949208));
#13917=CARTESIAN_POINT('Ctrl Pts',(-3.08569003217087,0.933950180492215,
-37.3700643226131));
#13918=CARTESIAN_POINT('Ctrl Pts',(-3.05924860296201,1.01722254567061,-37.3756758970466));
#13919=CARTESIAN_POINT('Ctrl Pts',(-2.98802080924565,1.21351041314089,-37.3893079125053));
#13920=CARTESIAN_POINT('Ctrl Pts',(-2.94016050826175,1.3252652804794,-37.3974039158715));
#13921=CARTESIAN_POINT('Ctrl Pts',(-2.79541636473548,1.61657255940743,-37.419261693474));
#13922=CARTESIAN_POINT('Ctrl Pts',(-2.6876070469541,1.7900941156866,-37.4331167519453));
#13923=CARTESIAN_POINT('Ctrl Pts',(-2.54086284320336,1.98282830846227,-37.4487612471043));
#13924=CARTESIAN_POINT('Ctrl Pts',(-2.51705578706488,2.0129636235733,-37.4512143910582));
#13925=CARTESIAN_POINT('Ctrl Pts',(-2.47664069178851,2.06228309955132,-37.4552313417631));
#13926=CARTESIAN_POINT('Ctrl Pts',(-2.46033516072461,2.08170885608321,-37.4568138685713));
#13927=CARTESIAN_POINT('Ctrl Pts',(-2.4242346770514,2.12370068041981,-37.4602332901854));
#13928=CARTESIAN_POINT('Ctrl Pts',(-2.40435103968709,2.14618605423676,-37.4620641605057));
#13929=CARTESIAN_POINT('Ctrl Pts',(-2.34037455674722,2.21652846608821,-37.4678035365746));
#13930=CARTESIAN_POINT('Ctrl Pts',(-2.29514289246163,2.26333200410626,-37.471640077336));
#13931=CARTESIAN_POINT('Ctrl Pts',(-2.17477526409264,2.38056029568585,-37.4813957823589));
#13932=CARTESIAN_POINT('Ctrl Pts',(-2.09762540973359,2.44881289968059,-37.487223094372));
#13933=CARTESIAN_POINT('Ctrl Pts',(-1.8388721672032,2.6565084350534,-37.5059091950354));
#13934=CARTESIAN_POINT('Ctrl Pts',(-1.64567290055719,2.78033087841417,-37.5186475156818));
#13935=CARTESIAN_POINT('Ctrl Pts',(-1.38660072774091,2.90983746461253,-37.5357030378488));
#13936=CARTESIAN_POINT('Ctrl Pts',(-1.33145051273807,2.93548198566862,-37.5393283976233));
#13937=CARTESIAN_POINT('Ctrl Pts',(-1.23491971576535,2.97708820394792,-37.5456848044145));
#13938=CARTESIAN_POINT('Ctrl Pts',(-1.19387337201152,2.9937847208708,-37.5483908505492));
#13939=CARTESIAN_POINT('Ctrl Pts',(-1.10698457413611,3.02705762747664,-37.5541322270884));
#13940=CARTESIAN_POINT('Ctrl Pts',(-1.06108439000323,3.04345071288269,-37.5571726978799));
#13941=CARTESIAN_POINT('Ctrl Pts',(-0.931197344000002,3.08654398550227,
-37.5658041048123));
#13942=CARTESIAN_POINT('Ctrl Pts',(-0.846466550857527,3.11084785851076,
-37.5714676993067));
#13943=CARTESIAN_POINT('Ctrl Pts',(-0.64106341765264,3.16075175310816,-37.5852732810637));
#13944=CARTESIAN_POINT('Ctrl Pts',(-0.519712022346255,3.18295605398513,
-37.5934937229118));
#13945=CARTESIAN_POINT('Ctrl Pts',(-0.19912849305455,3.22279106802224,-37.6152079394678));
#13946=CARTESIAN_POINT('Ctrl Pts',(0.0010100672380102,3.22893827289216,
-37.6287794571775));
#13947=CARTESIAN_POINT('Ctrl Pts',(0.239210334686556,3.21409476085178,-37.6442006335225));
#13948=CARTESIAN_POINT('Ctrl Pts',(0.277938100015091,3.21097764456997,-37.6466835403259));
#13949=CARTESIAN_POINT('Ctrl Pts',(0.341906645307251,3.2046628492782,-37.6507343620222));
#13950=CARTESIAN_POINT('Ctrl Pts',(0.367181967903874,3.20186534735771,-37.6523216745831));
#13951=CARTESIAN_POINT('Ctrl Pts',(0.422023658344153,3.19513738894977,-37.6557345600265));
#13952=CARTESIAN_POINT('Ctrl Pts',(0.451572968407502,3.19109525181101,-37.6575544676143));
#13953=CARTESIAN_POINT('Ctrl Pts',(0.544151207460026,3.17711942422927,-37.6632083345519));
#13954=CARTESIAN_POINT('Ctrl Pts',(0.606946870924651,3.16572344993154,-37.6669734338793));
#13955=CARTESIAN_POINT('Ctrl Pts',(0.766878093718888,3.13176510842158,-37.6764754408824));
#13956=CARTESIAN_POINT('Ctrl Pts',(0.863381578175057,3.10654615806019,-37.6821264776748));
#13957=CARTESIAN_POINT('Ctrl Pts',(1.18383383824032,3.00671351396365,-37.701042629767));
#13958=CARTESIAN_POINT('Ctrl Pts',(1.4006954226164,2.91201514955137,-37.7141566257034));
#13959=CARTESIAN_POINT('Ctrl Pts',(1.65721649088791,2.76465902735695,-37.7315932656678));
#13960=CARTESIAN_POINT('Ctrl Pts',(1.70831540366137,2.73337956605624,-37.7351674005065));
#13961=CARTESIAN_POINT('Ctrl Pts',(1.79555896916883,2.67657244486789,-37.7414666677254));
#13962=CARTESIAN_POINT('Ctrl Pts',(1.83210537742337,2.65169033956436,-37.7441682072329));
#13963=CARTESIAN_POINT('Ctrl Pts',(1.9081861862424,2.59756806694281,-37.7499328752155));
#13964=CARTESIAN_POINT('Ctrl Pts',(1.94758614415828,2.56815929828049,-37.7530018489588));
#13965=CARTESIAN_POINT('Ctrl Pts',(2.05772358588289,2.4819585511367,-37.7618293980166));
#13966=CARTESIAN_POINT('Ctrl Pts',(2.1267529474346,2.42306914216833,-37.7676662136421));
#13967=CARTESIAN_POINT('Ctrl Pts',(2.28799626571639,2.27330776958204,-37.7820595395862));
#13968=CARTESIAN_POINT('Ctrl Pts',(2.37739572758953,2.17964220445891,-37.7907047886177));
#13969=CARTESIAN_POINT('Ctrl Pts',(2.58145336776289,1.9383150342948,-37.8119672389101));
#13970=CARTESIAN_POINT('Ctrl Pts',(2.68938145637623,1.78555382187953,-37.8246189284822));
#13971=CARTESIAN_POINT('Ctrl Pts',(2.80377266717897,1.58952737727943,-37.8393071831893));
#13972=CARTESIAN_POINT('Ctrl Pts',(2.82341196639628,1.55437564829835,-37.841884019212));
#13973=CARTESIAN_POINT('Ctrl Pts',(2.85434878912896,1.49648073382498,-37.8460250691588));
#13974=CARTESIAN_POINT('Ctrl Pts',(2.86604503278857,1.47395645639384,-37.8476111927161));
#13975=CARTESIAN_POINT('Ctrl Pts',(2.89055298824072,1.42536464879731,-37.8509768166654));
#13976=CARTESIAN_POINT('Ctrl Pts',(2.90328055141569,1.39925806745773,-37.852751638427));
#13977=CARTESIAN_POINT('Ctrl Pts',(2.94086659208732,1.31944063753356,-37.8580876884661));
#13978=CARTESIAN_POINT('Ctrl Pts',(2.96460126551952,1.2652115024049,-37.8615906009248));
#13979=CARTESIAN_POINT('Ctrl Pts',(3.02005082158743,1.12837704823534,-37.8702000133257));
#13980=CARTESIAN_POINT('Ctrl Pts',(3.04988390963164,1.04506053216023,-37.8752396878314));
#13981=CARTESIAN_POINT('Ctrl Pts',(3.15053554888574,0.722736983060389,-37.8943235197578));
#13982=CARTESIAN_POINT('Ctrl Pts',(3.1969720521322,0.477060361114301,-37.9080953797963));
#13983=CARTESIAN_POINT('Ctrl Pts',(3.2190412275143,0.166567907088179,-37.926401410525));
#13984=CARTESIAN_POINT('Ctrl Pts',(3.22165222442586,0.104534703803008,-37.9300981335659));
#13985=CARTESIAN_POINT('Ctrl Pts',(3.22305591521284,-0.00197835242181084,
-37.9365343329445));
#13986=CARTESIAN_POINT('Ctrl Pts',(3.22272203532739,-0.0464298595534938,
-37.939246806003));
#13987=CARTESIAN_POINT('Ctrl Pts',(3.2201106075036,-0.139020218365842,-37.9449583445058));
#13988=CARTESIAN_POINT('Ctrl Pts',(3.21767245203043,-0.18714312022975,-37.9479616256255));
#13989=CARTESIAN_POINT('Ctrl Pts',(3.20796289165827,-0.319835277845849,
-37.9563453308025));
#13990=CARTESIAN_POINT('Ctrl Pts',(3.19842851436289,-0.40419492256789,-37.9617916941235));
#13991=CARTESIAN_POINT('Ctrl Pts',(3.16801459310315,-0.602701299123028,
-37.9748836704233));
#13992=CARTESIAN_POINT('Ctrl Pts',(3.14427935947758,-0.716288347962332,
-37.9825962776455));
#13993=CARTESIAN_POINT('Ctrl Pts',(3.06068975381992,-1.03057642115649,-38.0044246240833));
#13994=CARTESIAN_POINT('Ctrl Pts',(2.9873309965288,-1.22709855207136,-38.0186739640594));
#13995=CARTESIAN_POINT('Ctrl Pts',(2.87766210121168,-1.45148762481557,-38.034841967959));
#13996=CARTESIAN_POINT('Ctrl Pts',(2.85920660834066,-1.4875124890563,-38.0374329869506));
#13997=CARTESIAN_POINT('Ctrl Pts',(2.828070157859,-1.5455685217396,-38.0415897612611));
#13998=CARTESIAN_POINT('Ctrl Pts',(2.81579896211066,-1.56781352432736,-38.0431777700064));
#13999=CARTESIAN_POINT('Ctrl Pts',(2.78897719051659,-1.61510450283525,-38.046540640982));
#14000=CARTESIAN_POINT('Ctrl Pts',(2.77434984684862,-1.64010346937344,-38.04831097003));
#14001=CARTESIAN_POINT('Ctrl Pts',(2.72909016981954,-1.7151162292903,-38.0536110953751));
#14002=CARTESIAN_POINT('Ctrl Pts',(2.69742649943247,-1.76449652722705,-38.0570838083759));
#14003=CARTESIAN_POINT('Ctrl Pts',(2.61538227873249,-1.88507158489489,-38.0655922661487));
#14004=CARTESIAN_POINT('Ctrl Pts',(2.56342602756872,-1.95513885638657,-38.0705632772635));
#14005=CARTESIAN_POINT('Ctrl Pts',(2.43364121459208,-2.11608163164715,-38.0822536746435));
#14006=CARTESIAN_POINT('Ctrl Pts',(2.35353954212797,-2.20481568628638,-38.088924234407));
#14007=CARTESIAN_POINT('Ctrl Pts',(2.26878001451759,-2.28883263001591,-38.0956657793148));
#14008=CARTESIAN_POINT('Ctrl Pts',(2.26878020134171,-2.28883244482855,-38.344825298285));
#14009=CARTESIAN_POINT('Ctrl Pts',(2.27165473796579,-2.2859830917466,-38.3445913823381));
#14010=CARTESIAN_POINT('Ctrl Pts',(2.27452397086319,-2.2831282600329,-38.3443572989667));
#14011=CARTESIAN_POINT('Ctrl Pts',(2.33728119711145,-2.22045029895543,-38.3392240548976));
#14012=CARTESIAN_POINT('Ctrl Pts',(2.39479059336495,-2.15830009166445,-38.3342536326079));
#14013=CARTESIAN_POINT('Ctrl Pts',(2.48117376581954,-2.05723801477477,-38.3262930186285));
#14014=CARTESIAN_POINT('Ctrl Pts',(2.51173240763389,-2.01981470641953,-38.3233698719877));
#14015=CARTESIAN_POINT('Ctrl Pts',(2.56895635862974,-1.94642842073486,-38.3176751722873));
#14016=CARTESIAN_POINT('Ctrl Pts',(2.5957362913412,-1.9105688069594,-38.3149089432171));
#14017=CARTESIAN_POINT('Ctrl Pts',(2.65831344742135,-1.82302992032227,-38.3081891338843));
#14018=CARTESIAN_POINT('Ctrl Pts',(2.6933610757823,-1.77083984024132,-38.3042092848356));
#14019=CARTESIAN_POINT('Ctrl Pts',(2.8084074537765,-1.58819891998019,-38.2903617376354));
#14020=CARTESIAN_POINT('Ctrl Pts',(2.88062399551668,-1.45310837738793,-38.2802432098167));
#14021=CARTESIAN_POINT('Ctrl Pts',(3.02443360285753,-1.13087431368775,-38.2565738867371));
#14022=CARTESIAN_POINT('Ctrl Pts',(3.08874124059288,-0.94114693343855,-38.2429612400691));
#14023=CARTESIAN_POINT('Ctrl Pts',(3.14661130301666,-0.698170179423578,
-38.2266496987288));
#14024=CARTESIAN_POINT('Ctrl Pts',(3.15703825191403,-0.649395378250362,
-38.2234317481557));
#14025=CARTESIAN_POINT('Ctrl Pts',(3.17143641476915,-0.573463212716543,
-38.2185282831025));
#14026=CARTESIAN_POINT('Ctrl Pts',(3.17619965662134,-0.546465783410158,
-38.216805500934));
#14027=CARTESIAN_POINT('Ctrl Pts',(3.18437954695069,-0.496376033402855,
-38.2136512529005));
#14028=CARTESIAN_POINT('Ctrl Pts',(3.18789081486779,-0.47330166209682,-38.2122148635845));
#14029=CARTESIAN_POINT('Ctrl Pts',(3.19704019465122,-0.408446798069404,
-38.2082192915786));
#14030=CARTESIAN_POINT('Ctrl Pts',(3.20210985605113,-0.366589191315778,
-38.2056888441778));
#14031=CARTESIAN_POINT('Ctrl Pts',(3.22210160425585,-0.169138840918346,
-38.1939290625036));
#14032=CARTESIAN_POINT('Ctrl Pts',(3.22651440091117,-0.0126808017563364,
-38.1851190847756));
#14033=CARTESIAN_POINT('Ctrl Pts',(3.21306128460206,0.289168827813927,-38.1681348769976));
#14034=CARTESIAN_POINT('Ctrl Pts',(3.19668896002065,0.434233744232097,-38.1599758637728));
#14035=CARTESIAN_POINT('Ctrl Pts',(3.15316504134073,0.673108926160731,-38.1460328667813));
#14036=CARTESIAN_POINT('Ctrl Pts',(3.13148095010002,0.767691412365471,-38.1403778406849));
#14037=CARTESIAN_POINT('Ctrl Pts',(3.09222195982493,0.909271679335177,-38.131616180453));
#14038=CARTESIAN_POINT('Ctrl Pts',(3.07776113113975,0.957077660267318,-38.128605585575));
#14039=CARTESIAN_POINT('Ctrl Pts',(3.04857486485327,1.04604899943607,-38.1228939317893));
#14040=CARTESIAN_POINT('Ctrl Pts',(3.03411118073422,1.08728849400791,-38.1202018145761));
#14041=CARTESIAN_POINT('Ctrl Pts',(2.99908732392589,1.18100296592571,-38.1139755340226));
#14042=CARTESIAN_POINT('Ctrl Pts',(2.97798073577599,1.23325702772943,-38.1104242587957));
#14043=CARTESIAN_POINT('Ctrl Pts',(2.85262327461581,1.52159681219223,-38.0903663194394));
#14044=CARTESIAN_POINT('Ctrl Pts',(2.7216890709309,1.74501638187759,-38.0729606187827));
#14045=CARTESIAN_POINT('Ctrl Pts',(2.5102820556353,2.02310252600544,-38.0494496077613));
#14046=CARTESIAN_POINT('Ctrl Pts',(2.45193721640244,2.09343384765107,-38.0433298838923));
#14047=CARTESIAN_POINT('Ctrl Pts',(2.35019718567448,2.20597714833772,-38.0333455934372));
#14048=CARTESIAN_POINT('Ctrl Pts',(2.30846019730029,2.24961651861663,-38.0294222082498));
#14049=CARTESIAN_POINT('Ctrl Pts',(2.24479241847086,2.31254705214783,-38.0237178621356));
#14050=CARTESIAN_POINT('Ctrl Pts',(2.22378780579074,2.33275262487673,-38.0218788319707));
#14051=CARTESIAN_POINT('Ctrl Pts',(2.18408947651563,2.36991719229273,-38.0184869689903));
#14052=CARTESIAN_POINT('Ctrl Pts',(2.16546596637975,2.38694606527149,-38.0169295276647));
#14053=CARTESIAN_POINT('Ctrl Pts',(2.11717928420632,2.43006789568504,-38.0129722320241));
#14054=CARTESIAN_POINT('Ctrl Pts',(2.08723188216769,2.4558382441225,-38.0105940023849));
#14055=CARTESIAN_POINT('Ctrl Pts',(1.90741400056747,2.60490901225448,-37.996705216883));
#14056=CARTESIAN_POINT('Ctrl Pts',(1.74711244564422,2.71503104984654,-37.9858786194218));
#14057=CARTESIAN_POINT('Ctrl Pts',(1.46796802255642,2.87177146020033,-37.9678804646102));
#14058=CARTESIAN_POINT('Ctrl Pts',(1.35455454523371,2.92697473963885,-37.9607782171537));
#14059=CARTESIAN_POINT('Ctrl Pts',(1.15570854589672,3.0097241715196,-37.9483547195677));
#14060=CARTESIAN_POINT('Ctrl Pts',(1.07182567112627,3.04060679029611,-37.9431233706838));
#14061=CARTESIAN_POINT('Ctrl Pts',(0.940123047463643,3.08296732769151,-37.9348543001324));
#14062=CARTESIAN_POINT('Ctrl Pts',(0.893139190966295,3.09690504992285,-37.9318940797336));
#14063=CARTESIAN_POINT('Ctrl Pts',(0.803052859161704,3.12140857221847,-37.9261892204013));
#14064=CARTESIAN_POINT('Ctrl Pts',(0.760013997471235,3.13216599044381,-37.9234513557489));
#14065=CARTESIAN_POINT('Ctrl Pts',(0.657686482147988,3.15550921112142,-37.9169071005329));
#14066=CARTESIAN_POINT('Ctrl Pts',(0.598239500672287,3.16731726001198,-37.9130777288064));
#14067=CARTESIAN_POINT('Ctrl Pts',(0.312020075524238,3.21582438418708,-37.8944976847947));
#14068=CARTESIAN_POINT('Ctrl Pts',(0.0821172869127146,3.22987774663927,
-37.8790812014648));
#14069=CARTESIAN_POINT('Ctrl Pts',(-0.249118151567528,3.21472381895837,
-37.8567654922359));
#14070=CARTESIAN_POINT('Ctrl Pts',(-0.350676446671104,3.2052358492194,-37.8499206341811));
#14071=CARTESIAN_POINT('Ctrl Pts',(-0.51566289264444,3.18188517695293,-37.8389357872099));
#14072=CARTESIAN_POINT('Ctrl Pts',(-0.579425121929288,3.17089406489248,
-37.8347245081003));
#14073=CARTESIAN_POINT('Ctrl Pts',(-0.672221685925151,3.15200507709747,
-37.8286844756345));
#14074=CARTESIAN_POINT('Ctrl Pts',(-0.701542258503872,3.14560910070194,
-37.8267892111906));
#14075=CARTESIAN_POINT('Ctrl Pts',(-0.755555731291702,3.13303378668247,
-37.8233274876798));
#14076=CARTESIAN_POINT('Ctrl Pts',(-0.780270237289268,3.12697034897802,
-37.8217557123886));
#14077=CARTESIAN_POINT('Ctrl Pts',(-0.842426723475524,3.110938076983,-37.8178294684548));
#14078=CARTESIAN_POINT('Ctrl Pts',(-0.879765219573846,3.10058574433759,
-37.815495039914));
#14079=CARTESIAN_POINT('Ctrl Pts',(-1.10940055459906,3.0324353491069,-37.8012372224427));
#14080=CARTESIAN_POINT('Ctrl Pts',(-1.29615333912781,2.95743778531122,-37.7900550043966));
#14081=CARTESIAN_POINT('Ctrl Pts',(-1.58386467065014,2.80936935740552,-37.7718567513543));
#14082=CARTESIAN_POINT('Ctrl Pts',(-1.68970081467572,2.74701517829149,-37.7649309759927));
#14083=CARTESIAN_POINT('Ctrl Pts',(-1.86476915145129,2.62991963582593,-37.7527718483158));
#14084=CARTESIAN_POINT('Ctrl Pts',(-1.93578556139886,2.57809497685447,-37.7476227465077));
#14085=CARTESIAN_POINT('Ctrl Pts',(-2.04273006991471,2.49313935566136,-37.7394557677428));
#14086=CARTESIAN_POINT('Ctrl Pts',(-2.08017502740776,2.46198323741499,-37.736512301795));
#14087=CARTESIAN_POINT('Ctrl Pts',(-2.1503292694726,2.40086805639257,-37.7308250287658));
#14088=CARTESIAN_POINT('Ctrl Pts',(-2.18315446071986,2.37105876993493,-37.7280876212882));
#14089=CARTESIAN_POINT('Ctrl Pts',(-2.25961185074089,2.29869213355574,-37.7215212625154));
#14090=CARTESIAN_POINT('Ctrl Pts',(-2.30267103764056,2.25555681683872,-37.7176686810892));
#14091=CARTESIAN_POINT('Ctrl Pts',(-2.5204886100954,2.02461338064273,-37.6973396820467));
#14092=CARTESIAN_POINT('Ctrl Pts',(-2.67356470774371,1.81767279471486,-37.6800049339823));
#14093=CARTESIAN_POINT('Ctrl Pts',(-2.84296091881277,1.520218010426,-37.6570025041703));
#14094=CARTESIAN_POINT('Ctrl Pts',(-2.88245381252503,1.44393594396125,-37.6512637040534));
#14095=CARTESIAN_POINT('Ctrl Pts',(-2.9434697895925,1.31357332854842,-37.64180917393));
#14096=CARTESIAN_POINT('Ctrl Pts',(-2.96666074642067,1.26032304650454,-37.6380419089829));
#14097=CARTESIAN_POINT('Ctrl Pts',(-2.9992062980479,1.17970850993814,-37.632507870223));
#14098=CARTESIAN_POINT('Ctrl Pts',(-3.00965160544775,1.15280004331367,-37.630688281417));
#14099=CARTESIAN_POINT('Ctrl Pts',(-3.02862287431501,1.10191130135672,-37.6273035930529));
#14100=CARTESIAN_POINT('Ctrl Pts',(-3.03722863417711,1.07796441786877,-37.6257345581336));
#14101=CARTESIAN_POINT('Ctrl Pts',(-3.05887059356578,1.01542473126594,-37.6216930730648));
#14102=CARTESIAN_POINT('Ctrl Pts',(-3.07146080753454,0.976680879071006,
-37.619244202684));
#14103=CARTESIAN_POINT('Ctrl Pts',(-3.13576063457448,0.765253878824999,
-37.6061245389506));
#14104=CARTESIAN_POINT('Ctrl Pts',(-3.17365247230519,0.588686371692925,
-37.5960306659801));
#14105=CARTESIAN_POINT('Ctrl Pts',(-3.21345246228294,0.278279245276633,
-37.5784425206236));
#14106=CARTESIAN_POINT('Ctrl Pts',(-3.22218255573067,0.145785185533111,
-37.5709850725669));
#14107=CARTESIAN_POINT('Ctrl Pts',(-3.22309832160539,-0.0788896773562119,
-37.5580454959396));
#14108=CARTESIAN_POINT('Ctrl Pts',(-3.21953156783552,-0.170882403457803,
-37.5526655478121));
#14109=CARTESIAN_POINT('Ctrl Pts',(-3.20801406649237,-0.311765193062044,
-37.5442235958648));
#14110=CARTESIAN_POINT('Ctrl Pts',(-3.20286548072224,-0.360838060283908,
-37.5412453473283));
#14111=CARTESIAN_POINT('Ctrl Pts',(-3.19098467755158,-0.453519194078132,
-37.535539155528));
#14112=CARTESIAN_POINT('Ctrl Pts',(-3.18447940253439,-0.497145360915337,
-37.5328187782859));
#14113=CARTESIAN_POINT('Ctrl Pts',(-3.1671265731411,-0.599122854422057,
-37.5263731989797));
#14114=CARTESIAN_POINT('Ctrl Pts',(-3.15555869138312,-0.657333666120761,
-37.5226266992922));
#14115=CARTESIAN_POINT('Ctrl Pts',(-3.08905306072559,-0.949545461999719,
-37.5034658351552));
#14116=CARTESIAN_POINT('Ctrl Pts',(-3.00967224895398,-1.17716791912406,
-37.4873036305016));
#14117=CARTESIAN_POINT('Ctrl Pts',(-2.8633944082986,-1.48212104540801,-37.4645354758524));
#14118=CARTESIAN_POINT('Ctrl Pts',(-2.81702941848359,-1.56845697060663,
-37.4579631907309));
#14119=CARTESIAN_POINT('Ctrl Pts',(-2.73444297117563,-1.70672832789192,
-37.4473512783489));
#14120=CARTESIAN_POINT('Ctrl Pts',(-2.70049699380034,-1.75994801506134,
-37.4432450221919));
#14121=CARTESIAN_POINT('Ctrl Pts',(-2.64831334313962,-1.83669145117825,
-37.4373274845656));
#14122=CARTESIAN_POINT('Ctrl Pts',(-2.63127964940723,-1.86101225332141,
-37.4354527676264));
#14123=CARTESIAN_POINT('Ctrl Pts',(-2.59902664965847,-1.9057349229102,-37.4320116797367));
#14124=CARTESIAN_POINT('Ctrl Pts',(-2.58389874989663,-1.92619635664796,
-37.4304403967975));
#14125=CARTESIAN_POINT('Ctrl Pts',(-2.54495411727566,-1.97758681487464,
-37.4264974566633));
#14126=CARTESIAN_POINT('Ctrl Pts',(-2.52081508416879,-2.00826608877016,
-37.4241463904307));
#14127=CARTESIAN_POINT('Ctrl Pts',(-2.3707921899393,-2.1919676012109,-37.4100348518224));
#14128=CARTESIAN_POINT('Ctrl Pts',(-2.23156057411662,-2.33356644108525,
-37.3989932589583));
#14129=CARTESIAN_POINT('Ctrl Pts',(-1.98545025213148,-2.54155279390823,
-37.3808751831953));
#14130=CARTESIAN_POINT('Ctrl Pts',(-1.88617116396231,-2.61607709750948,
-37.3738802891545));
#14131=CARTESIAN_POINT('Ctrl Pts',(-1.70916031291056,-2.73362637923154,
-37.3616180156489));
#14132=CARTESIAN_POINT('Ctrl Pts',(-1.63349357892053,-2.77950337699727,
-37.3564371575791));
#14133=CARTESIAN_POINT('Ctrl Pts',(-1.51330441669205,-2.84577033926732,
-37.3482320588409));
#14134=CARTESIAN_POINT('Ctrl Pts',(-1.47004101513924,-2.86835808676202,
-37.3452834965974));
#14135=CARTESIAN_POINT('Ctrl Pts',(-1.38654949681861,-2.90956377465475,
-37.3395931763765));
#14136=CARTESIAN_POINT('Ctrl Pts',(-1.34641731772463,-2.92835123774248,
-37.336857982385));
#14137=CARTESIAN_POINT('Ctrl Pts',(-1.25040069938937,-2.97090938185656,
-37.3303082532387));
#14138=CARTESIAN_POINT('Ctrl Pts',(-1.19420821932128,-2.99393894765704,
-37.3264704241723));
#14139=CARTESIAN_POINT('Ctrl Pts',(-0.922691703143771,-3.09635546071641,
-37.3078923355994));
#14140=CARTESIAN_POINT('Ctrl Pts',(-0.699973903237812,-3.15416932650819,
-37.2924866311282));
#14141=CARTESIAN_POINT('Ctrl Pts',(-0.371595256884859,-3.20289767077732,
-37.2701339895035));
#14142=CARTESIAN_POINT('Ctrl Pts',(-0.269478967605364,-3.21310120746428,
-37.2632435857226));
#14143=CARTESIAN_POINT('Ctrl Pts',(-0.102211660402182,-3.22178292120925,
-37.2521973768242));
#14144=CARTESIAN_POINT('Ctrl Pts',(-0.037285516713679,-3.22318838502173,
-37.2479690811891));
#14145=CARTESIAN_POINT('Ctrl Pts',(0.057640407328837,-3.22237413426154,
-37.2419130170813));
#14146=CARTESIAN_POINT('Ctrl Pts',(0.0876341397706829,-3.22169798233136,
-37.2400179163342));
#14147=CARTESIAN_POINT('Ctrl Pts',(0.142977769507828,-3.21967685214438,
-37.2365604018247));
#14148=CARTESIAN_POINT('Ctrl Pts',(0.16832679075914,-3.21845114938461,-37.2349925782557));
#14149=CARTESIAN_POINT('Ctrl Pts',(0.232072714007886,-3.21461360458662,
-37.2310857203621));
#14150=CARTESIAN_POINT('Ctrl Pts',(0.270441858641376,-3.21161328055527,
-37.2287663813698));
#14151=CARTESIAN_POINT('Ctrl Pts',(0.510892767642874,-3.18847085508226,
-37.2143835673812));
#14152=CARTESIAN_POINT('Ctrl Pts',(0.710767523240319,-3.14995015062899,
-37.2030822114829));
#14153=CARTESIAN_POINT('Ctrl Pts',(1.02258776042949,-3.05863780125785,-37.1848089044967));
#14154=CARTESIAN_POINT('Ctrl Pts',(1.13743272318657,-3.01781303086743,-37.1779349305185));
#14155=CARTESIAN_POINT('Ctrl Pts',(1.33031802021586,-2.93666877169308,-37.1658523433417));
#14156=CARTESIAN_POINT('Ctrl Pts',(1.40952906066172,-2.89948194125591,-37.1607264147894));
#14157=CARTESIAN_POINT('Ctrl Pts',(1.53026951546676,-2.836680768831,-37.1525878490591));
#14158=CARTESIAN_POINT('Ctrl Pts',(1.57289841346733,-2.81326727797083,-37.1496487849099));
#14159=CARTESIAN_POINT('Ctrl Pts',(1.65335182683059,-2.76667877970481,-37.1439656231952));
#14160=CARTESIAN_POINT('Ctrl Pts',(1.69125979135601,-2.74366975961099,-37.1412278169675));
#14161=CARTESIAN_POINT('Ctrl Pts',(1.78021565882626,-2.68713204233637,-37.1346530707924));
#14162=CARTESIAN_POINT('Ctrl Pts',(1.83080742514473,-2.65292099259234,-37.1307922927997));
#14163=CARTESIAN_POINT('Ctrl Pts',(2.01842830872305,-2.5181248694824,-37.1159967540171));
#14164=CARTESIAN_POINT('Ctrl Pts',(2.14828130876245,-2.40827565919211,-37.1047397524462));
#14165=CARTESIAN_POINT('Ctrl Pts',(2.26878021215176,-2.28883243411322,-37.0933419659928));
#14166=CARTESIAN_POINT('Origin',(0.,0.,-41.3107734492731));
#14167=CARTESIAN_POINT('',(2.26878020052865,-2.28883244563449,-35.5935118781384));
#14168=CARTESIAN_POINT('',(2.26878031087686,-2.28883233625302,-35.8411988517434));
#14169=CARTESIAN_POINT('',(2.26878020078428,-2.2888324453811,-41.3107734492731));
#14170=CARTESIAN_POINT('Ctrl Pts',(2.26878020052865,-2.28883244563449,-35.5935118781384));
#14171=CARTESIAN_POINT('Ctrl Pts',(2.26354090144405,-2.29402584371414,-35.5939651056608));
#14172=CARTESIAN_POINT('Ctrl Pts',(2.25828373912089,-2.29920128299245,-35.5944191016049));
#14173=CARTESIAN_POINT('Ctrl Pts',(2.21867188016905,-2.33793043921428,-35.5978341633605));
#14174=CARTESIAN_POINT('Ctrl Pts',(2.18359041128584,-2.37072903991118,-35.6008265966311));
#14175=CARTESIAN_POINT('Ctrl Pts',(2.08533156771503,-2.4585622132953,-35.6091284325938));
#14176=CARTESIAN_POINT('Ctrl Pts',(2.02072402227752,-2.51193319617988,-35.614501462253));
#14177=CARTESIAN_POINT('Ctrl Pts',(1.86381843778374,-2.63157606181455,-35.6273559894686));
#14178=CARTESIAN_POINT('Ctrl Pts',(1.76995242735959,-2.69560321212375,-35.6349007857385));
#14179=CARTESIAN_POINT('Ctrl Pts',(1.49276364673534,-2.86394782860756,-35.6566541046229));
#14180=CARTESIAN_POINT('Ctrl Pts',(1.30231380304113,-2.95542318951066,-35.6710132350367));
#14181=CARTESIAN_POINT('Ctrl Pts',(1.06492003862431,-3.04200905587315,-35.6873951051703));
#14182=CARTESIAN_POINT('Ctrl Pts',(1.02527125238563,-3.05560027112643,-35.6900815707981));
#14183=CARTESIAN_POINT('Ctrl Pts',(0.963128167203858,-3.07555641233828,
-35.6942037504232));
#14184=CARTESIAN_POINT('Ctrl Pts',(0.940811702225469,-3.08245625379665,
-35.6956665444774));
#14185=CARTESIAN_POINT('Ctrl Pts',(0.892043499132521,-3.09695547891241,
-35.6988222243865));
#14186=CARTESIAN_POINT('Ctrl Pts',(0.865565458393363,-3.10445992109168,
-35.7005097615375));
#14187=CARTESIAN_POINT('Ctrl Pts',(0.7901364035587,-3.12479800629861,-35.7052525540808));
#14188=CARTESIAN_POINT('Ctrl Pts',(0.740972936182149,-3.13681969877855,
-35.7082672403231));
#14189=CARTESIAN_POINT('Ctrl Pts',(0.623315263681643,-3.16266904611618,
-35.715344096899));
#14190=CARTESIAN_POINT('Ctrl Pts',(0.554613593254188,-3.1754373207095,-35.7193667605599));
#14191=CARTESIAN_POINT('Ctrl Pts',(0.354464290981182,-3.20594052595851,
-35.7309037114525));
#14192=CARTESIAN_POINT('Ctrl Pts',(0.222269848251562,-3.21780941008953,
-35.7383024390774));
#14193=CARTESIAN_POINT('Ctrl Pts',(-0.0581403100300363,-3.22561872952891,
-35.7541104422919));
#14194=CARTESIAN_POINT('Ctrl Pts',(-0.206094044542116,-3.21955218789992,
-35.7625220916176));
#14195=CARTESIAN_POINT('Ctrl Pts',(-0.415109772789401,-3.19651267891872,
-35.7748860055901));
#14196=CARTESIAN_POINT('Ctrl Pts',(-0.476904236459283,-3.1878787676546,
-35.778600272211));
#14197=CARTESIAN_POINT('Ctrl Pts',(-0.582298553132052,-3.17002015577549,
-35.7850582445273));
#14198=CARTESIAN_POINT('Ctrl Pts',(-0.626030075138798,-3.16167446764726,
-35.7877745208966));
#14199=CARTESIAN_POINT('Ctrl Pts',(-0.716648593786405,-3.14242715613542,
-35.7934861806598));
#14200=CARTESIAN_POINT('Ctrl Pts',(-0.763492081499223,-3.13137559102172,
-35.7964856151189));
#14201=CARTESIAN_POINT('Ctrl Pts',(-0.891759464810913,-3.09806489205968,
-35.8048349783755));
#14202=CARTESIAN_POINT('Ctrl Pts',(-0.972579014633753,-3.07365077547407,
-35.8102498045939));
#14203=CARTESIAN_POINT('Ctrl Pts',(-1.16095434485393,-3.00857227787655,
-35.8232384370307));
#14204=CARTESIAN_POINT('Ctrl Pts',(-1.26747417942642,-2.96527027270289,
-35.8308775671399));
#14205=CARTESIAN_POINT('Ctrl Pts',(-1.55796622961292,-2.82866426343408,
-35.8524171422834));
#14206=CARTESIAN_POINT('Ctrl Pts',(-1.73564626281591,-2.72325891450911,
-35.8664501191032));
#14207=CARTESIAN_POINT('Ctrl Pts',(-1.93682175994712,-2.57617831349985,
-35.8826250535428));
#14208=CARTESIAN_POINT('Ctrl Pts',(-1.97108524325117,-2.55005815578797,
-35.8853894518258));
#14209=CARTESIAN_POINT('Ctrl Pts',(-2.02324996571201,-2.50861145630289,
-35.8896004995417));
#14210=CARTESIAN_POINT('Ctrl Pts',(-2.04152314618931,-2.49376325965712,
-35.8910760734246));
#14211=CARTESIAN_POINT('Ctrl Pts',(-2.08054793985152,-2.46133648896671,
-35.8942253632126));
#14212=CARTESIAN_POINT('Ctrl Pts',(-2.10124322674253,-2.44369271025123,
-35.8958943009146));
#14213=CARTESIAN_POINT('Ctrl Pts',(-2.15850879656005,-2.39360543380923,
-35.9005170867573));
#14214=CARTESIAN_POINT('Ctrl Pts',(-2.19456919951827,-2.36058759056946,
-35.9034335846283));
#14215=CARTESIAN_POINT('Ctrl Pts',(-2.27783208525988,-2.28079204148107,
-35.9102197763547));
#14216=CARTESIAN_POINT('Ctrl Pts',(-2.32436735996572,-2.23334919300036,
-35.9140543068686));
#14217=CARTESIAN_POINT('Ctrl Pts',(-2.52351336619857,-2.0173466082862,-35.9308299985919));
#14218=CARTESIAN_POINT('Ctrl Pts',(-2.65950097101085,-1.83435707226531,
-35.9433333446844));
#14219=CARTESIAN_POINT('Ctrl Pts',(-2.82328562500885,-1.55697045956263,
-35.9618602949035));
#14220=CARTESIAN_POINT('Ctrl Pts',(-2.86784359159268,-1.4732853251386,-35.967393536816));
#14221=CARTESIAN_POINT('Ctrl Pts',(-2.93008660238295,-1.34282866866419,
-35.9760204010245));
#14222=CARTESIAN_POINT('Ctrl Pts',(-2.9504806285277,-1.29740509821388,-35.9790239820137));
#14223=CARTESIAN_POINT('Ctrl Pts',(-2.98692010291811,-1.21093612069053,
-35.9847513708787));
#14224=CARTESIAN_POINT('Ctrl Pts',(-3.00319191667718,-1.16999829316909,
-35.9874669183777));
#14225=CARTESIAN_POINT('Ctrl Pts',(-3.03913559849512,-1.07387327498605,
-35.9938581341467));
#14226=CARTESIAN_POINT('Ctrl Pts',(-3.05815131467147,-1.01845905122748,
-35.997553915797));
#14227=CARTESIAN_POINT('Ctrl Pts',(-3.13436292744262,-0.774941887613437,
-36.013854970905));
#14228=CARTESIAN_POINT('Ctrl Pts',(-3.17578194538343,-0.582370067358845,
-36.0269346893612));
#14229=CARTESIAN_POINT('Ctrl Pts',(-3.22113441339815,-0.207678306326374,
-36.0523363672066));
#14230=CARTESIAN_POINT('Ctrl Pts',(-3.22771416946683,-0.026581414062457,
-36.0645824543539));
#14231=CARTESIAN_POINT('Ctrl Pts',(-3.21711584209016,0.194783298034463,
-36.0789319368598));
#14232=CARTESIAN_POINT('Ctrl Pts',(-3.21439855691865,0.235408448348466,
-36.081538718959));
#14233=CARTESIAN_POINT('Ctrl Pts',(-3.20873265899732,0.301330420113932,
-36.0857141027372));
#14234=CARTESIAN_POINT('Ctrl Pts',(-3.20625283717842,0.326662229438198,
-36.087305308439));
#14235=CARTESIAN_POINT('Ctrl Pts',(-3.20031757435715,0.3806832538367,-36.0906672383803));
#14236=CARTESIAN_POINT('Ctrl Pts',(-3.19677600772745,0.409360001350443,
-36.0924335792214));
#14237=CARTESIAN_POINT('Ctrl Pts',(-3.18493514338627,0.49567796082553,-36.0977053171184));
#14238=CARTESIAN_POINT('Ctrl Pts',(-3.17545846841295,0.553148160072557,
-36.1011545492486));
#14239=CARTESIAN_POINT('Ctrl Pts',(-3.14809473551754,0.695022387610974,
-36.1095869599579));
#14240=CARTESIAN_POINT('Ctrl Pts',(-3.12836642481632,0.779026098282429,
-36.1145069189186));
#14241=CARTESIAN_POINT('Ctrl Pts',(-3.03705563323056,1.10791259091326,-36.1338134750345));
#14242=CARTESIAN_POINT('Ctrl Pts',(-2.93989136922043,1.34469707506539,-36.1478928416227));
#14243=CARTESIAN_POINT('Ctrl Pts',(-2.78610860079051,1.62094126662066,-36.1665050202827));
#14244=CARTESIAN_POINT('Ctrl Pts',(-2.75487467292528,1.6734743977719,-36.1701471075011));
#14245=CARTESIAN_POINT('Ctrl Pts',(-2.69842956222401,1.76254421451183,-36.1765225081536));
#14246=CARTESIAN_POINT('Ctrl Pts',(-2.67392169209843,1.79950734901087,-36.1792303670357));
#14247=CARTESIAN_POINT('Ctrl Pts',(-2.62096552875842,1.87590525363985,-36.1849655544831));
#14248=CARTESIAN_POINT('Ctrl Pts',(-2.59237201101042,1.91522525571623,-36.1879978097528));
#14249=CARTESIAN_POINT('Ctrl Pts',(-2.50993334790275,2.02335981279647,-36.1965722591115));
#14250=CARTESIAN_POINT('Ctrl Pts',(-2.45416635020851,2.09064958200223,-36.2021855155395));
#14251=CARTESIAN_POINT('Ctrl Pts',(-2.31444534459754,2.24593679900908,-36.2158229478985));
#14252=CARTESIAN_POINT('Ctrl Pts',(-2.22811187230057,2.33160949522023,-36.2239227649028));
#14253=CARTESIAN_POINT('Ctrl Pts',(-1.98469415084609,2.54727223292994,-36.2457756443501));
#14254=CARTESIAN_POINT('Ctrl Pts',(-1.81976548560901,2.66759617722323,-36.2596214630228));
#14255=CARTESIAN_POINT('Ctrl Pts',(-1.61153798554035,2.79115363381581,-36.2752587787306));
#14256=CARTESIAN_POINT('Ctrl Pts',(-1.57815156720587,2.81016569152845,-36.2777129437919));
#14257=CARTESIAN_POINT('Ctrl Pts',(-1.5221699285708,2.84073222909436,-36.2817311405092));
#14258=CARTESIAN_POINT('Ctrl Pts',(-1.49976472430271,2.85262455054892,-36.2833139129441));
#14259=CARTESIAN_POINT('Ctrl Pts',(-1.45054739343048,2.87800806875332,-36.2867334176054));
#14260=CARTESIAN_POINT('Ctrl Pts',(-1.42368340388327,2.89139134360469,-36.2885641342824));
#14261=CARTESIAN_POINT('Ctrl Pts',(-1.33801520572887,2.93258653390383,-36.2943019864602));
#14262=CARTESIAN_POINT('Ctrl Pts',(-1.278551101498,2.95899589389115,-36.2981372201688));
#14263=CARTESIAN_POINT('Ctrl Pts',(-1.12307554049099,3.02248308835779,-36.3078883725895));
#14264=CARTESIAN_POINT('Ctrl Pts',(-1.02601350786151,3.05679590004349,-36.3137125568083));
#14265=CARTESIAN_POINT('Ctrl Pts',(-0.708237972260232,3.15228809390823,
-36.3323998912176));
#14266=CARTESIAN_POINT('Ctrl Pts',(-0.482627985629584,3.19461776418244,
-36.3451421882252));
#14267=CARTESIAN_POINT('Ctrl Pts',(-0.193837355632865,3.21748982242873,
-36.3622013383093));
#14268=CARTESIAN_POINT('Ctrl Pts',(-0.133110872217195,3.22057362616077,
-36.3658257830755));
#14269=CARTESIAN_POINT('Ctrl Pts',(-0.0280403261118533,3.22293258004212,
-36.3721811356575));
#14270=CARTESIAN_POINT('Ctrl Pts',(0.0162695635558281,3.22301344731505,
-36.3748870676241));
#14271=CARTESIAN_POINT('Ctrl Pts',(0.109299029638245,3.22126482714555,-36.3806287578051));
#14272=CARTESIAN_POINT('Ctrl Pts',(0.158003353452588,3.21924337409048,-36.3836696682562));
#14273=CARTESIAN_POINT('Ctrl Pts',(0.294618091048819,3.2104656425767,-36.3923041652124));
#14274=CARTESIAN_POINT('Ctrl Pts',(0.382318988508141,3.20120592937546,-36.3979705006071));
#14275=CARTESIAN_POINT('Ctrl Pts',(0.591572778784733,3.17039084675088,-36.4117850715972));
#14276=CARTESIAN_POINT('Ctrl Pts',(0.712479943286171,3.14542599256789,-36.4200119174888));
#14277=CARTESIAN_POINT('Ctrl Pts',(1.02450433014471,3.06208337111606,-36.441720909037));
#14278=CARTESIAN_POINT('Ctrl Pts',(1.21216502597076,2.99276270421163,-36.4552801299156));
#14279=CARTESIAN_POINT('Ctrl Pts',(1.42726638373711,2.88972989686238,-36.4706915708696));
#14280=CARTESIAN_POINT('Ctrl Pts',(1.46201480193291,2.87230590845259,-36.4731757721629));
#14281=CARTESIAN_POINT('Ctrl Pts',(1.51895972856227,2.84245059308457,-36.4772277656719));
#14282=CARTESIAN_POINT('Ctrl Pts',(1.54133870739029,2.83037792334745,-36.4788149951191));
#14283=CARTESIAN_POINT('Ctrl Pts',(1.58962559705208,2.80358620626423,-36.4822260193326));
#14284=CARTESIAN_POINT('Ctrl Pts',(1.61547618744904,2.78877069542717,-36.4840441848412));
#14285=CARTESIAN_POINT('Ctrl Pts',(1.69591130173054,2.74117780055491,-36.4896881486924));
#14286=CARTESIAN_POINT('Ctrl Pts',(1.74973495249272,2.70713862986431,-36.4934453713537));
#14287=CARTESIAN_POINT('Ctrl Pts',(1.88486629158105,2.61596347736303,-36.5029198393972));
#14288=CARTESIAN_POINT('Ctrl Pts',(1.96460586562053,2.55662115101025,-36.5085517749056));
#14289=CARTESIAN_POINT('Ctrl Pts',(2.22479866420522,2.3436118923492,-36.5275029417947));
#14290=CARTESIAN_POINT('Ctrl Pts',(2.39099481993979,2.1737940910071,-36.5406669302415));
#14291=CARTESIAN_POINT('Ctrl Pts',(2.57394562628078,1.94023102217013,-36.5581552824553));
#14292=CARTESIAN_POINT('Ctrl Pts',(2.6094965878973,1.89214677089969,-36.5617229272965));
#14293=CARTESIAN_POINT('Ctrl Pts',(2.66895747794847,1.806858000927,-36.5680141628378));
#14294=CARTESIAN_POINT('Ctrl Pts',(2.69347782595103,1.77009795282878,-36.5707143100193));
#14295=CARTESIAN_POINT('Ctrl Pts',(2.74368098157445,1.69137563538036,-36.5764792659022));
#14296=CARTESIAN_POINT('Ctrl Pts',(2.76917404639804,1.6493063860622,-36.5795499883659));
#14297=CARTESIAN_POINT('Ctrl Pts',(2.83902330206339,1.52785197110619,-36.5883937027893));
#14298=CARTESIAN_POINT('Ctrl Pts',(2.88099351072359,1.44715544802375,-36.5942454597321));
#14299=CARTESIAN_POINT('Ctrl Pts',(2.97451804017407,1.24709347451989,-36.6086916588234));
#14300=CARTESIAN_POINT('Ctrl Pts',(3.02236999044531,1.1261770577313,-36.6173758456667));
#14301=CARTESIAN_POINT('Ctrl Pts',(3.12050857877369,0.826411934281973,-36.6385985929753));
#14302=CARTESIAN_POINT('Ctrl Pts',(3.16289990345324,0.645447927472846,-36.6511683208497));
#14303=CARTESIAN_POINT('Ctrl Pts',(3.19527156673198,0.42188450113924,-36.665789298792));
#14304=CARTESIAN_POINT('Ctrl Pts',(3.20030532758923,0.38182858154707,-36.6683731381609));
#14305=CARTESIAN_POINT('Ctrl Pts',(3.20727806948035,0.316433148956264,-36.6725223378304));
#14306=CARTESIAN_POINT('Ctrl Pts',(3.20967224437507,0.291147394506173,-36.6741097649234));
#14307=CARTESIAN_POINT('Ctrl Pts',(3.21416154468152,0.236908320488248,-36.6774757767755));
#14308=CARTESIAN_POINT('Ctrl Pts',(3.21616491157962,0.207950447403865,-36.6792497342344));
#14309=CARTESIAN_POINT('Ctrl Pts',(3.22105371632892,0.120051725813268,-36.6845748383974));
#14310=CARTESIAN_POINT('Ctrl Pts',(3.22271204948684,0.0610524349901548,
-36.6880681142143));
#14311=CARTESIAN_POINT('Ctrl Pts',(3.22280501060443,-0.0860024722208844,
-36.6966449989047));
#14312=CARTESIAN_POINT('Ctrl Pts',(3.21925300262627,-0.174012354868599,
-36.7016625240194));
#14313=CARTESIAN_POINT('Ctrl Pts',(3.19177948652545,-0.511131051920171,
-36.720782694854));
#14314=CARTESIAN_POINT('Ctrl Pts',(3.14249326600938,-0.757259053267211,
-36.7346073127618));
#14315=CARTESIAN_POINT('Ctrl Pts',(3.04611802014202,-1.05409483015323,-36.7529653371432));
#14316=CARTESIAN_POINT('Ctrl Pts',(3.02530655092486,-1.11241649105303,-36.756652989525));
#14317=CARTESIAN_POINT('Ctrl Pts',(2.98668945696848,-1.21151959429912,-36.7630803984826));
#14318=CARTESIAN_POINT('Ctrl Pts',(2.96969504595494,-1.25259916821432,-36.7657934563463));
#14319=CARTESIAN_POINT('Ctrl Pts',(2.93247480316839,-1.33755065939312,-36.7715131782093));
#14320=CARTESIAN_POINT('Ctrl Pts',(2.91210142483516,-1.38134540825479,-36.774524207285));
#14321=CARTESIAN_POINT('Ctrl Pts',(2.85298125850654,-1.50130475331785,-36.7829527395469));
#14322=CARTESIAN_POINT('Ctrl Pts',(2.81218007840505,-1.57640704471713,-36.7884372819794));
#14323=CARTESIAN_POINT('Ctrl Pts',(2.70844608590889,-1.75047838560856,-36.8016515477586));
#14324=CARTESIAN_POINT('Ctrl Pts',(2.64300243359661,-1.84780659276855,-36.8094500858079));
#14325=CARTESIAN_POINT('Ctrl Pts',(2.47958917365417,-2.06433946078963,-36.8276623645477));
#14326=CARTESIAN_POINT('Ctrl Pts',(2.37811192243085,-2.18045859068994,-36.8381031557792));
#14327=CARTESIAN_POINT('Ctrl Pts',(2.26877996761344,-2.28883267650913,-36.8483014782414));
#14328=CARTESIAN_POINT('Ctrl Pts',(2.26878021215176,-2.28883243411322,-37.0933419659928));
#14329=CARTESIAN_POINT('Ctrl Pts',(2.3293632006447,-2.22878020685655,-37.0876115240873));
#14330=CARTESIAN_POINT('Ctrl Pts',(2.38758199684161,-2.16630275406731,-37.0818495827687));
#14331=CARTESIAN_POINT('Ctrl Pts',(2.49946924069445,-2.03622041415379,-37.070319701331));
#14332=CARTESIAN_POINT('Ctrl Pts',(2.55301074649338,-1.96867407175026,-37.0645609767881));
#14333=CARTESIAN_POINT('Ctrl Pts',(2.6380727781611,-1.85204634736598,-37.055078673354));
#14334=CARTESIAN_POINT('Ctrl Pts',(2.67108499195885,-1.80410905988064,-37.0513032307019));
#14335=CARTESIAN_POINT('Ctrl Pts',(2.71851485329101,-1.73107736394836,-37.045759840595));
#14336=CARTESIAN_POINT('Ctrl Pts',(2.73392108909224,-1.70664216101776,-37.0439388447458));
#14337=CARTESIAN_POINT('Ctrl Pts',(2.76228110319835,-1.66029168255183,-37.0405523428823));
#14338=CARTESIAN_POINT('Ctrl Pts',(2.7753071965688,-1.6384246581854,-37.0389828798441));
#14339=CARTESIAN_POINT('Ctrl Pts',(2.8084966117567,-1.58117754786866,-37.0349416966247));
#14340=CARTESIAN_POINT('Ctrl Pts',(2.82825157760693,-1.54556430087423,-37.0324935120232));
#14341=CARTESIAN_POINT('Ctrl Pts',(2.93196347960186,-1.34994640937079,-37.0193482395171));
#14342=CARTESIAN_POINT('Ctrl Pts',(3.0030334547773,-1.18345625097854,-37.0092307604122));
#14343=CARTESIAN_POINT('Ctrl Pts',(3.12188889640058,-0.824051868495065,
-36.9879545046333));
#14344=CARTESIAN_POINT('Ctrl Pts',(3.16657046584812,-0.630930709019529,
-36.9768194958653));
#14345=CARTESIAN_POINT('Ctrl Pts',(3.20111379056032,-0.377319400385622,
-36.9617066486205));
#14346=CARTESIAN_POINT('Ctrl Pts',(3.20740073335664,-0.319498594491366,
-36.9582315643087));
#14347=CARTESIAN_POINT('Ctrl Pts',(3.21569091535942,-0.217682928409825,
-36.9520434981848));
#14348=CARTESIAN_POINT('Ctrl Pts',(3.21836325773751,-0.173757219754812,
-36.9493514970819));
#14349=CARTESIAN_POINT('Ctrl Pts',(3.22214940303129,-0.0798231851999515,
-36.9435409237611));
#14350=CARTESIAN_POINT('Ctrl Pts',(3.2230000094219,-0.0298164427737187,
-36.9404150710669));
#14351=CARTESIAN_POINT('Ctrl Pts',(3.22208389723299,0.11642774257034,-36.9311714818407));
#14352=CARTESIAN_POINT('Ctrl Pts',(3.21717037149344,0.212584052119634,-36.9249628364989));
#14353=CARTESIAN_POINT('Ctrl Pts',(3.18755941271854,0.520626446370249,-36.9046634560514));
#14354=CARTESIAN_POINT('Ctrl Pts',(3.14614052381762,0.73032374168661,-36.8901773842451));
#14355=CARTESIAN_POINT('Ctrl Pts',(3.06319476412836,1.00412545347833,-36.8710213754367));
#14356=CARTESIAN_POINT('Ctrl Pts',(3.03970119454276,1.07314854162765,-36.8661758613724));
#14357=CARTESIAN_POINT('Ctrl Pts',(2.99544007236552,1.19002911794051,-36.8580009986111));
#14358=CARTESIAN_POINT('Ctrl Pts',(2.97581472189264,1.23828830629115,-36.8546349451425));
#14359=CARTESIAN_POINT('Ctrl Pts',(2.94393564573099,1.31153840349947,-36.8495619178843));
#14360=CARTESIAN_POINT('Ctrl Pts',(2.93251463023895,1.33688000202048,-36.8478136508048));
#14361=CARTESIAN_POINT('Ctrl Pts',(2.90961938170543,1.38597556806677,-36.8444443942661));
#14362=CARTESIAN_POINT('Ctrl Pts',(2.8981787909384,1.40974216743345,-36.8428219287517));
#14363=CARTESIAN_POINT('Ctrl Pts',(2.86662730329719,1.47327911253003,-36.8385008068562));
#14364=CARTESIAN_POINT('Ctrl Pts',(2.84598035853446,1.51277878983917,-36.8358318021515));
#14365=CARTESIAN_POINT('Ctrl Pts',(2.72611603084671,1.73094512479043,-36.821118478065));
#14366=CARTESIAN_POINT('Ctrl Pts',(2.61088983290953,1.90030277117432,-36.8097815085896));
#14367=CARTESIAN_POINT('Ctrl Pts',(2.40738484442296,2.14562107373458,-36.7918369811821));
#14368=CARTESIAN_POINT('Ctrl Pts',(2.32975290967503,2.22967281374451,-36.7853644909927));
#14369=CARTESIAN_POINT('Ctrl Pts',(2.18752728874511,2.36810506254828,-36.7738822963538));
#14370=CARTESIAN_POINT('Ctrl Pts',(2.12496095515062,2.42440436570682,-36.7689430996895));
#14371=CARTESIAN_POINT('Ctrl Pts',(2.0232919774748,2.50892790000559,-36.7610287398567));
#14372=CARTESIAN_POINT('Ctrl Pts',(1.98563521641259,2.53883478281596,-36.7581201032712));
#14373=CARTESIAN_POINT('Ctrl Pts',(1.91183788837063,2.59479806362307,-36.7524540178461));
#14374=CARTESIAN_POINT('Ctrl Pts',(1.87579827453292,2.62096959724471,-36.7497018671816));
#14375=CARTESIAN_POINT('Ctrl Pts',(1.78789734481723,2.6820604679368,-36.7430189310875));
#14376=CARTESIAN_POINT('Ctrl Pts',(1.73554131265916,2.71623282913346,-36.739062102272));
#14377=CARTESIAN_POINT('Ctrl Pts',(1.55370611120304,2.82751104012485,-36.7253905954449));
#14378=CARTESIAN_POINT('Ctrl Pts',(1.41984161191822,2.89704364316559,-36.7154331439458));
#14379=CARTESIAN_POINT('Ctrl Pts',(1.09579421580223,3.03749411006707,-36.6917583912923));
#14380=CARTESIAN_POINT('Ctrl Pts',(0.902787712234111,3.1003410204323,-36.6779654776262));
#14381=CARTESIAN_POINT('Ctrl Pts',(0.657527378304204,3.15533798471728,-36.66156732129));
#14382=CARTESIAN_POINT('Ctrl Pts',(0.609660039406449,3.16493526701714,-36.6584203903634));
#14383=CARTESIAN_POINT('Ctrl Pts',(0.534825948879233,3.17817833683819,-36.6536017463083));
#14384=CARTESIAN_POINT('Ctrl Pts',(0.508001471684254,3.18257615153751,-36.6518945662789));
#14385=CARTESIAN_POINT('Ctrl Pts',(0.457833939013362,3.1901505317259,-36.6487431403305));
#14386=CARTESIAN_POINT('Ctrl Pts',(0.43450581242328,3.19341151400356,-36.6472943812467));
#14387=CARTESIAN_POINT('Ctrl Pts',(0.368360183675865,3.20191958326549,-36.6432283770199));
#14388=CARTESIAN_POINT('Ctrl Pts',(0.325468588981579,3.20656339930327,-36.6406413189473));
#14389=CARTESIAN_POINT('Ctrl Pts',(0.0772558646317259,3.22840489205267,
-36.6258899543271));
#14390=CARTESIAN_POINT('Ctrl Pts',(-0.129262899783675,3.22674375193573,
-36.614459744368));
#14391=CARTESIAN_POINT('Ctrl Pts',(-0.448489763055395,3.19345779336678,
-36.5963920988824));
#14392=CARTESIAN_POINT('Ctrl Pts',(-0.562029973236523,3.17544263665794,
-36.5898904051983));
#14393=CARTESIAN_POINT('Ctrl Pts',(-0.756880953879801,3.1337469797369,-36.5783642992438));
#14394=CARTESIAN_POINT('Ctrl Pts',(-0.838670004772175,3.11285558371548,
-36.5734112518962));
#14395=CARTESIAN_POINT('Ctrl Pts',(-0.965663684523506,3.07504911826834,
-36.5654803458133));
#14396=CARTESIAN_POINT('Ctrl Pts',(-1.01147136058358,3.06028736409196,-36.5625695300077));
#14397=CARTESIAN_POINT('Ctrl Pts',(-1.098985711136,3.02990591429566,-36.5569025203809));
#14398=CARTESIAN_POINT('Ctrl Pts',(-1.14073303816111,3.01443647682831,-36.5541517019343));
#14399=CARTESIAN_POINT('Ctrl Pts',(-1.24018606445976,2.97522244460751,-36.5474779805147));
#14400=CARTESIAN_POINT('Ctrl Pts',(-1.29754694079023,2.95065775230396,-36.5435292174281));
#14401=CARTESIAN_POINT('Ctrl Pts',(-1.54863581723115,2.83439177346074,-36.5257861834419));
#14402=CARTESIAN_POINT('Ctrl Pts',(-1.733622720393,2.72517481304542,-36.511430163473));
#14403=CARTESIAN_POINT('Ctrl Pts',(-1.99502983227976,2.53338968175026,-36.4895926955401));
#14404=CARTESIAN_POINT('Ctrl Pts',(-2.08029953091262,2.46385125852985,-36.4821913202758));
#14405=CARTESIAN_POINT('Ctrl Pts',(-2.21204941030082,2.34468260880668,-36.470457319682));
#14406=CARTESIAN_POINT('Ctrl Pts',(-2.2608090660935,2.29770380726449,-36.4660423163337));
#14407=CARTESIAN_POINT('Ctrl Pts',(-2.32928382990072,2.22743788388161,-36.4597780894231));
#14408=CARTESIAN_POINT('Ctrl Pts',(-2.35020314631228,2.2053543973062,-36.4578551799428));
#14409=CARTESIAN_POINT('Ctrl Pts',(-2.38792184549556,2.16439025886892,-36.4543764471158));
#14410=CARTESIAN_POINT('Ctrl Pts',(-2.40481591436229,2.1456039686541,-36.4528144856812));
#14411=CARTESIAN_POINT('Ctrl Pts',(-2.44632368301413,2.09834087570868,-36.4489635681865));
#14412=CARTESIAN_POINT('Ctrl Pts',(-2.47066243935511,2.06962831888913,-36.4466929738892));
#14413=CARTESIAN_POINT('Ctrl Pts',(-2.62789688096676,1.87741005359106,-36.4318900954008));
#14414=CARTESIAN_POINT('Ctrl Pts',(-2.74500115013186,1.70161684466447,-36.4201896049185));
#14415=CARTESIAN_POINT('Ctrl Pts',(-2.89981434048922,1.41110681433615,-36.4016689136764));
#14416=CARTESIAN_POINT('Ctrl Pts',(-2.94970902206995,1.30359508714166,-36.3949755180019));
#14417=CARTESIAN_POINT('Ctrl Pts',(-3.02542151465806,1.11370449768179,-36.3831618702812));
#14418=CARTESIAN_POINT('Ctrl Pts',(-3.05405935049314,1.0325854935536,-36.3781187150349));
#14419=CARTESIAN_POINT('Ctrl Pts',(-3.09368826396924,0.904185818639147,
-36.3700795738229));
#14420=CARTESIAN_POINT('Ctrl Pts',(-3.1069149443198,0.857635251862282,-36.3671540043573));
#14421=CARTESIAN_POINT('Ctrl Pts',(-3.13026387493227,0.76781433008927,-36.3614789016122));
#14422=CARTESIAN_POINT('Ctrl Pts',(-3.14054911583673,0.724597626116939,
-36.3587352283597));
#14423=CARTESIAN_POINT('Ctrl Pts',(-3.1629732805215,0.620903553731744,-36.3521151103149));
#14424=CARTESIAN_POINT('Ctrl Pts',(-3.1742752650122,0.560265054473821,-36.3482139011018));
#14425=CARTESIAN_POINT('Ctrl Pts',(-3.21812448121106,0.280680609944262,
-36.33007897963));
#14426=CARTESIAN_POINT('Ctrl Pts',(-3.22979689244493,0.0590957213635396,
-36.3152368439635));
#14427=CARTESIAN_POINT('Ctrl Pts',(-3.21333312897307,-0.268214814711256,
-36.2931647987562));
#14428=CARTESIAN_POINT('Ctrl Pts',(-3.20272109471427,-0.374203673708924,
-36.2860055246003));
#14429=CARTESIAN_POINT('Ctrl Pts',(-3.17700427150586,-0.545132774536986,
-36.2745961397821));
#14430=CARTESIAN_POINT('Ctrl Pts',(-3.16509874051347,-0.610472828562163,
-36.2702683406673));
#14431=CARTESIAN_POINT('Ctrl Pts',(-3.14484894598609,-0.704950980272161,
-36.2641013987289));
#14432=CARTESIAN_POINT('Ctrl Pts',(-3.13810018109963,-0.734410095383784,
-36.2621915473615));
#14433=CARTESIAN_POINT('Ctrl Pts',(-3.12493895610913,-0.788362088487279,
-36.2587232018279));
#14434=CARTESIAN_POINT('Ctrl Pts',(-3.1186510706632,-0.812879940919055,
-36.2571589035257));
#14435=CARTESIAN_POINT('Ctrl Pts',(-3.10220023504282,-0.874022652333175,
-36.2532838048014));
#14436=CARTESIAN_POINT('Ctrl Pts',(-3.09167719487609,-0.910546154656176,
-36.2509919509918));
#14437=CARTESIAN_POINT('Ctrl Pts',(-3.01957730679511,-1.1451114648457,-36.2363716006436));
#14438=CARTESIAN_POINT('Ctrl Pts',(-2.93964476949381,-1.33702496849744,
-36.2248442199179));
#14439=CARTESIAN_POINT('Ctrl Pts',(-2.78526891677148,-1.62565927197093,
-36.2064316310738));
#14440=CARTESIAN_POINT('Ctrl Pts',(-2.72287280848679,-1.7281355464251,-36.1996601759258));
#14441=CARTESIAN_POINT('Ctrl Pts',(-2.60580124597897,-1.898268718711,-36.1877300085402));
#14442=CARTESIAN_POINT('Ctrl Pts',(-2.55383160173638,-1.96762970265087,
-36.1826507867877));
#14443=CARTESIAN_POINT('Ctrl Pts',(-2.46851431462195,-2.07241560396686,
-36.174568300428));
#14444=CARTESIAN_POINT('Ctrl Pts',(-2.43705128269534,-2.10932454297226,
-36.1716368206507));
#14445=CARTESIAN_POINT('Ctrl Pts',(-2.37521939414734,-2.17862811997138,
-36.1659582170153));
#14446=CARTESIAN_POINT('Ctrl Pts',(-2.34499025547948,-2.21113275370532,
-36.1632171424686));
#14447=CARTESIAN_POINT('Ctrl Pts',(-2.27136394556417,-2.28709288345824,
-36.1566171003333));
#14448=CARTESIAN_POINT('Ctrl Pts',(-2.22737834136518,-2.32995127812476,
-36.1527337795605));
#14449=CARTESIAN_POINT('Ctrl Pts',(-2.01753986888988,-2.52303759016171,
-36.1344654577454));
#14450=CARTESIAN_POINT('Ctrl Pts',(-1.83757175526662,-2.65696979043442,
-36.1194553422679));
#14451=CARTESIAN_POINT('Ctrl Pts',(-1.5546848266988,-2.82491735448134,-36.097299387746));
#14452=CARTESIAN_POINT('Ctrl Pts',(-1.46156738123851,-2.87419998621752,
-36.0902203807229));
#14453=CARTESIAN_POINT('Ctrl Pts',(-1.30646206170698,-2.94679912206043,
-36.078919129597));
#14454=CARTESIAN_POINT('Ctrl Pts',(-1.24587425542452,-2.97292225469375,
-36.0746207415771));
#14455=CARTESIAN_POINT('Ctrl Pts',(-1.15648138123724,-3.00825157800046,
-36.0684866633764));
#14456=CARTESIAN_POINT('Ctrl Pts',(-1.12828397849175,-3.01894056944114,
-36.0665812584264));
#14457=CARTESIAN_POINT('Ctrl Pts',(-1.07613164413316,-3.03787751489069,
-36.0631163856028));
#14458=CARTESIAN_POINT('Ctrl Pts',(-1.05222419946695,-3.0462408606694,-36.0615512279953));
#14459=CARTESIAN_POINT('Ctrl Pts',(-0.992076986397332,-3.06648904320856,
-36.0576675683651));
#14460=CARTESIAN_POINT('Ctrl Pts',(-0.955720632842481,-3.07801399534661,
-36.0553682195607));
#14461=CARTESIAN_POINT('Ctrl Pts',(-0.721519958336437,-3.14770547721308,
-36.0408127560886));
#14462=CARTESIAN_POINT('Ctrl Pts',(-0.518661636472471,-3.18742064519333,
-36.029347028721));
#14463=CARTESIAN_POINT('Ctrl Pts',(-0.193542023589923,-3.21918582058902,
-36.010972564263));
#14464=CARTESIAN_POINT('Ctrl Pts',(-0.073146526034735,-3.22416861074646,
-36.0041731332972));
#14465=CARTESIAN_POINT('Ctrl Pts',(0.134101229839968,-3.22113037301194,
-35.9922013000168));
#14466=CARTESIAN_POINT('Ctrl Pts',(0.220869375881308,-3.21634559109624,
-35.9871092559391));
#14467=CARTESIAN_POINT('Ctrl Pts',(0.355645001954417,-3.20343403313489,
-35.9790113854823));
#14468=CARTESIAN_POINT('Ctrl Pts',(0.403843594446042,-3.1977152699262,-35.9760778345149));
#14469=CARTESIAN_POINT('Ctrl Pts',(0.495827415973493,-3.18468863401984,
-35.9703980338708));
#14470=CARTESIAN_POINT('Ctrl Pts',(0.539627004562982,-3.17756021432315,
-35.9676579005885));
#14471=CARTESIAN_POINT('Ctrl Pts',(0.643560070621952,-3.15843422448798,
-35.9610649905727));
#14472=CARTESIAN_POINT('Ctrl Pts',(0.70352393929789,-3.14562070005593,-35.9571880051658));
#14473=CARTESIAN_POINT('Ctrl Pts',(1.00974351257171,-3.07099181385787,-35.9369979642906));
#14474=CARTESIAN_POINT('Ctrl Pts',(1.24840617831193,-2.98194843288396,-35.919848896879));
#14475=CARTESIAN_POINT('Ctrl Pts',(1.55119609875955,-2.82620307115287,-35.8969661843085));
#14476=CARTESIAN_POINT('Ctrl Pts',(1.62666041847073,-2.78345297153647,-35.8911704167628));
#14477=CARTESIAN_POINT('Ctrl Pts',(1.74994341087111,-2.70688548565644,-35.8816360030103));
#14478=CARTESIAN_POINT('Ctrl Pts',(1.79873059856379,-2.67471495584634,-35.8778448521494));
#14479=CARTESIAN_POINT('Ctrl Pts',(1.87032490588861,-2.6246597819614,-35.8722834962769));
#14480=CARTESIAN_POINT('Ctrl Pts',(1.89380754044571,-2.60776673889777,-35.8704597744819));
#14481=CARTESIAN_POINT('Ctrl Pts',(1.9375086163502,-2.57542715407489,-35.8670713503549));
#14482=CARTESIAN_POINT('Ctrl Pts',(1.95777682129483,-2.5600536349338,-35.8655026220409));
#14483=CARTESIAN_POINT('Ctrl Pts',(2.00993409369761,-2.5195104111105,-35.8614679039294));
#14484=CARTESIAN_POINT('Ctrl Pts',(2.04153418781651,-2.49397399119942,-35.8590252877775));
#14485=CARTESIAN_POINT('Ctrl Pts',(2.1404817407716,-2.41087191038697,-35.8513527509625));
#14486=CARTESIAN_POINT('Ctrl Pts',(2.20591396337446,-2.35114792362527,-35.8462418756784));
#14487=CARTESIAN_POINT('Ctrl Pts',(2.26878031087686,-2.28883233625302,-35.8411988517434));
#14488=CARTESIAN_POINT('Origin',(0.,0.,-41.3107734492731));
#14489=CARTESIAN_POINT('',(2.26878010865581,-2.28883253670244,-34.3485046109761));
#14490=CARTESIAN_POINT('',(2.26878020184338,-2.28883244433128,-34.5957191253299));
#14491=CARTESIAN_POINT('',(2.26878020078428,-2.2888324453811,-41.3107734492731));
#14492=CARTESIAN_POINT('Ctrl Pts',(2.2687801086558,-2.28883253670245,-34.3485046109761));
#14493=CARTESIAN_POINT('Ctrl Pts',(2.15700584426002,-2.39962754841884,-34.3575848935098));
#14494=CARTESIAN_POINT('Ctrl Pts',(2.03721275441062,-2.50213866773743,-34.366358323638));
#14495=CARTESIAN_POINT('Ctrl Pts',(1.81827356931631,-2.66328125615279,-34.3816629304255));
#14496=CARTESIAN_POINT('Ctrl Pts',(1.72266971123268,-2.7260947863319,-34.3881340470896));
#14497=CARTESIAN_POINT('Ctrl Pts',(1.5512683466518,-2.82608592203579,-34.3996141200708));
#14498=CARTESIAN_POINT('Ctrl Pts',(1.47697419281886,-2.86561349792613,-34.4045526052959));
#14499=CARTESIAN_POINT('Ctrl Pts',(1.35792484610279,-2.92309243929206,-34.4124660255598));
#14500=CARTESIAN_POINT('Ctrl Pts',(1.31416629502935,-2.94302495384176,-34.4153744560725));
#14501=CARTESIAN_POINT('Ctrl Pts',(1.22904826684484,-2.97952031683764,-34.4210402393136));
#14502=CARTESIAN_POINT('Ctrl Pts',(1.18775893223603,-2.99621917983728,-34.4237922965348));
#14503=CARTESIAN_POINT('Ctrl Pts',(1.08771353214931,-3.03428814414662,-34.430475145985));
#14504=CARTESIAN_POINT('Ctrl Pts',(1.02865763813113,-3.05481388859171,-34.4344319849203));
#14505=CARTESIAN_POINT('Ctrl Pts',(0.825336125197219,-3.11891696388786,
-34.4481038307153));
#14506=CARTESIAN_POINT('Ctrl Pts',(0.678642483971953,-3.15408589545084,
-34.4580616438956));
#14507=CARTESIAN_POINT('Ctrl Pts',(0.330259734717609,-3.21217510004361,
-34.4817377001873));
#14508=CARTESIAN_POINT('Ctrl Pts',(0.12777831773368,-3.22657988157259,-34.495531584636));
#14509=CARTESIAN_POINT('Ctrl Pts',(-0.123517059971134,-3.22075201923825,
-34.5119305997965));
#14510=CARTESIAN_POINT('Ctrl Pts',(-0.172285430652327,-3.21851181774909,
-34.515077531067));
#14511=CARTESIAN_POINT('Ctrl Pts',(-0.248102191478151,-3.21330073025679,
-34.519896112185));
#14512=CARTESIAN_POINT('Ctrl Pts',(-0.275194031599388,-3.21109399499259,
-34.5216032320977));
#14513=CARTESIAN_POINT('Ctrl Pts',(-0.325704457999064,-3.20633574169521,
-34.5247545381566));
#14514=CARTESIAN_POINT('Ctrl Pts',(-0.349128932961697,-3.20386974433673,
-34.5262032379756));
#14515=CARTESIAN_POINT('Ctrl Pts',(-0.4153669684613,-3.19616146903437,-34.5302689168139));
#14516=CARTESIAN_POINT('Ctrl Pts',(-0.458106839413337,-3.19031603007539,
-34.5328557156488));
#14517=CARTESIAN_POINT('Ctrl Pts',(-0.704254303229759,-3.1516019675485,
-34.5476072367903));
#14518=CARTESIAN_POINT('Ctrl Pts',(-0.904272043636709,-3.10014171965664,
-34.5590377638131));
#14519=CARTESIAN_POINT('Ctrl Pts',(-1.20603458439057,-2.99078534656033,
-34.5771058785864));
#14520=CARTESIAN_POINT('Ctrl Pts',(-1.31187208619722,-2.9458964546036,-34.583607721888));
#14521=CARTESIAN_POINT('Ctrl Pts',(-1.49090168313425,-2.85840013740546,
-34.5951340674383));
#14522=CARTESIAN_POINT('Ctrl Pts',(-1.56523120276755,-2.81838407721604,
-34.6000872000718));
#14523=CARTESIAN_POINT('Ctrl Pts',(-1.67934619186124,-2.75104159134923,
-34.6080182162998));
#14524=CARTESIAN_POINT('Ctrl Pts',(-1.72023668208287,-2.72565934404721,
-34.6109290538131));
#14525=CARTESIAN_POINT('Ctrl Pts',(-1.79783058004558,-2.67505227210551,
-34.6165960907502));
#14526=CARTESIAN_POINT('Ctrl Pts',(-1.83460971359678,-2.64996346130282,
-34.6193469144118));
#14527=CARTESIAN_POINT('Ctrl Pts',(-1.92165686580859,-2.58790358006154,
-34.6260206282659));
#14528=CARTESIAN_POINT('Ctrl Pts',(-1.97139231540311,-2.55021990303089,
-34.6299693779722));
#14529=CARTESIAN_POINT('Ctrl Pts',(-2.13530465371551,-2.41836512718779,
-34.643458630102));
#14530=CARTESIAN_POINT('Ctrl Pts',(-2.24407082621219,-2.31779057106791,
-34.6532315648553));
#14531=CARTESIAN_POINT('Ctrl Pts',(-2.43666998029154,-2.1133901351265,-34.6720491091999));
#14532=CARTESIAN_POINT('Ctrl Pts',(-2.52173594617269,-2.01112554606369,
-34.6810464597918));
#14533=CARTESIAN_POINT('Ctrl Pts',(-2.64139660869419,-1.84769956315272,
-34.6945927172459));
#14534=CARTESIAN_POINT('Ctrl Pts',(-2.68071723906216,-1.79017478774294,
-34.6992163509935));
#14535=CARTESIAN_POINT('Ctrl Pts',(-2.7452771635445,-1.6888225015762,-34.7070668152836));
#14536=CARTESIAN_POINT('Ctrl Pts',(-2.7714066487484,-1.64559227716962,-34.7103269275318));
#14537=CARTESIAN_POINT('Ctrl Pts',(-2.8101787528156,-1.57790025045115,-34.7152772125008));
#14538=CARTESIAN_POINT('Ctrl Pts',(-2.82354139393212,-1.55386226634818,
-34.717005819691));
#14539=CARTESIAN_POINT('Ctrl Pts',(-2.84768639832253,-1.50908772944498,
-34.7201677771165));
#14540=CARTESIAN_POINT('Ctrl Pts',(-2.85855379229225,-1.4883997667111,-34.7216061730157));
#14541=CARTESIAN_POINT('Ctrl Pts',(-2.888308160447,-1.43022901639573,-34.7255929003826));
#14542=CARTESIAN_POINT('Ctrl Pts',(-2.90669009308099,-1.39249134217169,
-34.7281130055937));
#14543=CARTESIAN_POINT('Ctrl Pts',(-2.9834843888935,-1.22668262085376,-34.7389454743223));
#14544=CARTESIAN_POINT('Ctrl Pts',(-3.03421295903237,-1.09521150202432,
-34.7469241659683));
#14545=CARTESIAN_POINT('Ctrl Pts',(-3.12276655164491,-0.811700281835316,
-34.7636518480597));
#14546=CARTESIAN_POINT('Ctrl Pts',(-3.15844057919212,-0.659378186072398,
-34.7723718958333));
#14547=CARTESIAN_POINT('Ctrl Pts',(-3.19871767776629,-0.405556570087333,
-34.7871099169284));
#14548=CARTESIAN_POINT('Ctrl Pts',(-3.20983238129255,-0.305359483045984,
-34.792976886234));
#14549=CARTESIAN_POINT('Ctrl Pts',(-3.21945636374139,-0.154230778247315,
-34.8020023677299));
#14550=CARTESIAN_POINT('Ctrl Pts',(-3.22148360358471,-0.103582721474755,
-34.8050561936212));
#14551=CARTESIAN_POINT('Ctrl Pts',(-3.22303646590291,-0.00901041361086034,
-34.8108234095914));
#14552=CARTESIAN_POINT('Ctrl Pts',(-3.22286008437264,0.0348974613347764,
-34.8135270896846));
#14553=CARTESIAN_POINT('Ctrl Pts',(-3.22041634235099,0.134828572752071,
-34.8197455264607));
#14554=CARTESIAN_POINT('Ctrl Pts',(-3.21758392805247,0.190822478239483,
-34.8232765832901));
#14555=CARTESIAN_POINT('Ctrl Pts',(-3.20105477719983,0.406106380548137,
-34.8370420230614));
#14556=CARTESIAN_POINT('Ctrl Pts',(-3.17697527065622,0.564349734224334,
-34.8475757196387));
#14557=CARTESIAN_POINT('Ctrl Pts',(-3.10587378834236,0.874497057878567,
-34.8688880136112));
#14558=CARTESIAN_POINT('Ctrl Pts',(-3.05915714949187,1.02603839900073,-34.8796332095907));
#14559=CARTESIAN_POINT('Ctrl Pts',(-2.97147372618767,1.25030245186017,-34.8956434110911));
#14560=CARTESIAN_POINT('Ctrl Pts',(-2.93852073077748,1.32589982133244,-34.9010572132222));
#14561=CARTESIAN_POINT('Ctrl Pts',(-2.88862319236059,1.42934383474286,-34.9084147909857));
#14562=CARTESIAN_POINT('Ctrl Pts',(-2.87410375741152,1.45831941836085,-34.9104699256199));
#14563=CARTESIAN_POINT('Ctrl Pts',(-2.84761106202955,1.5092561243403,-34.914066056812));
#14564=CARTESIAN_POINT('Ctrl Pts',(-2.83581575709415,1.53130397909653,-34.9156164591919));
#14565=CARTESIAN_POINT('Ctrl Pts',(-2.8070517461125,1.58359731731963,-34.9192804387879));
#14566=CARTESIAN_POINT('Ctrl Pts',(-2.78984961915996,1.61370979201426,-34.9213803325797));
#14567=CARTESIAN_POINT('Ctrl Pts',(-2.72087174896168,1.73005497251443,-34.9294774931738));
#14568=CARTESIAN_POINT('Ctrl Pts',(-2.66555301386505,1.81412895273838,-34.9352943191486));
#14569=CARTESIAN_POINT('Ctrl Pts',(-2.51775092655695,2.01736441106725,-34.949613897843));
#14570=CARTESIAN_POINT('Ctrl Pts',(-2.42067258631048,2.13287955687515,-34.9579993181559));
#14571=CARTESIAN_POINT('Ctrl Pts',(-2.24644231211711,2.31291595012444,-34.9721556750646));
#14572=CARTESIAN_POINT('Ctrl Pts',(-2.17372684684648,2.38138470599216,-34.9778435854657));
#14573=CARTESIAN_POINT('Ctrl Pts',(-2.03941000172662,2.49657216369485,-34.9881263006929));
#14574=CARTESIAN_POINT('Ctrl Pts',(-1.97908574658288,2.5446579390078,-34.9926716634702));
#14575=CARTESIAN_POINT('Ctrl Pts',(-1.87939851657902,2.61843052029085,-35.0001129422563));
#14576=CARTESIAN_POINT('Ctrl Pts',(-1.84109610222593,2.64550221572821,-35.0029561941834));
#14577=CARTESIAN_POINT('Ctrl Pts',(-1.7648061163322,2.69696374746712,-35.0085967852438));
#14578=CARTESIAN_POINT('Ctrl Pts',(-1.7268698184464,2.72141036864695,-35.0113911636954));
#14579=CARTESIAN_POINT('Ctrl Pts',(-1.63180585265499,2.77988258618225,-35.0183738222498));
#14580=CARTESIAN_POINT('Ctrl Pts',(-1.57411681069742,2.81295090543525,-35.0225944000651));
#14581=CARTESIAN_POINT('Ctrl Pts',(-1.44470459437286,2.88190421653859,-35.032031106279));
#14582=CARTESIAN_POINT('Ctrl Pts',(-1.3725824014475,2.91694348879139,-35.0372703484799));
#14583=CARTESIAN_POINT('Ctrl Pts',(-1.10965187998685,3.03277204486511,-35.0562726155883));
#14584=CARTESIAN_POINT('Ctrl Pts',(-0.912461961896676,3.09781191070751,
-35.0703807730241));
#14585=CARTESIAN_POINT('Ctrl Pts',(-0.625475374497176,3.16266997724789,
-35.0899860035357));
#14586=CARTESIAN_POINT('Ctrl Pts',(-0.539785471905421,3.1784170313087,-35.0957207452498));
#14587=CARTESIAN_POINT('Ctrl Pts',(-0.420552224945453,3.19536613024062,
-35.1034509951651));
#14588=CARTESIAN_POINT('Ctrl Pts',(-0.387475243087062,3.19954559569184,
-35.1055691057823));
#14589=CARTESIAN_POINT('Ctrl Pts',(-0.329509648010112,3.20595772580962,
-35.1092281946368));
#14590=CARTESIAN_POINT('Ctrl Pts',(-0.304650750548156,3.20841543033335,
-35.1107800447365));
#14591=CARTESIAN_POINT('Ctrl Pts',(-0.246841077342685,3.21345283830605,
-35.1143488701027));
#14592=CARTESIAN_POINT('Ctrl Pts',(-0.213875251475101,3.21581517404566,
-35.1163547588733));
#14593=CARTESIAN_POINT('Ctrl Pts',(-0.0930033442108636,3.22260984352113,
-35.123621325248));
#14594=CARTESIAN_POINT('Ctrl Pts',(-0.00495643619134498,3.22394816095712,
-35.128744378643));
#14595=CARTESIAN_POINT('Ctrl Pts',(0.265484150667288,3.21697734410398,-35.1442463003433));
#14596=CARTESIAN_POINT('Ctrl Pts',(0.447202374201056,3.19678583647782,-35.1543518866553));
#14597=CARTESIAN_POINT('Ctrl Pts',(0.75478555717288,3.13585536735573,-35.1721210086342));
#14598=CARTESIAN_POINT('Ctrl Pts',(0.881647955232236,3.1025767235475,-35.1796485045852));
#14599=CARTESIAN_POINT('Ctrl Pts',(1.05906921337028,3.04427261081192,-35.1907054745601));
#14600=CARTESIAN_POINT('Ctrl Pts',(1.11155041612107,3.02550466091211,-35.1940435891295));
#14601=CARTESIAN_POINT('Ctrl Pts',(1.20437532491047,2.98956807952176,-35.2000842424896));
#14602=CARTESIAN_POINT('Ctrl Pts',(1.24490572054345,2.97291888296745,-35.2027694218143));
#14603=CARTESIAN_POINT('Ctrl Pts',(1.33237515967555,2.93488559233414,-35.2086748778193));
#14604=CARTESIAN_POINT('Ctrl Pts',(1.37916498930865,2.91319076984041,-35.2119048792196));
#14605=CARTESIAN_POINT('Ctrl Pts',(1.52143860638185,2.84302757691006,-35.2219545429626));
#14606=CARTESIAN_POINT('Ctrl Pts',(1.61503634061994,2.79092009456253,-35.2288921709981));
#14607=CARTESIAN_POINT('Ctrl Pts',(1.85550250735081,2.6408969571709,-35.2475774212668));
#14608=CARTESIAN_POINT('Ctrl Pts',(1.99722069913298,2.53541483346839,-35.2595141716288));
#14609=CARTESIAN_POINT('Ctrl Pts',(2.22194170354755,2.33756994612819,-35.2796272495667));
#14610=CARTESIAN_POINT('Ctrl Pts',(2.30957218088143,2.25103079011394,-35.287827185852));
#14611=CARTESIAN_POINT('Ctrl Pts',(2.41634378832392,2.13277168207641,-35.2980900640551));
#14612=CARTESIAN_POINT('Ctrl Pts',(2.44018823150816,2.10544864589801,-35.3004010430417));
#14613=CARTESIAN_POINT('Ctrl Pts',(2.47976067797567,2.05852748541694,-35.3042608866362));
#14614=CARTESIAN_POINT('Ctrl Pts',(2.49572904666603,2.0391383222866,-35.3058251761443));
#14615=CARTESIAN_POINT('Ctrl Pts',(2.53104779020776,1.99521693535195,-35.309299240326));
#14616=CARTESIAN_POINT('Ctrl Pts',(2.5502707586273,1.97058690795218,-35.3112008888017));
#14617=CARTESIAN_POINT('Ctrl Pts',(2.61344449778358,1.88717044498049,-35.3175017999067));
#14618=CARTESIAN_POINT('Ctrl Pts',(2.65574726692722,1.8271596682661,-35.3218075352602));
#14619=CARTESIAN_POINT('Ctrl Pts',(2.76536485063017,1.65979456666491,-35.3333614219237));
#14620=CARTESIAN_POINT('Ctrl Pts',(2.82845962271793,1.54983226508888,-35.3404704309024));
#14621=CARTESIAN_POINT('Ctrl Pts',(2.96805273031486,1.26947536284365,-35.3580731674177));
#14622=CARTESIAN_POINT('Ctrl Pts',(3.03652744225533,1.09562680945297,-35.368562364152));
#14623=CARTESIAN_POINT('Ctrl Pts',(3.10771481836829,0.855738501234879,-35.3832566992314));
#14624=CARTESIAN_POINT('Ctrl Pts',(3.12402939344504,0.794115443589744,-35.3870472893939));
#14625=CARTESIAN_POINT('Ctrl Pts',(3.14866151122781,0.688510875674616,-35.393593406024));
#14626=CARTESIAN_POINT('Ctrl Pts',(3.1579098371248,0.644764838406605,-35.3963193841941));
#14627=CARTESIAN_POINT('Ctrl Pts',(3.17513239046499,0.554007524635492,-35.4020108906884));
#14628=CARTESIAN_POINT('Ctrl Pts',(3.18297931941968,0.506983539569178,-35.404979616173));
#14629=CARTESIAN_POINT('Ctrl Pts',(3.20143322228754,0.378964200486526,-35.4131216186116));
#14630=CARTESIAN_POINT('Ctrl Pts',(3.21000808518044,0.297716010688075,-35.4183543283446));
#14631=CARTESIAN_POINT('Ctrl Pts',(3.22280641341184,0.107400609165122,-35.4307647231612));
#14632=CARTESIAN_POINT('Ctrl Pts',(3.22459453473107,-0.00172737352979303,
-35.4379992562718));
#14633=CARTESIAN_POINT('Ctrl Pts',(3.21320166933526,-0.333119993313931,
-35.4602137468149));
#14634=CARTESIAN_POINT('Ctrl Pts',(3.18254381919031,-0.554126004956237,
-35.4754021874223));
#14635=CARTESIAN_POINT('Ctrl Pts',(3.11978679271869,-0.809105689326679,
-35.4923923928286));
#14636=CARTESIAN_POINT('Ctrl Pts',(3.10949022012298,-0.847816342486037,
-35.4949553300529));
#14637=CARTESIAN_POINT('Ctrl Pts',(3.09150279239003,-0.910697859025966,
-35.4990807293006));
#14638=CARTESIAN_POINT('Ctrl Pts',(3.08424378365282,-0.934986928939391,
-35.5006647696574));
#14639=CARTESIAN_POINT('Ctrl Pts',(3.06802235357057,-0.98701880831585,-35.5040348461883));
#14640=CARTESIAN_POINT('Ctrl Pts',(3.05896885323836,-1.01473000639363,-35.5058160261602));
#14641=CARTESIAN_POINT('Ctrl Pts',(3.03021604938352,-1.09885311185906,-35.5111920557482));
#14642=CARTESIAN_POINT('Ctrl Pts',(3.00932205699648,-1.15484594100018,-35.5147273853425));
#14643=CARTESIAN_POINT('Ctrl Pts',(2.95316984913018,-1.29343131086734,-35.5234435463508));
#14644=CARTESIAN_POINT('Ctrl Pts',(2.91599410384748,-1.37519336744652,-35.528555473604));
#14645=CARTESIAN_POINT('Ctrl Pts',(2.76456548512911,-1.67439319643931,-35.5475013444154));
#14646=CARTESIAN_POINT('Ctrl Pts',(2.629012717813,-1.88007998604159,-35.5610835686793));
#14647=CARTESIAN_POINT('Ctrl Pts',(2.43119495573586,-2.11644447820218,-35.5792010272464));
#14648=CARTESIAN_POINT('Ctrl Pts',(2.38957608063778,-2.16332418873763,-35.5829318836063));
#14649=CARTESIAN_POINT('Ctrl Pts',(2.32113404127666,-2.23603147064495,-35.588963307873));
#14650=CARTESIAN_POINT('Ctrl Pts',(2.29518395708476,-2.26266000989839,-35.5912278113247));
#14651=CARTESIAN_POINT('Ctrl Pts',(2.26878020052865,-2.28883244563449,-35.5935118781384));
#14652=CARTESIAN_POINT('Ctrl Pts',(2.26878031087686,-2.28883233625302,-35.8411988517434));
#14653=CARTESIAN_POINT('Ctrl Pts',(2.3352642194958,-2.2229308805301,-35.8358656336423));
#14654=CARTESIAN_POINT('Ctrl Pts',(2.39887845558188,-2.15413101434946,-35.8306078869139));
#14655=CARTESIAN_POINT('Ctrl Pts',(2.58543395974036,-1.93382159103378,-35.8143819814439));
#14656=CARTESIAN_POINT('Ctrl Pts',(2.69765956891768,-1.7739104211318,-35.8034030000764));
#14657=CARTESIAN_POINT('Ctrl Pts',(2.8239873749062,-1.55391820984128,-35.7884331224572));
#14658=CARTESIAN_POINT('Ctrl Pts',(2.85183321938616,-1.50220276761051,-35.7849255811006));
#14659=CARTESIAN_POINT('Ctrl Pts',(2.89807255958858,-1.41040235386445,-35.7787014572064));
#14660=CARTESIAN_POINT('Ctrl Pts',(2.91708557042082,-1.37064614107615,-35.7760067120446));
#14661=CARTESIAN_POINT('Ctrl Pts',(2.95579910417561,-1.28523934759973,-35.7702130346711));
#14662=CARTESIAN_POINT('Ctrl Pts',(2.97527020600965,-1.23949800263655,-35.7671073183813));
#14663=CARTESIAN_POINT('Ctrl Pts',(3.02857798210034,-1.10576583198921,-35.7580123216606));
#14664=CARTESIAN_POINT('Ctrl Pts',(3.05961980623481,-1.01672345909062,-35.751936752157));
#14665=CARTESIAN_POINT('Ctrl Pts',(3.14899064177308,-0.718962594587075,
-35.7315647453863));
#14666=CARTESIAN_POINT('Ctrl Pts',(3.19018363631925,-0.505729780936466,
-35.7168458592631));
#14667=CARTESIAN_POINT('Ctrl Pts',(3.21621819047205,-0.217589292394158,
-35.6974752454061));
#14668=CARTESIAN_POINT('Ctrl Pts',(3.22030896490971,-0.144968167778426,
-35.6926418127545));
#14669=CARTESIAN_POINT('Ctrl Pts',(3.22310572519618,-0.0202788587376412,
-35.6844844986759));
#14670=CARTESIAN_POINT('Ctrl Pts',(3.2230133999614,0.0317337139200843,-35.6811241054923));
#14671=CARTESIAN_POINT('Ctrl Pts',(3.22094058042385,0.111494639841122,-35.6760575422183));
#14672=CARTESIAN_POINT('Ctrl Pts',(3.21985981988505,0.139255677651452,-35.6743102376787));
#14673=CARTESIAN_POINT('Ctrl Pts',(3.21705282575042,0.193351881914526,-35.6709412599188));
#14674=CARTESIAN_POINT('Ctrl Pts',(3.21536186256889,0.219686113523178,-35.6693181418974));
#14675=CARTESIAN_POINT('Ctrl Pts',(3.20994116781044,0.290494126147055,-35.6649925930572));
#14676=CARTESIAN_POINT('Ctrl Pts',(3.20561064170182,0.334917873948849,-35.6623199245407));
#14677=CARTESIAN_POINT('Ctrl Pts',(3.17631952792257,0.582102106214547,-35.6476083543977));
#14678=CARTESIAN_POINT('Ctrl Pts',(3.13304428715088,0.78223958459152,-35.6362756330802));
#14679=CARTESIAN_POINT('Ctrl Pts',(3.03645169598095,1.0858853185833,-35.6183367593132));
#14680=CARTESIAN_POINT('Ctrl Pts',(2.99602741198798,1.19289709093965,-35.6118656414026));
#14681=CARTESIAN_POINT('Ctrl Pts',(2.91613410060458,1.37453884301584,-35.6003855665772));
#14682=CARTESIAN_POINT('Ctrl Pts',(2.8792625904275,1.4501863406919,-35.5954470807774));
#14683=CARTESIAN_POINT('Ctrl Pts',(2.81673491560534,1.5666632412962,-35.5875336598621));
#14684=CARTESIAN_POINT('Ctrl Pts',(2.79304954196039,1.60850961644331,-35.5846252292824));
#14685=CARTESIAN_POINT('Ctrl Pts',(2.74563904741926,1.68806610707185,-35.5789594460696));
#14686=CARTESIAN_POINT('Ctrl Pts',(2.72205062044186,1.72584503196518,-35.5762073889462));
#14687=CARTESIAN_POINT('Ctrl Pts',(2.66348857227354,1.81544867575635,-35.5695245400191));
#14688=CARTESIAN_POINT('Ctrl Pts',(2.62777608443872,1.8667665305759,-35.5655677015226));
#14689=CARTESIAN_POINT('Ctrl Pts',(2.50096445415971,2.03813628233367,-35.5518958649956));
#14690=CARTESIAN_POINT('Ctrl Pts',(2.40295868190494,2.1528128086686,-35.5419380612097));
#14691=CARTESIAN_POINT('Ctrl Pts',(2.15525510626092,2.40458226337193,-35.5182620034814));
#14692=CARTESIAN_POINT('Ctrl Pts',(1.99991099440145,2.535251686477,-35.5044681073185));
#14693=CARTESIAN_POINT('Ctrl Pts',(1.79318309875631,2.67824465028816,-35.4880690820898));
#14694=CARTESIAN_POINT('Ctrl Pts',(1.75241190949501,2.70509761173168,-35.4849221515694));
#14695=CARTESIAN_POINT('Ctrl Pts',(1.68801187211209,2.74544571972678,-35.4801035713358));
#14696=CARTESIAN_POINT('Ctrl Pts',(1.66479702851349,2.75958461610264,-35.4783964515819));
#14697=CARTESIAN_POINT('Ctrl Pts',(1.62113640513057,2.78542439108237,-35.4752451456248));
#14698=CARTESIAN_POINT('Ctrl Pts',(1.60073612904937,2.79719791857979,-35.473796445753));
#14699=CARTESIAN_POINT('Ctrl Pts',(1.5426176152966,2.82989553661957,-35.4697307664582));
#14700=CARTESIAN_POINT('Ctrl Pts',(1.50460446448734,2.8502883457805,-35.4671439672262));
#14701=CARTESIAN_POINT('Ctrl Pts',(1.28271142795066,2.96364985697702,-35.4523924461607));
#14702=CARTESIAN_POINT('Ctrl Pts',(1.09064610887298,3.03958511523094,-35.4409619193667));
#14703=CARTESIAN_POINT('Ctrl Pts',(0.782237031361676,3.12848551765377,-35.4228938048794));
#14704=CARTESIAN_POINT('Ctrl Pts',(0.670227667279095,3.15437936292708,-35.4163919616088));
#14705=CARTESIAN_POINT('Ctrl Pts',(0.47396063935328,3.18882431100243,-35.4048656161305));
#14706=CARTESIAN_POINT('Ctrl Pts',(0.390305945875559,3.20014043336239,-35.399912483523));
#14707=CARTESIAN_POINT('Ctrl Pts',(0.258402061867658,3.21273432512499,-35.3919814673502));
#14708=CARTESIAN_POINT('Ctrl Pts',(0.21040165012732,3.21623448270812,-35.3890706298528));
#14709=CARTESIAN_POINT('Ctrl Pts',(0.117880778127801,3.22090105019819,-35.3834035929523));
#14710=CARTESIAN_POINT('Ctrl Pts',(0.0733790013280007,3.22222200811857,
-35.3806527693102));
#14711=CARTESIAN_POINT('Ctrl Pts',(-0.0335215065450131,3.22317954172133,
-35.373979055508));
#14712=CARTESIAN_POINT('Ctrl Pts',(-0.0959082398382097,3.22192657032154,
-35.3700303058386));
#14713=CARTESIAN_POINT('Ctrl Pts',(-0.306018399468717,3.21159907082808,
-35.356541053828));
#14714=CARTESIAN_POINT('Ctrl Pts',(-0.453128322195566,3.1941636977453,-35.3467681191974));
#14715=CARTESIAN_POINT('Ctrl Pts',(-0.729087873775642,3.1420072133465,-35.3279505750423));
#14716=CARTESIAN_POINT('Ctrl Pts',(-0.858017304166652,3.10927394262781,
-35.3189532245111));
#14717=CARTESIAN_POINT('Ctrl Pts',(-1.05088419609975,3.04739431749685,-35.3054069672449));
#14718=CARTESIAN_POINT('Ctrl Pts',(-1.11650746773125,3.02396788356028,-35.3007833336355));
#14719=CARTESIAN_POINT('Ctrl Pts',(-1.22831092107886,2.97991953374572,-35.292932869543));
#14720=CARTESIAN_POINT('Ctrl Pts',(-1.27486020639078,2.96030407382419,-35.2896727573618));
#14721=CARTESIAN_POINT('Ctrl Pts',(-1.34601587167561,2.92832974515092,-35.2847224724694));
#14722=CARTESIAN_POINT('Ctrl Pts',(-1.37095564778479,2.91673697097014,-35.2829938652967));
#14723=CARTESIAN_POINT('Ctrl Pts',(-1.41680717881892,2.89470568735291,-35.2798319078943));
#14724=CARTESIAN_POINT('Ctrl Pts',(-1.43775916449653,2.88435646789259,-35.2783935120017));
#14725=CARTESIAN_POINT('Ctrl Pts',(-1.49602286287619,2.85478452125253,-35.2744067846416));
#14726=CARTESIAN_POINT('Ctrl Pts',(-1.53307580699154,2.83505873047486,-35.2718866794257));
#14727=CARTESIAN_POINT('Ctrl Pts',(-1.69266361320067,2.74605521466,-35.2610542109695));
#14728=CARTESIAN_POINT('Ctrl Pts',(-1.81098066855724,2.66951035423643,-35.2530755195169));
#14729=CARTESIAN_POINT('Ctrl Pts',(-2.04926574345631,2.49219545733055,-35.2363478372434));
#14730=CARTESIAN_POINT('Ctrl Pts',(-2.1676593229078,2.38993295839145,-35.2276277891041));
#14731=CARTESIAN_POINT('Ctrl Pts',(-2.34943678676138,2.20826123881373,-35.2128897675376));
#14732=CARTESIAN_POINT('Ctrl Pts',(-2.41732314180717,2.13373315065483,-35.2070227981109));
#14733=CARTESIAN_POINT('Ctrl Pts',(-2.51394033186439,2.01712429433846,-35.1979973165043));
#14734=CARTESIAN_POINT('Ctrl Pts',(-2.5453505841666,1.97734073746211,-35.1949434906091));
#14735=CARTESIAN_POINT('Ctrl Pts',(-2.60219508379396,1.90174288323518,-35.189176274664));
#14736=CARTESIAN_POINT('Ctrl Pts',(-2.62786078929637,1.86611699212361,-35.1864725945987));
#14737=CARTESIAN_POINT('Ctrl Pts',(-2.68462179330101,1.78383463048775,-35.18025415793));
#14738=CARTESIAN_POINT('Ctrl Pts',(-2.71524271338279,1.7368697589535,-35.176723101184));
#14739=CARTESIAN_POINT('Ctrl Pts',(-2.82841102645769,1.55298587523434,-35.162957664705));
#14740=CARTESIAN_POINT('Ctrl Pts',(-2.90194338697604,1.41081077965373,-35.1524239716011));
#14741=CARTESIAN_POINT('Ctrl Pts',(-3.02672111244333,1.11810393665668,-35.1311116787717));
#14742=CARTESIAN_POINT('Ctrl Pts',(-3.07800034025221,0.968045029552722,
-35.1203664802707));
#14743=CARTESIAN_POINT('Ctrl Pts',(-3.13888207863788,0.735072530136991,
-35.10435627566));
#14744=CARTESIAN_POINT('Ctrl Pts',(-3.15665756691841,0.654543679398243,
-35.0989424729181));
#14745=CARTESIAN_POINT('Ctrl Pts',(-3.17709247811663,0.541526666860606,
-35.091584894491));
#14746=CARTESIAN_POINT('Ctrl Pts',(-3.18237742946235,0.509550616572541,
-35.0895297597963));
#14747=CARTESIAN_POINT('Ctrl Pts',(-3.19088423345794,0.452769939489621,
-35.0859336285606));
#14748=CARTESIAN_POINT('Ctrl Pts',(-3.19430103518963,0.42799974433517,-35.0843832261971));
#14749=CARTESIAN_POINT('Ctrl Pts',(-3.2017677143166,0.368786485915752,-35.0807192467316));
#14750=CARTESIAN_POINT('Ctrl Pts',(-3.20555056969504,0.33431382764763,-35.0786193530487));
#14751=CARTESIAN_POINT('Ctrl Pts',(-3.21813227936215,0.199644456009511,
-35.0705221942678));
#14752=CARTESIAN_POINT('Ctrl Pts',(-3.22279592866093,0.0991116701523034,
-35.0647053698551));
#14753=CARTESIAN_POINT('Ctrl Pts',(-3.22268034131199,-0.152185129279559,
-35.0503857923619));
#14754=CARTESIAN_POINT('Ctrl Pts',(-3.21204041784068,-0.302700064493506,
-35.0420003717722));
#14755=CARTESIAN_POINT('Ctrl Pts',(-3.17690790664443,-0.550762571349196,
-35.0278440136735));
#14756=CARTESIAN_POINT('Ctrl Pts',(-3.15832478350957,-0.648896053149135,
-35.0221561023034));
#14757=CARTESIAN_POINT('Ctrl Pts',(-3.1173656588011,-0.821034149274176,
-35.0118733855988));
#14758=CARTESIAN_POINT('Ctrl Pts',(-3.09682641937535,-0.895394074366066,
-35.0073280223274));
#14759=CARTESIAN_POINT('Ctrl Pts',(-3.05954018946172,-1.01367203911393,
-34.9998867429761));
#14760=CARTESIAN_POINT('Ctrl Pts',(-3.04446522857545,-1.05808709620345,
-34.997043490985));
#14761=CARTESIAN_POINT('Ctrl Pts',(-3.0129936634984,-1.14456247841059,-34.9914028999584));
#14762=CARTESIAN_POINT('Ctrl Pts',(-2.99667191798091,-1.18663860559836,
-34.9886085216076));
#14763=CARTESIAN_POINT('Ctrl Pts',(-2.954132665167,-1.28982081289588,-34.9816258636257));
#14764=CARTESIAN_POINT('Ctrl Pts',(-2.92689832369941,-1.35048240710605,
-34.9774052862986));
#14765=CARTESIAN_POINT('Ctrl Pts',(-2.86273139085445,-1.48233338362255,
-34.9679685814317));
#14766=CARTESIAN_POINT('Ctrl Pts',(-2.82497888557456,-1.55307310185483,
-34.9627293401044));
#14767=CARTESIAN_POINT('Ctrl Pts',(-2.68034599700982,-1.80132697538337,
-34.9437270797267));
#14768=CARTESIAN_POINT('Ctrl Pts',(-2.55904553647452,-1.9698505967047,-34.9296189284839));
#14769=CARTESIAN_POINT('Ctrl Pts',(-2.36499114692388,-2.19100837949097,
-34.9100136975336));
#14770=CARTESIAN_POINT('Ctrl Pts',(-2.30492239037816,-2.25411534085376,
-34.9042789500282));
#14771=CARTESIAN_POINT('Ctrl Pts',(-2.21842303076359,-2.33791106277472,
-34.8965486938852));
#14772=CARTESIAN_POINT('Ctrl Pts',(-2.19411981155172,-2.36073449081934,
-34.8944305826072));
#14773=CARTESIAN_POINT('Ctrl Pts',(-2.15099360866885,-2.39999334233975,
-34.8907714930869));
#14774=CARTESIAN_POINT('Ctrl Pts',(-2.13232694087042,-2.41659336063151,
-34.8892196429684));
#14775=CARTESIAN_POINT('Ctrl Pts',(-2.08851885528587,-2.45464837643007,
-34.8856508181931));
#14776=CARTESIAN_POINT('Ctrl Pts',(-2.06323749636522,-2.47593636625069,
-34.8836449300139));
#14777=CARTESIAN_POINT('Ctrl Pts',(-1.96944395792036,-2.55248003043506,
-34.8763783696987));
#14778=CARTESIAN_POINT('Ctrl Pts',(-1.89899923460882,-2.60531537463542,
-34.8712553214422));
#14779=CARTESIAN_POINT('Ctrl Pts',(-1.67611131819944,-2.75863657529509,
-34.8557534295035));
#14780=CARTESIAN_POINT('Ctrl Pts',(-1.51723033107526,-2.84911242478676,
-34.8456478666228));
#14781=CARTESIAN_POINT('Ctrl Pts',(-1.2325763064649,-2.98061166511535,-34.8278787439843));
#14782=CARTESIAN_POINT('Ctrl Pts',(-1.1103813351518,-3.02825673617044,-34.8203512212046));
#14783=CARTESIAN_POINT('Ctrl Pts',(-0.932573740909747,-3.08537348604897,
-34.8092942211876));
#14784=CARTESIAN_POINT('Ctrl Pts',(-0.879084006879159,-3.10103758323379,
-34.8059561050844));
#14785=CARTESIAN_POINT('Ctrl Pts',(-0.782864059520709,-3.12652540206666,
-34.7999154501342));
#14786=CARTESIAN_POINT('Ctrl Pts',(-0.740288127713118,-3.13687909008653,
-34.7972302707906));
#14787=CARTESIAN_POINT('Ctrl Pts',(-0.647168477502677,-3.15752275776517,
-34.7913248161217));
#14788=CARTESIAN_POINT('Ctrl Pts',(-0.596562834274296,-3.16747364816955,
-34.7880948161093));
#14789=CARTESIAN_POINT('Ctrl Pts',(-0.440220340477743,-3.19433674738178,
-34.778045163548));
#14790=CARTESIAN_POINT('Ctrl Pts',(-0.333870324497253,-3.20719627244352,
-34.7711075457247));
#14791=CARTESIAN_POINT('Ctrl Pts',(-0.0511483941743684,-3.22716748116875,
-34.7524223410741));
#14792=CARTESIAN_POINT('Ctrl Pts',(0.125504346323852,-3.22513059804636,
-34.7404856274706));
#14793=CARTESIAN_POINT('Ctrl Pts',(0.423597963677889,-3.19715860171786,
-34.7203725358168));
#14794=CARTESIAN_POINT('Ctrl Pts',(0.545359649590148,-3.17865479436919,
-34.7121725513879));
#14795=CARTESIAN_POINT('Ctrl Pts',(0.701251356756557,-3.14573979964565,
-34.7019096268518));
#14796=CARTESIAN_POINT('Ctrl Pts',(0.736602010426943,-3.13765040836752,
-34.6995986467861));
#14797=CARTESIAN_POINT('Ctrl Pts',(0.796196375762298,-3.1229504894476,-34.6957388020278));
#14798=CARTESIAN_POINT('Ctrl Pts',(0.820511722950976,-3.11665029869525,
-34.6941745124122));
#14799=CARTESIAN_POINT('Ctrl Pts',(0.874901520807166,-3.10187699040634,
-34.6907004487907));
#14800=CARTESIAN_POINT('Ctrl Pts',(0.904930385116731,-3.09324986082381,
-34.6887988009628));
#14801=CARTESIAN_POINT('Ctrl Pts',(1.00506989321956,-3.06289714638004,-34.6824978952339));
#14802=CARTESIAN_POINT('Ctrl Pts',(1.07456692700322,-3.03921238262024,-34.6781921643721));
#14803=CARTESIAN_POINT('Ctrl Pts',(1.26162385029788,-2.96824290739178,-34.6666382961886));
#14804=CARTESIAN_POINT('Ctrl Pts',(1.37730259368907,-2.91636784184618,-34.6595293006397));
#14805=CARTESIAN_POINT('Ctrl Pts',(1.65502558558038,-2.77160515790573,-34.6419265578614));
#14806=CARTESIAN_POINT('Ctrl Pts',(1.81260872761203,-2.67120698321779,-34.6314373418852));
#14807=CARTESIAN_POINT('Ctrl Pts',(2.01120362071568,-2.51897593697931,-34.6167429855911));
#14808=CARTESIAN_POINT('Ctrl Pts',(2.06062351542123,-2.47871130162602,-34.6129523952937));
#14809=CARTESIAN_POINT('Ctrl Pts',(2.14262412661997,-2.40775380598445,-34.6064062785327));
#14810=CARTESIAN_POINT('Ctrl Pts',(2.17581945505171,-2.37779854808404,-34.6036803003651));
#14811=CARTESIAN_POINT('Ctrl Pts',(2.22876678606824,-2.32798190370282,-34.5992011997548));
#14812=CARTESIAN_POINT('Ctrl Pts',(2.24890195437326,-2.30853654037346,-34.597465658131));
#14813=CARTESIAN_POINT('Ctrl Pts',(2.26878020184338,-2.28883244433128,-34.5957191253299));
#14814=CARTESIAN_POINT('Origin',(0.,0.,-41.3107734492731));
#14815=CARTESIAN_POINT('',(2.26878017716708,-2.2888324687914,-33.0953665650246));
#14816=CARTESIAN_POINT('',(2.26878022243768,-2.28883242391741,-33.3405291647262));
#14817=CARTESIAN_POINT('',(2.26878020078428,-2.2888324453811,-41.3107734492731));
#14818=CARTESIAN_POINT('Ctrl Pts',(2.26878017716708,-2.2888324687914,-33.0953665650246));
#14819=CARTESIAN_POINT('Ctrl Pts',(2.25513518290648,-2.30235792026857,-33.0966503519412));
#14820=CARTESIAN_POINT('Ctrl Pts',(2.2413678000685,-2.31576278083686,-33.0979366661943));
#14821=CARTESIAN_POINT('Ctrl Pts',(2.08286720356223,-2.46735143037641,-33.1126403973839));
#14822=CARTESIAN_POINT('Ctrl Pts',(1.92568569537045,-2.59189080711268,-33.1262646258381));
#14823=CARTESIAN_POINT('Ctrl Pts',(1.71620807102168,-2.72822831962593,-33.1425841306978));
#14824=CARTESIAN_POINT('Ctrl Pts',(1.67382313920823,-2.75443580311782,-33.1457987636766));
#14825=CARTESIAN_POINT('Ctrl Pts',(1.60723780360399,-2.79350198703619,-33.1506960970612));
#14826=CARTESIAN_POINT('Ctrl Pts',(1.58345400366048,-2.80705187850117,-33.1524160342899));
#14827=CARTESIAN_POINT('Ctrl Pts',(1.53898885258495,-2.83163913499436,-33.1555734248723));
#14828=CARTESIAN_POINT('Ctrl Pts',(1.51835455793478,-2.84275682615637,-33.1570157123206));
#14829=CARTESIAN_POINT('Ctrl Pts',(1.46004330051404,-2.87335868486747,-33.1610326168507));
#14830=CARTESIAN_POINT('Ctrl Pts',(1.42209890099693,-2.89232634112015,-33.1635782642917));
#14831=CARTESIAN_POINT('Ctrl Pts',(1.19693712200369,-2.9993774020375,-33.1783503480835));
#14832=CARTESIAN_POINT('Ctrl Pts',(1.00194484908313,-3.07002406313783,-33.1898287210299));
#14833=CARTESIAN_POINT('Ctrl Pts',(0.689959120139942,-3.15013294156086,
-33.2079601832759));
#14834=CARTESIAN_POINT('Ctrl Pts',(0.576959686460083,-3.17277426477144,
-33.2144772147706));
#14835=CARTESIAN_POINT('Ctrl Pts',(0.379353359645486,-3.20146093324465,
-33.226026467992));
#14836=CARTESIAN_POINT('Ctrl Pts',(0.295271051875767,-3.21030752864928,
-33.2309868774288));
#14837=CARTESIAN_POINT('Ctrl Pts',(0.162899144393818,-3.2189904552102,-33.2389267232889));
#14838=CARTESIAN_POINT('Ctrl Pts',(0.114792996079793,-3.22106471252725,
-33.2418388482718));
#14839=CARTESIAN_POINT('Ctrl Pts',(0.0221571438913656,-3.22298122841051,
-33.2475067653327));
#14840=CARTESIAN_POINT('Ctrl Pts',(-0.0223584445544171,-3.22297979085081,
-33.2502571432136));
#14841=CARTESIAN_POINT('Ctrl Pts',(-0.129180639200564,-3.22076321688906,
-33.2569269144018));
#14842=CARTESIAN_POINT('Ctrl Pts',(-0.19144893514027,-3.21766216524124,
-33.260872081195));
#14843=CARTESIAN_POINT('Ctrl Pts',(-0.500463146355082,-3.19327147973357,
-33.280747707219));
#14844=CARTESIAN_POINT('Ctrl Pts',(-0.74424233835898,-3.14539570446211,
-33.2974621844789));
#14845=CARTESIAN_POINT('Ctrl Pts',(-1.06486340831942,-3.04304161805856,
-33.3200897644635));
#14846=CARTESIAN_POINT('Ctrl Pts',(-1.14848303963809,-3.01247814227129,
-33.326043727433));
#14847=CARTESIAN_POINT('Ctrl Pts',(-1.28564488330281,-2.95580189397782,
-33.3358000483637));
#14848=CARTESIAN_POINT('Ctrl Pts',(-1.33992168706782,-2.93159656184382,
-33.3396576959825));
#14849=CARTESIAN_POINT('Ctrl Pts',(-1.41973569084597,-2.89332242051299,
-33.3452948122007));
#14850=CARTESIAN_POINT('Ctrl Pts',(-1.44579942754109,-2.88038681751157,
-33.3471298171583));
#14851=CARTESIAN_POINT('Ctrl Pts',(-1.49425773645198,-2.85551311160995,
-33.3505256595042));
#14852=CARTESIAN_POINT('Ctrl Pts',(-1.51669230236408,-2.84366063445182,
-33.3520908203042));
#14853=CARTESIAN_POINT('Ctrl Pts',(-1.57430094990484,-2.81234950173778,
-33.3560966624343));
#14854=CARTESIAN_POINT('Ctrl Pts',(-1.6092563386829,-2.79249486374002,-33.3585146658838));
#14855=CARTESIAN_POINT('Ctrl Pts',(-1.82412891528854,-2.66507213151402,
-33.3733559610289));
#14856=CARTESIAN_POINT('Ctrl Pts',(-1.99358372486125,-2.54080677522296,
-33.3849861482271));
#14857=CARTESIAN_POINT('Ctrl Pts',(-2.23625067278748,-2.32352576272029,
-33.4033187248563));
#14858=CARTESIAN_POINT('Ctrl Pts',(-2.31847104350024,-2.2414903350086,-33.4098842228074));
#14859=CARTESIAN_POINT('Ctrl Pts',(-2.45287922393343,-2.09205970325972,
-33.4215062511335));
#14860=CARTESIAN_POINT('Ctrl Pts',(-2.50715246175046,-2.02670055657058,
-33.4264895332933));
#14861=CARTESIAN_POINT('Ctrl Pts',(-2.58808962786105,-1.92099821046018,
-33.4344567627992));
#14862=CARTESIAN_POINT('Ctrl Pts',(-2.61653682317474,-1.88206714287472,
-33.4373725435977));
#14863=CARTESIAN_POINT('Ctrl Pts',(-2.66953166546536,-1.80601692018826,
-33.4430422083021));
#14864=CARTESIAN_POINT('Ctrl Pts',(-2.69420492630011,-1.76899856958464,
-33.4457905525562));
#14865=CARTESIAN_POINT('Ctrl Pts',(-2.75149098626182,-1.67907020052297,
-33.4524458217324));
#14866=CARTESIAN_POINT('Ctrl Pts',(-2.78335387907905,-1.62570592191355,
-33.456378228878));
#14867=CARTESIAN_POINT('Ctrl Pts',(-2.91939440476421,-1.38212886629318,
-33.4742641091173));
#14868=CARTESIAN_POINT('Ctrl Pts',(-3.00574296928829,-1.18263609477538,
-33.4887959230864));
#14869=CARTESIAN_POINT('Ctrl Pts',(-3.10430948207055,-0.872460667001341,
-33.5107168227683));
#14870=CARTESIAN_POINT('Ctrl Pts',(-3.13196075265785,-0.767299589019079,
-33.5180289730792));
#14871=CARTESIAN_POINT('Ctrl Pts',(-3.16803231808227,-0.595152646469083,
-33.5296436145815));
#14872=CARTESIAN_POINT('Ctrl Pts',(-3.17975668556551,-0.528946243713139,
-33.534026750248));
#14873=CARTESIAN_POINT('Ctrl Pts',(-3.19375641491715,-0.432386762982047,
-33.5402554593491));
#14874=CARTESIAN_POINT('Ctrl Pts',(-3.19768623877609,-0.402294951309812,
-33.5421736250841));
#14875=CARTESIAN_POINT('Ctrl Pts',(-3.20411008306368,-0.347037924226917,
-33.5456485452067));
#14876=CARTESIAN_POINT('Ctrl Pts',(-3.20673379298496,-0.321893095036145,
-33.5472113168359));
#14877=CARTESIAN_POINT('Ctrl Pts',(-3.21253877950483,-0.259110989934605,
-33.5510708370597));
#14878=CARTESIAN_POINT('Ctrl Pts',(-3.21535482197858,-0.221444261801844,
-33.5533490151824));
#14879=CARTESIAN_POINT('Ctrl Pts',(-3.22945337670295,0.0254451694556208,
-33.5680870235743));
#14880=CARTESIAN_POINT('Ctrl Pts',(-3.22097239020679,0.235316330868668,
-33.5797260394388));
#14881=CARTESIAN_POINT('Ctrl Pts',(-3.17582410463868,0.560721496509795,
-33.5982081408355));
#14882=CARTESIAN_POINT('Ctrl Pts',(-3.15296643102383,0.677545446060423,
-33.6049291498048));
#14883=CARTESIAN_POINT('Ctrl Pts',(-3.10249245064262,0.876409154352357,
-33.6167840495007));
#14884=CARTESIAN_POINT('Ctrl Pts',(-3.07793584415687,0.959094160048735,
-33.6218400001516));
#14885=CARTESIAN_POINT('Ctrl Pts',(-3.03445719448557,1.08652300457852,-33.6298945094339));
#14886=CARTESIAN_POINT('Ctrl Pts',(-3.01778886182617,1.13199501612168,-33.6328221668055));
#14887=CARTESIAN_POINT('Ctrl Pts',(-2.98388351142591,1.21841241530387,-33.6384984716431));
#14888=CARTESIAN_POINT('Ctrl Pts',(-2.96681197181193,1.25941099101307,-33.6412411915081));
#14889=CARTESIAN_POINT('Ctrl Pts',(-2.92405979523054,1.35638620065473,-33.6478540497705));
#14890=CARTESIAN_POINT('Ctrl Pts',(-2.8976118914326,1.41200344714246,-33.6517488044581));
#14891=CARTESIAN_POINT('Ctrl Pts',(-2.76844559137495,1.66469468424587,-33.6699325423795));
#14892=CARTESIAN_POINT('Ctrl Pts',(-2.64712144118443,1.85154547174523,-33.6848360126741));
#14893=CARTESIAN_POINT('Ctrl Pts',(-2.44097011282467,2.10689897326052,-33.7069385796269));
#14894=CARTESIAN_POINT('Ctrl Pts',(-2.37033777372358,2.18606016015702,-33.7140683960266));
#14895=CARTESIAN_POINT('Ctrl Pts',(-2.24944774491906,2.30878529938712,-33.725438123356));
#14896=CARTESIAN_POINT('Ctrl Pts',(-2.20151919041601,2.3545316288309,-33.7297551558329));
#14897=CARTESIAN_POINT('Ctrl Pts',(-2.12973675486259,2.41893585094417,-33.7359100645792));
#14898=CARTESIAN_POINT('Ctrl Pts',(-2.10697867246153,2.43878460029075,-33.7378182854353));
#14899=CARTESIAN_POINT('Ctrl Pts',(-2.06463143179795,2.47468293264917,-33.7412853495083));
#14900=CARTESIAN_POINT('Ctrl Pts',(-2.0451278329901,2.49082531496769,-33.7428499550626));
#14901=CARTESIAN_POINT('Ctrl Pts',(-1.99583681753157,2.53065226290494,-33.7467281503791));
#14902=CARTESIAN_POINT('Ctrl Pts',(-1.96581671579061,2.55404197318377,-33.7490227186743));
#14903=CARTESIAN_POINT('Ctrl Pts',(-1.76990160376916,2.70118481668855,-33.7636196026392));
#14904=CARTESIAN_POINT('Ctrl Pts',(-1.59280807428144,2.80925847559134,-33.775124693466));
#14905=CARTESIAN_POINT('Ctrl Pts',(-1.29851769894735,2.95201420267694,-33.7935234837422));
#14906=CARTESIAN_POINT('Ctrl Pts',(-1.18764046013171,2.99834020625426,-33.8003050504581));
#14907=CARTESIAN_POINT('Ctrl Pts',(-0.992679404864649,3.06728320257979,
-33.8122502858677));
#14908=CARTESIAN_POINT('Ctrl Pts',(-0.90978865695149,3.09288238958538,-33.817334151159));
#14909=CARTESIAN_POINT('Ctrl Pts',(-0.779082383471197,3.12753917872972,
-33.8254222140341));
#14910=CARTESIAN_POINT('Ctrl Pts',(-0.731921029369964,3.13891094270284,
-33.8283544495412));
#14911=CARTESIAN_POINT('Ctrl Pts',(-0.641154254754654,3.15864028930871,
-33.8340334998117));
#14912=CARTESIAN_POINT('Ctrl Pts',(-0.597597393427313,3.16716976312302,
-33.8367742410062));
#14913=CARTESIAN_POINT('Ctrl Pts',(-0.493423269460232,3.18534414007337,
-33.8433717220453));
#14914=CARTESIAN_POINT('Ctrl Pts',(-0.432681166047868,3.19416186606653,
-33.8472527628742));
#14915=CARTESIAN_POINT('Ctrl Pts',(-0.149161112198021,3.22708416691309,
-33.8655376640036));
#14916=CARTESIAN_POINT('Ctrl Pts',(0.0754645436143387,3.2296437681523,-33.8805687433087));
#14917=CARTESIAN_POINT('Ctrl Pts',(0.403194128887664,3.19915728413175,-33.9027352765442));
#14918=CARTESIAN_POINT('Ctrl Pts',(0.507351232064744,3.18430045068996,-33.9098043918657));
#14919=CARTESIAN_POINT('Ctrl Pts',(0.675310769280718,3.15189092876012,-33.9210922977994));
#14920=CARTESIAN_POINT('Ctrl Pts',(0.739628699154956,3.13742117910994,-33.9253870426276));
#14921=CARTESIAN_POINT('Ctrl Pts',(0.832654173036695,3.11347286267701,-33.9315170452971));
#14922=CARTESIAN_POINT('Ctrl Pts',(0.861740983126144,3.10554807926666,-33.9334218953873));
#14923=CARTESIAN_POINT('Ctrl Pts',(0.915057744129675,3.09021496704233,-33.9368863356755));
#14924=CARTESIAN_POINT('Ctrl Pts',(0.939317027293624,3.0829276306688,-33.9384516013507));
#14925=CARTESIAN_POINT('Ctrl Pts',(0.999895941088634,3.06394862010903,-33.9423363319439));
#14926=CARTESIAN_POINT('Ctrl Pts',(1.03609819125512,3.05189676473568,-33.944636617782));
#14927=CARTESIAN_POINT('Ctrl Pts',(1.26640816662163,2.97065489779202,-33.9591839687126));
#14928=CARTESIAN_POINT('Ctrl Pts',(1.45373681265877,2.88361731984841,-33.9706419824356));
#14929=CARTESIAN_POINT('Ctrl Pts',(1.73538184648514,2.71828648359193,-33.989011692974));
#14930=CARTESIAN_POINT('Ctrl Pts',(1.83577203909949,2.65152227255239,-33.9958146326008));
#14931=CARTESIAN_POINT('Ctrl Pts',(2.00173381057107,2.52719820325288,-34.0077916897256));
#14932=CARTESIAN_POINT('Ctrl Pts',(2.06914227549585,2.47231014881584,-34.0128853398841));
#14933=CARTESIAN_POINT('Ctrl Pts',(2.17061542892803,2.38262504125599,-34.0209851389862));
#14934=CARTESIAN_POINT('Ctrl Pts',(2.20625146237104,2.34966540946579,-34.0239189510395));
#14935=CARTESIAN_POINT('Ctrl Pts',(2.27301420244556,2.28505860344945,-34.0295989072626));
#14936=CARTESIAN_POINT('Ctrl Pts',(2.30425819509295,2.25354836950868,-34.0323389266786));
#14937=CARTESIAN_POINT('Ctrl Pts',(2.37709179606774,2.17699551326187,-34.0389309594077));
#14938=CARTESIAN_POINT('Ctrl Pts',(2.41806503719888,2.13139286732515,-34.0428071635249));
#14939=CARTESIAN_POINT('Ctrl Pts',(2.62198078357479,1.89098536190384,-34.0630007882741));
#14940=CARTESIAN_POINT('Ctrl Pts',(2.76276276864001,1.67860432457326,-34.0801548260348));
#14941=CARTESIAN_POINT('Ctrl Pts',(2.91618824585569,1.37458166249732,-34.1030404633608));
#14942=CARTESIAN_POINT('Ctrl Pts',(2.95209928004865,1.29566195351805,-34.1088344401637));
#14943=CARTESIAN_POINT('Ctrl Pts',(3.00681584290379,1.16128727718757,-34.1183663352648));
#14944=CARTESIAN_POINT('Ctrl Pts',(3.02737156840673,1.10659474388166,-34.1221567268739));
#14945=CARTESIAN_POINT('Ctrl Pts',(3.05586610072001,1.02402953427941,-34.1277172174223));
#14946=CARTESIAN_POINT('Ctrl Pts',(3.0649337319084,0.996561825332186,-34.1295408102141));
#14947=CARTESIAN_POINT('Ctrl Pts',(3.08127937266239,0.944712724952865,-34.132929152254));
#14948=CARTESIAN_POINT('Ctrl Pts',(3.08864049603775,0.920361137104176,-34.1344979240421));
#14949=CARTESIAN_POINT('Ctrl Pts',(3.10700725064891,0.856897969454276,-34.1385329862793));
#14950=CARTESIAN_POINT('Ctrl Pts',(3.11756338058618,0.817659519530494,-34.1409758948028));
#14951=CARTESIAN_POINT('Ctrl Pts',(3.17137297685285,0.601421648596455,-34.1542071474229));
#14952=CARTESIAN_POINT('Ctrl Pts',(3.20030223372359,0.42118159973948,-34.1644049639806));
#14953=CARTESIAN_POINT('Ctrl Pts',(3.22833380326741,0.044943813274584,-34.1856104600273));
#14954=CARTESIAN_POINT('Ctrl Pts',(3.22513769176329,-0.150454589831461,
-34.1965927607226));
#14955=CARTESIAN_POINT('Ctrl Pts',(3.19802443635561,-0.402748389013214,
-34.2115663513047));
#14956=CARTESIAN_POINT('Ctrl Pts',(3.19015460947218,-0.460954984497453,
-34.2150739233834));
#14957=CARTESIAN_POINT('Ctrl Pts',(3.17360407226503,-0.562402487549828,
-34.2212980813588));
#14958=CARTESIAN_POINT('Ctrl Pts',(3.16561782684986,-0.605741569158405,
-34.2239928290579));
#14959=CARTESIAN_POINT('Ctrl Pts',(3.14673698999318,-0.697592153456303,
-34.2297864905141));
#14960=CARTESIAN_POINT('Ctrl Pts',(3.13560345814871,-0.746042239054158,
-34.2328921878864));
#14961=CARTESIAN_POINT('Ctrl Pts',(3.10012521323423,-0.885565348201471,
-34.2419870469939));
#14962=CARTESIAN_POINT('Ctrl Pts',(3.0729014764931,-0.975846361725071,-34.2480624936056));
#14963=CARTESIAN_POINT('Ctrl Pts',(2.97018489822096,-1.26927235750758,-34.2684345690076));
#14964=CARTESIAN_POINT('Ctrl Pts',(2.87817451151786,-1.46599696375291,-34.2831536722957));
#14965=CARTESIAN_POINT('Ctrl Pts',(2.72987057081456,-1.71441278346529,-34.3025244865525));
#14966=CARTESIAN_POINT('Ctrl Pts',(2.69049452599039,-1.77556886134533,-34.307357908211));
#14967=CARTESIAN_POINT('Ctrl Pts',(2.61946673923537,-1.87808832109708,-34.3155152062688));
#14968=CARTESIAN_POINT('Ctrl Pts',(2.58881986581317,-1.92011304333786,-34.3188755942587));
#14969=CARTESIAN_POINT('Ctrl Pts',(2.54026067673939,-1.98342253963959,-34.32394215152));
#14970=CARTESIAN_POINT('Ctrl Pts',(2.523068802453,-2.00524642394919,-34.3256894551054));
#14971=CARTESIAN_POINT('Ctrl Pts',(2.48900094624645,-2.04736125880574,-34.3290584325427));
#14972=CARTESIAN_POINT('Ctrl Pts',(2.4721540476785,-2.06767218408784,-34.3306815511669));
#14973=CARTESIAN_POINT('Ctrl Pts',(2.42614866163923,-2.12177091478953,-34.3350071039688));
#14974=CARTESIAN_POINT('Ctrl Pts',(2.39653352839163,-2.15516510292579,-34.3376797757416));
#14975=CARTESIAN_POINT('Ctrl Pts',(2.33447250556559,-2.22228355789538,-34.3430826064246));
#14976=CARTESIAN_POINT('Ctrl Pts',(2.30198005379905,-2.25592345578822,-34.3458075242752));
#14977=CARTESIAN_POINT('Ctrl Pts',(2.2687801086558,-2.28883253670245,-34.3485046109761));
#14978=CARTESIAN_POINT('Ctrl Pts',(2.26878020184338,-2.28883244433128,-34.5957191253299));
#14979=CARTESIAN_POINT('Ctrl Pts',(2.28275431418291,-2.2749807578556,-34.5944913387453));
#14980=CARTESIAN_POINT('Ctrl Pts',(2.29660145941807,-2.26100120851142,-34.5932581244753));
#14981=CARTESIAN_POINT('Ctrl Pts',(2.36726430182595,-2.18834372672855,-34.586878066658));
#14982=CARTESIAN_POINT('Ctrl Pts',(2.42195799566748,-2.12765274332109,-34.5816453573719));
#14983=CARTESIAN_POINT('Ctrl Pts',(2.54417663641725,-1.98120703338518,-34.5692349639376));
#14984=CARTESIAN_POINT('Ctrl Pts',(2.60976706956622,-1.89397168328745,-34.5620004317896));
#14985=CARTESIAN_POINT('Ctrl Pts',(2.79533776067639,-1.61917284960125,-34.5397859401555));
#14986=CARTESIAN_POINT('Ctrl Pts',(2.90043913069693,-1.4223549679812,-34.5245974973487));
#14987=CARTESIAN_POINT('Ctrl Pts',(2.99954093615506,-1.17918438778175,-34.5076072903031));
#14988=CARTESIAN_POINT('Ctrl Pts',(3.01396438259134,-1.14181464329064,-34.5050443534769));
#14989=CARTESIAN_POINT('Ctrl Pts',(3.03637307326663,-1.08036968935533,-34.5009189546891));
#14990=CARTESIAN_POINT('Ctrl Pts',(3.04477716846044,-1.05645268169334,-34.4993349144063));
#14991=CARTESIAN_POINT('Ctrl Pts',(3.06223732723952,-1.0048232888163,-34.4959648378351));
#14992=CARTESIAN_POINT('Ctrl Pts',(3.07120112559852,-0.977082942840127,
-34.4941836577518));
#14993=CARTESIAN_POINT('Ctrl Pts',(3.09738594297763,-0.8921254334767,-34.4888076273285));
#14994=CARTESIAN_POINT('Ctrl Pts',(3.11339410979983,-0.834545090850007,
-34.4852722970275));
#14995=CARTESIAN_POINT('Ctrl Pts',(3.14942446318477,-0.689421692088562,
-34.4765561336581));
#14996=CARTESIAN_POINT('Ctrl Pts',(3.16740718754507,-0.601423415670002,
-34.4714442047867));
#14997=CARTESIAN_POINT('Ctrl Pts',(3.22076408682028,-0.270358203708891,
-34.4524983364445));
#14998=CARTESIAN_POINT('Ctrl Pts',(3.23199925033774,-0.0242782529003616,
-34.4389161158309));
#14999=CARTESIAN_POINT('Ctrl Pts',(3.21089289386406,0.283218939623277,-34.420798660998));
#15000=CARTESIAN_POINT('Ctrl Pts',(3.204777719176,0.345608395335527,-34.4170678039333));
#15001=CARTESIAN_POINT('Ctrl Pts',(3.19120969630814,0.451977550233154,-34.4105907388083));
#15002=CARTESIAN_POINT('Ctrl Pts',(3.18465580620903,0.496054561874655,-34.4078724178608));
#15003=CARTESIAN_POINT('Ctrl Pts',(3.16914429757165,0.587322799796455,-34.402165523574));
#15004=CARTESIAN_POINT('Ctrl Pts',(3.16004132848768,0.634477790566203,-34.399173090636));
#15005=CARTESIAN_POINT('Ctrl Pts',(3.1321753072958,0.763291388460768,-34.3908712568216));
#15006=CARTESIAN_POINT('Ctrl Pts',(3.11127739106761,0.844444756922051,-34.3854982290444));
#15007=CARTESIAN_POINT('Ctrl Pts',(3.05466245178758,1.03346457621671,-34.3726437078281));
#15008=CARTESIAN_POINT('Ctrl Pts',(3.01635749649642,1.14043663225102,-34.3650989157743));
#15009=CARTESIAN_POINT('Ctrl Pts',(2.89105753980571,1.43955786079567,-34.3433455914678));
#15010=CARTESIAN_POINT('Ctrl Pts',(2.79074818166118,1.62550672723553,-34.3289864507506));
#15011=CARTESIAN_POINT('Ctrl Pts',(2.6495864078017,1.83509281791907,-34.3126045728813));
#15012=CARTESIAN_POINT('Ctrl Pts',(2.62549859376958,1.86939329465406,-34.3099181087708));
#15013=CARTESIAN_POINT('Ctrl Pts',(2.58695372173706,1.92206491913183,-34.3057959308746));
#15014=CARTESIAN_POINT('Ctrl Pts',(2.57295494921852,1.94076429396683,-34.3043331370721));
#15015=CARTESIAN_POINT('Ctrl Pts',(2.54202307249814,1.98115964575032,-34.3011774570349));
#15016=CARTESIAN_POINT('Ctrl Pts',(2.52501288363555,2.00279427357257,-34.2994899195145));
#15017=CARTESIAN_POINT('Ctrl Pts',(2.47594389590218,2.06358424694428,-34.2947471245486));
#15018=CARTESIAN_POINT('Ctrl Pts',(2.44323596504014,2.10220758666463,-34.291732436312));
#15019=CARTESIAN_POINT('Ctrl Pts',(2.36324269945501,2.19227766636083,-34.2846555737673));
#15020=CARTESIAN_POINT('Ctrl Pts',(2.31516683158788,2.24298929271774,-34.2806329062166));
#15021=CARTESIAN_POINT('Ctrl Pts',(2.17117198606978,2.38531167123716,-34.2690959575433));
#15022=CARTESIAN_POINT('Ctrl Pts',(2.07120086263719,2.47261566851285,-34.2616972355133));
#15023=CARTESIAN_POINT('Ctrl Pts',(1.84893457844744,2.64375441405337,-34.245889239122));
#15024=CARTESIAN_POINT('Ctrl Pts',(1.72567168717498,2.72581148782508,-34.2374775909167));
#15025=CARTESIAN_POINT('Ctrl Pts',(1.54303214809534,2.8300284839086,-34.2251136782484));
#15026=CARTESIAN_POINT('Ctrl Pts',(1.48796449225416,2.85936537673015,-34.2213994116818));
#15027=CARTESIAN_POINT('Ctrl Pts',(1.39220167180797,2.90686668046207,-34.214941439447));
#15028=CARTESIAN_POINT('Ctrl Pts',(1.35191665529052,2.92581962045885,-34.2122251630985));
#15029=CARTESIAN_POINT('Ctrl Pts',(1.26729144825611,2.96351244704122,-34.2065135033633));
#15030=CARTESIAN_POINT('Ctrl Pts',(1.22289832365684,2.98210545429801,-34.2035140689117));
#15031=CARTESIAN_POINT('Ctrl Pts',(1.09954829213986,3.03055020943928,-34.1951647056184));
#15032=CARTESIAN_POINT('Ctrl Pts',(1.01981364412113,3.0583033140502,-34.1897498793646));
#15033=CARTESIAN_POINT('Ctrl Pts',(0.829162615932968,3.1163779454646,-34.1767612468011));
#15034=CARTESIAN_POINT('Ctrl Pts',(0.717533976910228,3.14395667563413,-34.1691221166082));
#15035=CARTESIAN_POINT('Ctrl Pts',(0.40222596419993,3.20418703644321,-34.1475825410917));
#15036=CARTESIAN_POINT('Ctrl Pts',(0.196524080880937,3.22335002034519,-34.1335495640038));
#15037=CARTESIAN_POINT('Ctrl Pts',(-0.052682124323602,3.22260730248037,
-34.1173746297146));
#15038=CARTESIAN_POINT('Ctrl Pts',(-0.0957549019505773,3.22161522101677,
-34.1146102318553));
#15039=CARTESIAN_POINT('Ctrl Pts',(-0.16231880035045,3.21874579136757,-34.110399184628));
#15040=CARTESIAN_POINT('Ctrl Pts',(-0.185829663757392,3.2174740539212,-34.1089236108247));
#15041=CARTESIAN_POINT('Ctrl Pts',(-0.236461362457809,3.21417844340634,
-34.1057743210566));
#15042=CARTESIAN_POINT('Ctrl Pts',(-0.26357495516198,3.21206871083601,-34.1041053832965));
#15043=CARTESIAN_POINT('Ctrl Pts',(-0.339344344231211,3.20520710941833,
-34.099482596997));
#15044=CARTESIAN_POINT('Ctrl Pts',(-0.387925230829476,3.19969088509346,
-34.0965660987336));
#15045=CARTESIAN_POINT('Ctrl Pts',(-0.502188986630655,3.18407562230666,
-34.089779905838));
#15046=CARTESIAN_POINT('Ctrl Pts',(-0.56772303409955,3.17304629658005,-34.0859453745583));
#15047=CARTESIAN_POINT('Ctrl Pts',(-0.855798812563382,3.11535158528491,
-34.0691696744409));
#15048=CARTESIAN_POINT('Ctrl Pts',(-1.07337376811176,3.04724139140263,-34.0566663210387));
#15049=CARTESIAN_POINT('Ctrl Pts',(-1.36892210851935,2.91910105586133,-34.0381393677788));
#15050=CARTESIAN_POINT('Ctrl Pts',(-1.45415905513403,2.8775889106468,-34.0326061313529));
#15051=CARTESIAN_POINT('Ctrl Pts',(-1.58119510274997,2.80863283045792,-34.0239792737522));
#15052=CARTESIAN_POINT('Ctrl Pts',(-1.62439350654731,2.78387170367313,-34.0209756936361));
#15053=CARTESIAN_POINT('Ctrl Pts',(-1.70469883702285,2.73533542090594,-34.0152483054809));
#15054=CARTESIAN_POINT('Ctrl Pts',(-1.74192566316203,2.7117803522099,-34.0125327577926));
#15055=CARTESIAN_POINT('Ctrl Pts',(-1.82750560302044,2.65514072525237,-34.0061415400768));
#15056=CARTESIAN_POINT('Ctrl Pts',(-1.87546132461454,2.62148681582104,-34.0024457566313));
#15057=CARTESIAN_POINT('Ctrl Pts',(-2.080601206629,2.46901498075038,-33.9861170325249));
#15058=CARTESIAN_POINT('Ctrl Pts',(-2.22759875855569,2.33724623802432,-33.9730072397113));
#15059=CARTESIAN_POINT('Ctrl Pts',(-2.48438253152257,2.06070523692144,-33.9476082426829));
#15060=CARTESIAN_POINT('Ctrl Pts',(-2.59582690327688,1.91842473082648,-33.9353960022716));
#15061=CARTESIAN_POINT('Ctrl Pts',(-2.71712523652305,1.73349571666927,-33.9210757626383));
#15062=CARTESIAN_POINT('Ctrl Pts',(-2.73882054866971,1.69901127102594,-33.9184672845013));
#15063=CARTESIAN_POINT('Ctrl Pts',(-2.77300125182289,1.64232443867431,-33.914289962674));
#15064=CARTESIAN_POINT('Ctrl Pts',(-2.78588720453655,1.62036975938497,-33.9126984752009));
#15065=CARTESIAN_POINT('Ctrl Pts',(-2.8128363786728,1.57318252856204,-33.9093368337774));
#15066=CARTESIAN_POINT('Ctrl Pts',(-2.82682290460113,1.54790961139833,-33.9075710454565));
#15067=CARTESIAN_POINT('Ctrl Pts',(-2.86795106962706,1.47117594494492,-33.9023031580817));
#15068=CARTESIAN_POINT('Ctrl Pts',(-2.89404214267402,1.41916275888841,-33.8988571018703));
#15069=CARTESIAN_POINT('Ctrl Pts',(-2.95522847058906,1.28847165071172,-33.8904350533469));
#15070=CARTESIAN_POINT('Ctrl Pts',(-2.98860551890029,1.20903809799406,-33.8855220777578));
#15071=CARTESIAN_POINT('Ctrl Pts',(-3.10819065154371,0.889105337964295,
-33.8662019369981));
#15072=CARTESIAN_POINT('Ctrl Pts',(-3.16885482755945,0.640086550662371,
-33.8521041742066));
#15073=CARTESIAN_POINT('Ctrl Pts',(-3.20680935577038,0.325911580244707,
-33.8334735867785));
#15074=CARTESIAN_POINT('Ctrl Pts',(-3.21240728329331,0.265110069091308,
-33.8298347954596));
#15075=CARTESIAN_POINT('Ctrl Pts',(-3.21908421325108,0.15993865223235,-33.8234631443419));
#15076=CARTESIAN_POINT('Ctrl Pts',(-3.22097987681796,0.115636853831259,
-33.8207556495403));
#15077=CARTESIAN_POINT('Ctrl Pts',(-3.22303714865995,0.0226864077860033,
-33.8150192707975));
#15078=CARTESIAN_POINT('Ctrl Pts',(-3.22301242389749,-0.0259547603712082,
-33.8119854183815));
#15079=CARTESIAN_POINT('Ctrl Pts',(-3.21986202117663,-0.16206301649558,
-33.803399911913));
#15080=CARTESIAN_POINT('Ctrl Pts',(-3.2142745029355,-0.249425484656043,
-33.7977768863106));
#15081=CARTESIAN_POINT('Ctrl Pts',(-3.19241656248833,-0.457654033886757,
-33.7841069704923));
#15082=CARTESIAN_POINT('Ctrl Pts',(-3.17282901197651,-0.578033525436453,
-33.7759838996774));
#15083=CARTESIAN_POINT('Ctrl Pts',(-3.10258292516575,-0.895143215456569,
-33.7541575145555));
#15084=CARTESIAN_POINT('Ctrl Pts',(-3.04007265521266,-1.08870083126494,
-33.7403644121018));
#15085=CARTESIAN_POINT('Ctrl Pts',(-2.94453737792606,-1.31045766475141,
-33.7247686030642));
#15086=CARTESIAN_POINT('Ctrl Pts',(-2.92867229131383,-1.34554025187347,
-33.7223089290002));
#15087=CARTESIAN_POINT('Ctrl Pts',(-2.90131326193549,-1.4032614897725,-33.7182845471293));
#15088=CARTESIAN_POINT('Ctrl Pts',(-2.89017408583808,-1.42606289219463,
-33.7167009708395));
#15089=CARTESIAN_POINT('Ctrl Pts',(-2.86529347454357,-1.47550297645306,
-33.7132830934927));
#15090=CARTESIAN_POINT('Ctrl Pts',(-2.85144789365922,-1.50208548024471,
-33.7114547357917));
#15091=CARTESIAN_POINT('Ctrl Pts',(-2.80650730927186,-1.58550663512205,
-33.7057346359889));
#15092=CARTESIAN_POINT('Ctrl Pts',(-2.77406676565735,-1.64160570309285,
-33.7019141609664));
#15093=CARTESIAN_POINT('Ctrl Pts',(-2.68614632392249,-1.78358669658062,
-33.6922157819068));
#15094=CARTESIAN_POINT('Ctrl Pts',(-2.62823160448952,-1.8678769734824,-33.6864283693618));
#15095=CARTESIAN_POINT('Ctrl Pts',(-2.4270397116735,-2.13276511884671,-33.6676926112711));
#15096=CARTESIAN_POINT('Ctrl Pts',(-2.2684102164415,-2.30076402015599,-33.6548712654513));
#15097=CARTESIAN_POINT('Ctrl Pts',(-2.0471420065427,-2.48977932967462,-33.6377316381259));
#15098=CARTESIAN_POINT('Ctrl Pts',(-1.99995587692025,-2.52783846583439,
-33.6341175166604));
#15099=CARTESIAN_POINT('Ctrl Pts',(-1.91648719797233,-2.59136170038243,
-33.6277738680245));
#15100=CARTESIAN_POINT('Ctrl Pts',(-1.88069997615021,-2.61745027596987,
-33.6250690372428));
#15101=CARTESIAN_POINT('Ctrl Pts',(-1.80435382173455,-2.67073177051281,
-33.6193233923976));
#15102=CARTESIAN_POINT('Ctrl Pts',(-1.76369190480553,-2.6977567280764,-33.6162772918358));
#15103=CARTESIAN_POINT('Ctrl Pts',(-1.64751902048468,-2.77121904017934,
-33.607606639185));
#15104=CARTESIAN_POINT('Ctrl Pts',(-1.57068815370951,-2.81547692765836,
-33.6019083140625));
#15105=CARTESIAN_POINT('Ctrl Pts',(-1.38180571086802,-2.91414223076599,
-33.5879862187869));
#15106=CARTESIAN_POINT('Ctrl Pts',(-1.26823661294438,-2.96533027698748,
-33.5796820035108));
#15107=CARTESIAN_POINT('Ctrl Pts',(-0.967871025850895,-3.08029438539235,
-33.5580595436397));
#15108=CARTESIAN_POINT('Ctrl Pts',(-0.777653858128373,-3.13372799872132,
-33.5446731416994));
#15109=CARTESIAN_POINT('Ctrl Pts',(-0.545244104860971,-3.17653245338414,
-33.5293981784373));
#15110=CARTESIAN_POINT('Ctrl Pts',(-0.506622808517742,-3.182920546094,-33.5268957773784));
#15111=CARTESIAN_POINT('Ctrl Pts',(-0.442698106575825,-3.19230079895184,
-33.522823232662));
#15112=CARTESIAN_POINT('Ctrl Pts',(-0.417459350130495,-3.19569927649663,
-33.5212332291259));
#15113=CARTESIAN_POINT('Ctrl Pts',(-0.362735435088652,-3.20240856643265,
-33.517826954121));
#15114=CARTESIAN_POINT('Ctrl Pts',(-0.333240430192541,-3.20561204536868,
-33.5160160854558));
#15115=CARTESIAN_POINT('Ctrl Pts',(-0.241107852332009,-3.21433320843082,
-33.5104259638604));
#15116=CARTESIAN_POINT('Ctrl Pts',(-0.17834726898087,-3.21842574500099,
-33.5067134156217));
#15117=CARTESIAN_POINT('Ctrl Pts',(-0.0182121905898079,-3.22416866569615,
-33.497394937094));
#15118=CARTESIAN_POINT('Ctrl Pts',(0.0791922332697886,-3.2232477172368,
-33.4918707979789));
#15119=CARTESIAN_POINT('Ctrl Pts',(0.417629179523971,-3.20469421428213,
-33.4727600975917));
#15120=CARTESIAN_POINT('Ctrl Pts',(0.656576001985493,-3.16439225171484,
-33.4593506363506));
#15121=CARTESIAN_POINT('Ctrl Pts',(0.94565424611697,-3.08145381087424,-33.4416121788331));
#15122=CARTESIAN_POINT('Ctrl Pts',(1.00207374517393,-3.06357097315353,-33.4380792037024));
#15123=CARTESIAN_POINT('Ctrl Pts',(1.09963649348201,-3.02966388566108,-33.4318267754984));
#15124=CARTESIAN_POINT('Ctrl Pts',(1.14100304310047,-3.01432835661935,-33.4291298375298));
#15125=CARTESIAN_POINT('Ctrl Pts',(1.22807272407289,-2.98000055407047,-33.4233488529819));
#15126=CARTESIAN_POINT('Ctrl Pts',(1.27367895014745,-2.96079506688683,-33.4202583992583));
#15127=CARTESIAN_POINT('Ctrl Pts',(1.40349074996438,-2.90257503646365,-33.4112738339166));
#15128=CARTESIAN_POINT('Ctrl Pts',(1.48647173981525,-2.86096614691009,-33.4052967808635));
#15129=CARTESIAN_POINT('Ctrl Pts',(1.68509592767479,-2.75039495435885,-33.390411590174));
#15130=CARTESIAN_POINT('Ctrl Pts',(1.79843350213316,-2.67765806823329,-33.3814054518618));
#15131=CARTESIAN_POINT('Ctrl Pts',(2.03498792430055,-2.50403513889978,-33.3616524141691));
#15132=CARTESIAN_POINT('Ctrl Pts',(2.15594766665167,-2.40067646646913,-33.3509112477571));
#15133=CARTESIAN_POINT('Ctrl Pts',(2.26878022243767,-2.28883242391741,-33.3405291647262));
#15134=CARTESIAN_POINT('Origin',(0.,0.,-41.3107734492731));
#15135=CARTESIAN_POINT('',(2.26878017977789,-2.28883246620346,-31.8449383693487));
#15136=CARTESIAN_POINT('',(2.2687802230564,-2.28883242330411,-32.0941031001172));
#15137=CARTESIAN_POINT('',(2.26878020078428,-2.2888324453811,-41.3107734492731));
#15138=CARTESIAN_POINT('Ctrl Pts',(2.26878017977789,-2.28883246620346,-31.8449383693487));
#15139=CARTESIAN_POINT('Ctrl Pts',(2.25083588328518,-2.3066195540851,-31.846380501056));
#15140=CARTESIAN_POINT('Ctrl Pts',(2.23268039414462,-2.3241976195804,-31.8478279111245));
#15141=CARTESIAN_POINT('Ctrl Pts',(2.1462447988872,-2.40593611880222,-31.8546706275703));
#15142=CARTESIAN_POINT('Ctrl Pts',(2.07540247335777,-2.46730576859294,-31.8601415705246));
#15143=CARTESIAN_POINT('Ctrl Pts',(1.96325219349776,-2.55620855956848,-31.8686829425726));
#15144=CARTESIAN_POINT('Ctrl Pts',(1.92381287218028,-2.58602107719331,-31.871665215293));
#15145=CARTESIAN_POINT('Ctrl Pts',(1.84817462527405,-2.64050859320595,-31.8773549611355));
#15146=CARTESIAN_POINT('Ctrl Pts',(1.812127704753,-2.66537576456635,-31.8800543163724));
#15147=CARTESIAN_POINT('Ctrl Pts',(1.72782991028612,-2.72102850467852,-31.886344765084));
#15148=CARTESIAN_POINT('Ctrl Pts',(1.67924445321783,-2.7512778370562,-31.889954238958));
#15149=CARTESIAN_POINT('Ctrl Pts',(1.4128275107822,-2.90746285085639,-31.9096745557479));
#15150=CARTESIAN_POINT('Ctrl Pts',(1.18164818863494,-3.00883529266556,-31.9266293063323));
#15151=CARTESIAN_POINT('Ctrl Pts',(0.851284269751612,-3.10970237164751,
-31.9498862792296));
#15152=CARTESIAN_POINT('Ctrl Pts',(0.760322551787671,-3.13318447952589,
-31.9561826750656));
#15153=CARTESIAN_POINT('Ctrl Pts',(0.608364816766492,-3.16540420845404,
-31.9664119974058));
#15154=CARTESIAN_POINT('Ctrl Pts',(0.547911775597553,-3.17642649160067,
-31.9704069821587));
#15155=CARTESIAN_POINT('Ctrl Pts',(0.458194836643132,-3.19014649338539,
-31.9761923790283));
#15156=CARTESIAN_POINT('Ctrl Pts',(0.429152534537554,-3.19418305762291,
-31.9780431230572));
#15157=CARTESIAN_POINT('Ctrl Pts',(0.375078773353542,-3.20094786007096,
-31.9814431589607));
#15158=CARTESIAN_POINT('Ctrl Pts',(0.35006392680792,-3.20378004332276,-31.9829973620236));
#15159=CARTESIAN_POINT('Ctrl Pts',(0.286117003506866,-3.21026220754779,
-31.986927542094));
#15160=CARTESIAN_POINT('Ctrl Pts',(0.247145756334189,-3.21349741867446,
-31.989282537349));
#15161=CARTESIAN_POINT('Ctrl Pts',(0.0108207900656008,-3.22879107716611,
-32.003371646215));
#15162=CARTESIAN_POINT('Ctrl Pts',(-0.18726055140136,-3.22337705591122,
-32.0143908945148));
#15163=CARTESIAN_POINT('Ctrl Pts',(-0.507096719864957,-3.18503339747847,
-32.0325030121935));
#15164=CARTESIAN_POINT('Ctrl Pts',(-0.629614834490448,-3.16309464160002,
-32.0395157929653));
#15165=CARTESIAN_POINT('Ctrl Pts',(-0.836762037811956,-3.11348758835781,
-32.0518072842348));
#15166=CARTESIAN_POINT('Ctrl Pts',(-0.922076070187199,-3.08929595876016,
-32.0569990088072));
#15167=CARTESIAN_POINT('Ctrl Pts',(-1.05272490635079,-3.04635487102285,
-32.0652205457101));
#15168=CARTESIAN_POINT('Ctrl Pts',(-1.09881450676877,-3.03003531753112,
-32.0681744142687));
#15169=CARTESIAN_POINT('Ctrl Pts',(-1.18601302635277,-2.99690864860922,
-32.0738752365067));
#15170=CARTESIAN_POINT('Ctrl Pts',(-1.22718085794768,-2.9802877691009,-32.0766156151959));
#15171=CARTESIAN_POINT('Ctrl Pts',(-1.323948884494,-2.93887423123703,-32.0831797393906));
#15172=CARTESIAN_POINT('Ctrl Pts',(-1.37921417656479,-2.91334685140059,
-32.0870268690308));
#15173=CARTESIAN_POINT('Ctrl Pts',(-1.6626232612589,-2.7725667718116,-32.1072857019854));
#15174=CARTESIAN_POINT('Ctrl Pts',(-1.87715825308495,-2.63204874213256,
-32.1245463100748));
#15175=CARTESIAN_POINT('Ctrl Pts',(-2.13834646174866,-2.4126578648444,-32.1474542580902));
#15176=CARTESIAN_POINT('Ctrl Pts',(-2.20166970063346,-2.35501496362171,
-32.1531719569035));
#15177=CARTESIAN_POINT('Ctrl Pts',(-2.30389382249911,-2.25422922051474,
-32.1625973402715));
#15178=CARTESIAN_POINT('Ctrl Pts',(-2.3440599041077,-2.21243308489319,-32.1663559011371));
#15179=CARTESIAN_POINT('Ctrl Pts',(-2.40253355258328,-2.14820510720482,
-32.1718835959574));
#15180=CARTESIAN_POINT('Ctrl Pts',(-2.42170034524762,-2.12657476499325,
-32.1737050229972));
#15181=CARTESIAN_POINT('Ctrl Pts',(-2.4572556922702,-2.08534516621055,-32.1770973021609));
#15182=CARTESIAN_POINT('Ctrl Pts',(-2.47370644362626,-2.06580407155842,
-32.1786719965604));
#15183=CARTESIAN_POINT('Ctrl Pts',(-2.51600693232524,-2.01432732049326,
-32.1827399623243));
#15184=CARTESIAN_POINT('Ctrl Pts',(-2.54148230592145,-1.98208815951638,
-32.1852091812825));
#15185=CARTESIAN_POINT('Ctrl Pts',(-2.69704990466933,-1.77728412314121,
-32.2004726696924));
#15186=CARTESIAN_POINT('Ctrl Pts',(-2.81013855576133,-1.59246938591455,
-32.2124346304722));
#15187=CARTESIAN_POINT('Ctrl Pts',(-2.95219312378926,-1.29733639368063,
-32.230887026916));
#15188=CARTESIAN_POINT('Ctrl Pts',(-2.99526577543067,-1.19453206597594,
-32.2372009879123));
#15189=CARTESIAN_POINT('Ctrl Pts',(-3.06091380635784,-1.01181742644336,
-32.2484432786366));
#15190=CARTESIAN_POINT('Ctrl Pts',(-3.08588683134635,-0.932881949061886,
-32.2533057073726));
#15191=CARTESIAN_POINT('Ctrl Pts',(-3.1204625871208,-0.806921118863847,
-32.2611283657312));
#15192=CARTESIAN_POINT('Ctrl Pts',(-3.13210186047686,-0.760490646535977,
-32.2640249262468));
#15193=CARTESIAN_POINT('Ctrl Pts',(-3.15259132338029,-0.670282626630437,
-32.2696863776339));
#15194=CARTESIAN_POINT('Ctrl Pts',(-3.16157401945455,-0.626546297592554,
-32.2724464079597));
#15195=CARTESIAN_POINT('Ctrl Pts',(-3.1792506354493,-0.530382830994488,
-32.2785531588805));
#15196=CARTESIAN_POINT('Ctrl Pts',(-3.18756208361038,-0.477899567372165,
-32.2819107512426));
#15197=CARTESIAN_POINT('Ctrl Pts',(-3.22975530768901,-0.16092515098102,
-32.3023473661338));
#15198=CARTESIAN_POINT('Ctrl Pts',(-3.23199421620793,0.106698558096767,
-32.320385288323));
#15199=CARTESIAN_POINT('Ctrl Pts',(-3.19173000777098,0.453679046004111,
-32.3438423296109));
#15200=CARTESIAN_POINT('Ctrl Pts',(-3.17902872457724,0.535483718605843,
-32.3493667979328));
#15201=CARTESIAN_POINT('Ctrl Pts',(-3.15234404317121,0.672352681006745,
-32.358518118322));
#15202=CARTESIAN_POINT('Ctrl Pts',(-3.14002920181656,0.727700850441106,
-32.3621928105448));
#15203=CARTESIAN_POINT('Ctrl Pts',(-3.11930831632351,0.810464340586884,
-32.3676210694632));
#15204=CARTESIAN_POINT('Ctrl Pts',(-3.11198693902731,0.838137367822374,
-32.3694246973641));
#15205=CARTESIAN_POINT('Ctrl Pts',(-3.0974336889949,0.890322975649689,-32.3727996731793));
#15206=CARTESIAN_POINT('Ctrl Pts',(-3.09027734962206,0.914853209685398,
-32.374374525629));
#15207=CARTESIAN_POINT('Ctrl Pts',(-3.07076554150476,0.978892197073889,
-32.3784609029816));
#15208=CARTESIAN_POINT('Ctrl Pts',(-3.05793885156614,1.01825403401639,-32.3809477652685));
#15209=CARTESIAN_POINT('Ctrl Pts',(-2.97412251692548,1.25957853082372,-32.3961021176234));
#15210=CARTESIAN_POINT('Ctrl Pts',(-2.88390729941012,1.4543181869831,-32.4079553553971));
#15211=CARTESIAN_POINT('Ctrl Pts',(-2.71795552466129,1.73534922344312,-32.4263353282678));
#15212=CARTESIAN_POINT('Ctrl Pts',(-2.65586674929463,1.82895842259242,-32.4326949003001));
#15213=CARTESIAN_POINT('Ctrl Pts',(-2.53950015327866,1.98594378806094,-32.4440059698837));
#15214=CARTESIAN_POINT('Ctrl Pts',(-2.48741230417156,2.05080769402615,-32.4488901444259));
#15215=CARTESIAN_POINT('Ctrl Pts',(-2.40146485775406,2.14973910505034,-32.4567369407344));
#15216=CARTESIAN_POINT('Ctrl Pts',(-2.36925167340508,2.18519057020091,-32.4596349736365));
#15217=CARTESIAN_POINT('Ctrl Pts',(-2.30556673476992,2.25221342335293,-32.4652922884253));
#15218=CARTESIAN_POINT('Ctrl Pts',(-2.27420637256636,2.28387572801475,-32.4680465549153));
#15219=CARTESIAN_POINT('Ctrl Pts',(-2.19703467369579,2.35862461684478,-32.4747555442305));
#15220=CARTESIAN_POINT('Ctrl Pts',(-2.15060051292473,2.40103894595991,-32.4787369330605));
#15221=CARTESIAN_POINT('Ctrl Pts',(-1.91778021712075,2.60152956111959,-32.4984483604495));
#15222=CARTESIAN_POINT('Ctrl Pts',(-1.71508782504844,2.73939352585008,-32.5149364938315));
#15223=CARTESIAN_POINT('Ctrl Pts',(-1.41888633657627,2.89500083990007,-32.5374379689575));
#15224=CARTESIAN_POINT('Ctrl Pts',(-1.33722970849517,2.9336132194913,-32.5434815765863));
#15225=CARTESIAN_POINT('Ctrl Pts',(-1.19882303832718,2.99207886570611,-32.553362667385));
#15226=CARTESIAN_POINT('Ctrl Pts',(-1.14294581035873,3.01386602881807,-32.5572571042036));
#15227=CARTESIAN_POINT('Ctrl Pts',(-1.05902494929008,3.04391766645125,-32.5629351043087));
#15228=CARTESIAN_POINT('Ctrl Pts',(-1.03142672873532,3.05337970942992,-32.5647753963254));
#15229=CARTESIAN_POINT('Ctrl Pts',(-0.979633077398192,3.07035473088118,
-32.5681740253747));
#15230=CARTESIAN_POINT('Ctrl Pts',(-0.95547140880725,3.07795931697447,-32.5697368457888));
#15231=CARTESIAN_POINT('Ctrl Pts',(-0.892990635504107,3.09681773332658,
-32.5737249626882));
#15232=CARTESIAN_POINT('Ctrl Pts',(-0.854546221334146,3.10764596204018,
-32.5761279967936));
#15233=CARTESIAN_POINT('Ctrl Pts',(-0.632208441644363,3.16583115169922,
-32.5897863116035));
#15234=CARTESIAN_POINT('Ctrl Pts',(-0.444598695442307,3.19758061653721,
-32.6003916737218));
#15235=CARTESIAN_POINT('Ctrl Pts',(-0.0649455071326363,3.22774707530151,
-32.6218006860141));
#15236=CARTESIAN_POINT('Ctrl Pts',(0.126326062762748,3.22592644778593,-32.6325712379312));
#15237=CARTESIAN_POINT('Ctrl Pts',(0.373914219011914,3.20150856486668,-32.6472656260573));
#15238=CARTESIAN_POINT('Ctrl Pts',(0.431359353452693,3.19427572950281,-32.6507259395644));
#15239=CARTESIAN_POINT('Ctrl Pts',(0.532062040695091,3.17883045479747,-32.65689877275));
#15240=CARTESIAN_POINT('Ctrl Pts',(0.575405130293294,3.1712713099674,-32.6595907303629));
#15241=CARTESIAN_POINT('Ctrl Pts',(0.667839695784798,3.15319317610403,-32.6654132797304));
#15242=CARTESIAN_POINT('Ctrl Pts',(0.716866930620908,3.14240965325868,-32.6685514190392));
#15243=CARTESIAN_POINT('Ctrl Pts',(0.860223985671916,3.10734894106575,-32.6778817680555));
#15244=CARTESIAN_POINT('Ctrl Pts',(0.953721948456661,3.07993737187872,-32.6841675482006));
#15245=CARTESIAN_POINT('Ctrl Pts',(1.25753677142511,2.97570407620439,-32.7052479952225));
#15246=CARTESIAN_POINT('Ctrl Pts',(1.46109355801271,2.88121572739542,-32.7204858707239));
#15247=CARTESIAN_POINT('Ctrl Pts',(1.70991249643382,2.73252314307851,-32.7398416925248));
#15248=CARTESIAN_POINT('Ctrl Pts',(1.76557861967916,2.69689014960709,-32.7442192928158));
#15249=CARTESIAN_POINT('Ctrl Pts',(1.86030349849153,2.63206389133094,-32.7517068566758));
#15250=CARTESIAN_POINT('Ctrl Pts',(1.89986839864351,2.6036493726888,-32.7548464265614));
#15251=CARTESIAN_POINT('Ctrl Pts',(1.96047663790549,2.55800447872138,-32.759656904073));
#15252=CARTESIAN_POINT('Ctrl Pts',(1.98197043911462,2.54138719175909,-32.7613630679379));
#15253=CARTESIAN_POINT('Ctrl Pts',(2.02171898741522,2.5098457412055,-32.7645146925915));
#15254=CARTESIAN_POINT('Ctrl Pts',(2.04002481606516,2.49498940431175,-32.7659646274535));
#15255=CARTESIAN_POINT('Ctrl Pts',(2.09144683894697,2.45231281432277,-32.7700385020309));
#15256=CARTESIAN_POINT('Ctrl Pts',(2.1241695562899,2.42402395033417,-32.7726320685745));
#15257=CARTESIAN_POINT('Ctrl Pts',(2.3093308273636,2.25732164070832,-32.7873801495241));
#15258=CARTESIAN_POINT('Ctrl Pts',(2.44880886121207,2.10519891532581,-32.7988028289234));
#15259=CARTESIAN_POINT('Ctrl Pts',(2.64198066892902,1.84911926120305,-32.8168601661398));
#15260=CARTESIAN_POINT('Ctrl Pts',(2.70618217865005,1.75381863327001,-32.8233591362569));
#15261=CARTESIAN_POINT('Ctrl Pts',(2.80848998372138,1.58291464189368,-32.8348810773274));
#15262=CARTESIAN_POINT('Ctrl Pts',(2.84895971447847,1.50886104377346,-32.8398327684402));
#15263=CARTESIAN_POINT('Ctrl Pts',(2.9078768313499,1.39021055643107,-32.8477620609976));
#15264=CARTESIAN_POINT('Ctrl Pts',(2.92830902276181,1.34663987670954,-32.8506726733008));
#15265=CARTESIAN_POINT('Ctrl Pts',(2.96575238062977,1.26190825397263,-32.8563396253359));
#15266=CARTESIAN_POINT('Ctrl Pts',(2.98290094548011,1.22081991648424,-32.8590905975815));
#15267=CARTESIAN_POINT('Ctrl Pts',(3.02202884611609,1.12131763936864,-32.865765279464));
#15268=CARTESIAN_POINT('Ctrl Pts',(3.04317256965212,1.06259657036668,-32.8697148678552));
#15269=CARTESIAN_POINT('Ctrl Pts',(3.10872802721022,0.862487310983578,-32.8832177932101));
#15270=CARTESIAN_POINT('Ctrl Pts',(3.14508697658735,0.718674708985431,-32.8930043191624));
#15271=CARTESIAN_POINT('Ctrl Pts',(3.19518631999257,0.441331320160369,-32.9118889058492));
#15272=CARTESIAN_POINT('Ctrl Pts',(3.21074159277277,0.308426797108418,-32.9209404836845));
#15273=CARTESIAN_POINT('Ctrl Pts',(3.22175127287199,0.105906404441358,-32.9345021426273));
#15274=CARTESIAN_POINT('Ctrl Pts',(3.22328197619651,0.0367652693626423,
-32.9390900708907));
#15275=CARTESIAN_POINT('Ctrl Pts',(3.22208264448847,-0.0826164956901453,
-32.9468880662188));
#15276=CARTESIAN_POINT('Ctrl Pts',(3.22040299919485,-0.132842677331466,
-32.9501308794266));
#15277=CARTESIAN_POINT('Ctrl Pts',(3.21599056982555,-0.210418022095615,
-32.9550610040053));
#15278=CARTESIAN_POINT('Ctrl Pts',(3.21408157120335,-0.237804258152322,
-32.9567862952362));
#15279=CARTESIAN_POINT('Ctrl Pts',(3.20989823803415,-0.288475287034926,
-32.959946299043));
#15280=CARTESIAN_POINT('Ctrl Pts',(3.20771989716076,-0.31176562337916,-32.9613859789023));
#15281=CARTESIAN_POINT('Ctrl Pts',(3.20090857459537,-0.376930539533431,
-32.9653833164193));
#15282=CARTESIAN_POINT('Ctrl Pts',(3.19570764009236,-0.418742621981689,
-32.9679124801845));
#15283=CARTESIAN_POINT('Ctrl Pts',(3.15978957037525,-0.667562742506565,
-32.9828129972776));
#15284=CARTESIAN_POINT('Ctrl Pts',(3.1097853410238,-0.871300080003428,-32.9944154238782));
#15285=CARTESIAN_POINT('Ctrl Pts',(3.00251751658217,-1.17645011977741,-33.012625793801));
#15286=CARTESIAN_POINT('Ctrl Pts',(2.95897130873465,-1.28204251690308,-33.0190875279521));
#15287=CARTESIAN_POINT('Ctrl Pts',(2.87379517307445,-1.46098694633041,-33.030553400946));
#15288=CARTESIAN_POINT('Ctrl Pts',(2.83472010025197,-1.53542888959496,-33.0354873333003));
#15289=CARTESIAN_POINT('Ctrl Pts',(2.76879687369862,-1.64990654963131,-33.0433951230423));
#15290=CARTESIAN_POINT('Ctrl Pts',(2.74388342933559,-1.69101481674904,-33.0463026344805));
#15291=CARTESIAN_POINT('Ctrl Pts',(2.694132227438,-1.76911067071832,-33.0519675656619));
#15292=CARTESIAN_POINT('Ctrl Pts',(2.66942841901444,-1.80617071007457,-33.0547197124503));
#15293=CARTESIAN_POINT('Ctrl Pts',(2.60820717319357,-1.89401266655825,-33.0614044034138));
#15294=CARTESIAN_POINT('Ctrl Pts',(2.57096504606206,-1.94426503617086,-33.0653630417495));
#15295=CARTESIAN_POINT('Ctrl Pts',(2.45056934212156,-2.09720798546166,-33.0778461096972));
#15296=CARTESIAN_POINT('Ctrl Pts',(2.36256546156562,-2.19586883031866,-33.0865427928208));
#15297=CARTESIAN_POINT('Ctrl Pts',(2.26878017716708,-2.2888324687914,-33.0953665650246));
#15298=CARTESIAN_POINT('Ctrl Pts',(2.26878022243768,-2.28883242391741,-33.3405291647262));
#15299=CARTESIAN_POINT('Ctrl Pts',(2.2815974322282,-2.27612750424933,-33.3393498124077));
#15300=CARTESIAN_POINT('Ctrl Pts',(2.29430977757391,-2.26331308373006,-33.3381752501945));
#15301=CARTESIAN_POINT('Ctrl Pts',(2.33543620901607,-2.22115363659044,-33.334361238633));
#15302=CARTESIAN_POINT('Ctrl Pts',(2.36339974731244,-2.19137576576757,-33.3317455726527));
#15303=CARTESIAN_POINT('Ctrl Pts',(2.40787166087554,-2.1421765670001,-33.3275600333921));
#15304=CARTESIAN_POINT('Ctrl Pts',(2.424728572414,-2.12307745939442,-33.3259673477335));
#15305=CARTESIAN_POINT('Ctrl Pts',(2.46018622729106,-2.08193014870757,-33.3226069194139));
#15306=CARTESIAN_POINT('Ctrl Pts',(2.47872055074316,-2.05982863014307,-33.3208434672996));
#15307=CARTESIAN_POINT('Ctrl Pts',(2.5335875716952,-1.99258844351747,-33.31559178847));
#15308=CARTESIAN_POINT('Ctrl Pts',(2.56900379044949,-1.9467139146164,-33.3121590930041));
#15309=CARTESIAN_POINT('Ctrl Pts',(2.65362054990467,-1.83077586405287,-33.30378054767));
#15310=CARTESIAN_POINT('Ctrl Pts',(2.70130415338509,-1.75965897275495,-33.2988968671888));
#15311=CARTESIAN_POINT('Ctrl Pts',(2.88056244141489,-1.46781433037686,-33.2795193884745));
#15312=CARTESIAN_POINT('Ctrl Pts',(2.98835648675837,-1.23362830000713,-33.2653442274646));
#15313=CARTESIAN_POINT('Ctrl Pts',(3.08586548324229,-0.931261988041518,
-33.2466361085819));
#15314=CARTESIAN_POINT('Ctrl Pts',(3.10288507312785,-0.87287925949752,-33.2430112044922));
#15315=CARTESIAN_POINT('Ctrl Pts',(3.12943437333506,-0.771181718808912,
-33.2366553495684));
#15316=CARTESIAN_POINT('Ctrl Pts',(3.13974057372274,-0.728086241477337,
-33.2339493876052));
#15317=CARTESIAN_POINT('Ctrl Pts',(3.15951093839578,-0.637168421462377,
-33.2282079333869));
#15318=CARTESIAN_POINT('Ctrl Pts',(3.16878501068295,-0.589316655256495,
-33.2251672953158));
#15319=CARTESIAN_POINT('Ctrl Pts',(3.19177271721751,-0.454392146050003,
-33.2165346005326));
#15320=CARTESIAN_POINT('Ctrl Pts',(3.20300388944414,-0.366945685563639,
-33.2108698443246));
#15321=CARTESIAN_POINT('Ctrl Pts',(3.22131818113831,-0.156307985165885,
-33.1970605566852));
#15322=CARTESIAN_POINT('Ctrl Pts',(3.22493916864179,-0.0329582027652135,
-33.1888375032897));
#15323=CARTESIAN_POINT('Ctrl Pts',(3.2158892792051,0.289946190392386,-33.1671241262386));
#15324=CARTESIAN_POINT('Ctrl Pts',(3.19174408638474,0.488662767621672,-33.1535562716225));
#15325=CARTESIAN_POINT('Ctrl Pts',(3.14110992853273,0.721841778671662,-33.1381380285115));
#15326=CARTESIAN_POINT('Ctrl Pts',(3.13217883163252,0.759659929697509,-33.1356547407048));
#15327=CARTESIAN_POINT('Ctrl Pts',(3.11627577706345,0.8219423327106,-33.131603796716));
#15328=CARTESIAN_POINT('Ctrl Pts',(3.10969447453718,0.846501246732696,-33.1300167238944));
#15329=CARTESIAN_POINT('Ctrl Pts',(3.09476944567145,0.899670800413077,-33.1266055425404));
#15330=CARTESIAN_POINT('Ctrl Pts',(3.08631843840116,0.928247874742262,-33.124787073679));
#15331=CARTESIAN_POINT('Ctrl Pts',(3.0585616381,1.0175343225671,-33.1191407200418));
#15332=CARTESIAN_POINT('Ctrl Pts',(3.0378506618822,1.07779396780705,-33.1153814975561));
#15333=CARTESIAN_POINT('Ctrl Pts',(2.98027419515235,1.23043464517424,-33.1059000114187));
#15334=CARTESIAN_POINT('Ctrl Pts',(2.94089431022154,1.32179666326859,-33.1002632209355));
#15335=CARTESIAN_POINT('Ctrl Pts',(2.79369608742939,1.62401196210732,-33.0813185043216));
#15336=CARTESIAN_POINT('Ctrl Pts',(2.66691941525258,1.82474236356701,-33.0681649119777));
#15337=CARTESIAN_POINT('Ctrl Pts',(2.48200555414001,2.05653692367404,-33.0506870742025));
#15338=CARTESIAN_POINT('Ctrl Pts',(2.44340934727261,2.10224779426727,-33.047117928724));
#15339=CARTESIAN_POINT('Ctrl Pts',(2.37412946475749,2.17981177645596,-33.0408250318442));
#15340=CARTESIAN_POINT('Ctrl Pts',(2.3440201885715,2.21215712792206,-33.0381247651418));
#15341=CARTESIAN_POINT('Ctrl Pts',(2.27901920673361,2.27916805398083,-33.0323605564128));
#15342=CARTESIAN_POINT('Ctrl Pts',(2.24398012566538,2.31367420883668,-33.029290722216));
#15343=CARTESIAN_POINT('Ctrl Pts',(2.14199860597922,2.40960829487838,-33.020453173));
#15344=CARTESIAN_POINT('Ctrl Pts',(2.07323366333846,2.46902205143278,-33.0146068720087));
#15345=CARTESIAN_POINT('Ctrl Pts',(1.90039199017234,2.60604277202085,-33.0001794937773));
#15346=CARTESIAN_POINT('Ctrl Pts',(1.7939612724467,2.68041918950734,-32.9915090151857));
#15347=CARTESIAN_POINT('Ctrl Pts',(1.52481879398387,2.84527768743866,-32.9702734009079));
#15348=CARTESIAN_POINT('Ctrl Pts',(1.358177791081,2.92848748170027,-32.9576759668926));
#15349=CARTESIAN_POINT('Ctrl Pts',(1.14778115879816,3.01170091910822,-32.943032277101));
#15350=CARTESIAN_POINT('Ctrl Pts',(1.11000142506506,3.02582900842403,-32.9404508320781));
#15351=CARTESIAN_POINT('Ctrl Pts',(1.04801880832871,3.04769074400936,-32.9363043321251));
#15352=CARTESIAN_POINT('Ctrl Pts',(1.02397285787188,3.05585373487842,-32.9347172674222));
#15353=CARTESIAN_POINT('Ctrl Pts',(0.972222598731633,3.07274212763279,-32.9313506132433));
#15354=CARTESIAN_POINT('Ctrl Pts',(0.944492511835474,3.08137874970391,-32.9295756795287));
#15355=CARTESIAN_POINT('Ctrl Pts',(0.859989506013474,3.10644948513728,-32.9242441493829));
#15356=CARTESIAN_POINT('Ctrl Pts',(0.802875295836612,3.12169865785259,-32.9207456223695));
#15357=CARTESIAN_POINT('Ctrl Pts',(0.65950989410396,3.15578087598898,-32.912151462353));
#15358=CARTESIAN_POINT('Ctrl Pts',(0.572842375995145,3.17265811121929,-32.9071222517133));
#15359=CARTESIAN_POINT('Ctrl Pts',(0.238846222655787,3.22356409536986,-32.8880248769923));
#15360=CARTESIAN_POINT('Ctrl Pts',(-0.0114100151469539,3.23237942279218,
-32.8742312969334));
#15361=CARTESIAN_POINT('Ctrl Pts',(-0.321982003329754,3.20722473081007,
-32.855904270197));
#15362=CARTESIAN_POINT('Ctrl Pts',(-0.38362967329787,3.20043597470433,-32.8522111359217));
#15363=CARTESIAN_POINT('Ctrl Pts',(-0.489082500146419,3.18573277076142,
-32.8457773211945));
#15364=CARTESIAN_POINT('Ctrl Pts',(-0.532991024301267,3.17868136950936,
-32.8430634853532));
#15365=CARTESIAN_POINT('Ctrl Pts',(-0.624224832187557,3.16208642000774,
-32.837345072925));
#15366=CARTESIAN_POINT('Ctrl Pts',(-0.671509481383014,3.15238350993329,
-32.834336193556));
#15367=CARTESIAN_POINT('Ctrl Pts',(-0.801650372699304,3.12261749750859,
-32.8259229835529));
#15368=CARTESIAN_POINT('Ctrl Pts',(-0.883951024262481,3.10032448249165,
-32.8204520388855));
#15369=CARTESIAN_POINT('Ctrl Pts',(-1.07665938532853,3.03982787306527,-32.8072821242616));
#15370=CARTESIAN_POINT('Ctrl Pts',(-1.18606212424275,2.99883342109459,-32.7995150399525));
#15371=CARTESIAN_POINT('Ctrl Pts',(-1.4868604540302,2.86708196989205,-32.7774708454677));
#15372=CARTESIAN_POINT('Ctrl Pts',(-1.67189970196541,2.76327216693552,-32.7630597475327));
#15373=CARTESIAN_POINT('Ctrl Pts',(-1.87708164520897,2.61995660934746,-32.7468923892728));
#15374=CARTESIAN_POINT('Ctrl Pts',(-1.90833490544678,2.59728056373657,-32.7444254118261));
#15375=CARTESIAN_POINT('Ctrl Pts',(-1.95945363087026,2.55876995148225,-32.7403928379803));
#15376=CARTESIAN_POINT('Ctrl Pts',(-1.97955219478087,2.54325293108103,-32.738808203014));
#15377=CARTESIAN_POINT('Ctrl Pts',(-2.02292719340222,2.50893960604838,-32.7353926002089));
#15378=CARTESIAN_POINT('Ctrl Pts',(-2.04612879794041,2.49005410976413,-32.7335674784356));
#15379=CARTESIAN_POINT('Ctrl Pts',(-2.11846848759079,2.42947751712734,-32.7278710792597));
#15380=CARTESIAN_POINT('Ctrl Pts',(-2.16662347248104,2.3866322694978,-32.7240702372045));
#15381=CARTESIAN_POINT('Ctrl Pts',(-2.28710011035673,2.2727856743607,-32.7144416410786));
#15382=CARTESIAN_POINT('Ctrl Pts',(-2.3574176992672,2.19976488968956,-32.7087027598979));
#15383=CARTESIAN_POINT('Ctrl Pts',(-2.57733014835126,1.94871930176628,-32.6899013367315));
#15384=CARTESIAN_POINT('Ctrl Pts',(-2.71110468455041,1.75785100827698,-32.6769742390252));
#15385=CARTESIAN_POINT('Ctrl Pts',(-2.85229916113503,1.50138292843653,-32.6597270239733));
#15386=CARTESIAN_POINT('Ctrl Pts',(-2.87991784346774,1.44769946412563,-32.6561270870826));
#15387=CARTESIAN_POINT('Ctrl Pts',(-2.92514201908039,1.35337348664802,-32.6497996798029));
#15388=CARTESIAN_POINT('Ctrl Pts',(-2.94344780861348,1.31308428135173,-32.6470965288372));
#15389=CARTESIAN_POINT('Ctrl Pts',(-2.98023303065432,1.22748601163033,-32.6413459165926));
#15390=CARTESIAN_POINT('Ctrl Pts',(-2.99852161134579,1.1821076788523,-32.6382929867005));
#15391=CARTESIAN_POINT('Ctrl Pts',(-3.04725003618361,1.05278488299647,-32.6295736237474));
#15392=CARTESIAN_POINT('Ctrl Pts',(-3.07524255259424,0.967971953567275,
-32.6238320127503));
#15393=CARTESIAN_POINT('Ctrl Pts',(-3.13416365658659,0.760927611098515,
-32.6097633118767));
#15394=CARTESIAN_POINT('Ctrl Pts',(-3.16151179436378,0.637833457108885,
-32.6013532233444));
#15395=CARTESIAN_POINT('Ctrl Pts',(-3.212465236872,0.322109630769983,-32.57984681089));
#15396=CARTESIAN_POINT('Ctrl Pts',(-3.22602271593976,0.128349844134028,
-32.5666937389803));
#15397=CARTESIAN_POINT('Ctrl Pts',(-3.22128256542905,-0.104962294955333,
-32.5516036674606));
#15398=CARTESIAN_POINT('Ctrl Pts',(-3.21975372826244,-0.144446178298068,
-32.5490768268331));
#15399=CARTESIAN_POINT('Ctrl Pts',(-3.21605741476315,-0.209118714780682,
-32.5449924904373));
#15400=CARTESIAN_POINT('Ctrl Pts',(-3.21431905868137,-0.234326882862213,
-32.543414254866));
#15401=CARTESIAN_POINT('Ctrl Pts',(-3.20991898652324,-0.288791292684576,
-32.5400367778838));
#15402=CARTESIAN_POINT('Ctrl Pts',(-3.20715349735872,-0.318036002562597,
-32.5382427985214));
#15403=CARTESIAN_POINT('Ctrl Pts',(-3.19740645270749,-0.407972118388398,
-32.5327750166298));
#15404=CARTESIAN_POINT('Ctrl Pts',(-3.18909857162773,-0.468508859145859,
-32.5291637721633));
#15405=CARTESIAN_POINT('Ctrl Pts',(-3.16382118005518,-0.620479850239381,
-32.5201928028806));
#15406=CARTESIAN_POINT('Ctrl Pts',(-3.14460654418237,-0.711485210831207,
-32.5149073068681));
#15407=CARTESIAN_POINT('Ctrl Pts',(-3.05870670186714,-1.04601126980313,
-32.4954124982467));
#15408=CARTESIAN_POINT('Ctrl Pts',(-2.96743453887896,-1.28224413779704,
-32.4814360873824));
#15409=CARTESIAN_POINT('Ctrl Pts',(-2.82286436611143,-1.55589693967944,
-32.463153272247));
#15410=CARTESIAN_POINT('Ctrl Pts',(-2.79485369377115,-1.60566832335914,
-32.4597398967317));
#15411=CARTESIAN_POINT('Ctrl Pts',(-2.74294386451853,-1.69242809094574,
-32.4536151884451));
#15412=CARTESIAN_POINT('Ctrl Pts',(-2.71958079605436,-1.72972075503202,
-32.4509231221459));
#15413=CARTESIAN_POINT('Ctrl Pts',(-2.66803393858905,-1.80837395621602,
-32.4451105685868));
#15414=CARTESIAN_POINT('Ctrl Pts',(-2.63963577296326,-1.84957941516449,
-32.4419827600668));
#15415=CARTESIAN_POINT('Ctrl Pts',(-2.55374237163742,-1.9682007271315,-32.4327257345505));
#15416=CARTESIAN_POINT('Ctrl Pts',(-2.49372243359689,-2.04371224273494,
-32.4265052067696));
#15417=CARTESIAN_POINT('Ctrl Pts',(-2.33585429497226,-2.22500221416585,
-32.410735245973));
#15418=CARTESIAN_POINT('Ctrl Pts',(-2.2341311116399,-2.32712328416571,-32.4010698372943));
#15419=CARTESIAN_POINT('Ctrl Pts',(-2.00651131109712,-2.52691058902443,
-32.3806714397064));
#15420=CARTESIAN_POINT('Ctrl Pts',(-1.87949660575656,-2.62275886816318,
-32.369958240645));
#15421=CARTESIAN_POINT('Ctrl Pts',(-1.71032621107988,-2.73179340987916,
-32.3569046598221));
#15422=CARTESIAN_POINT('Ctrl Pts',(-1.6742796409564,-2.7540332332896,-32.3541888181361));
#15423=CARTESIAN_POINT('Ctrl Pts',(-1.61762499048443,-2.78746406087564,
-32.3500330044091));
#15424=CARTESIAN_POINT('Ctrl Pts',(-1.59731651132404,-2.79915104320127,
-32.3485652643575));
#15425=CARTESIAN_POINT('Ctrl Pts',(-1.55297764875523,-2.82402713061975,
-32.3454110684784));
#15426=CARTESIAN_POINT('Ctrl Pts',(-1.5289027696891,-2.83713328085056,-32.3437297535109));
#15427=CARTESIAN_POINT('Ctrl Pts',(-1.46046516621276,-2.87326590960952,
-32.3390298794213));
#15428=CARTESIAN_POINT('Ctrl Pts',(-1.41572823777866,-2.89557069069907,
-32.3360506831119));
#15429=CARTESIAN_POINT('Ctrl Pts',(-1.14203251646074,-3.02416820933234,
-32.3182744569069));
#15430=CARTESIAN_POINT('Ctrl Pts',(-0.9017390025095,-3.10430711995979,-32.3044831216224));
#15431=CARTESIAN_POINT('Ctrl Pts',(-0.537303710116642,-3.17989890461302,
-32.2833161060094));
#15432=CARTESIAN_POINT('Ctrl Pts',(-0.418816860247447,-3.19766179005776,
-32.2764081120268));
#15433=CARTESIAN_POINT('Ctrl Pts',(-0.245576636569195,-3.21383823689162,
-32.2660884180779));
#15434=CARTESIAN_POINT('Ctrl Pts',(-0.191413404359537,-3.21751837554626,
-32.2628319206372));
#15435=CARTESIAN_POINT('Ctrl Pts',(-0.093457474831853,-3.22169192450732,
-32.2568746313912));
#15436=CARTESIAN_POINT('Ctrl Pts',(-0.0496979836122681,-3.2226639569138,
-32.2541890225231));
#15437=CARTESIAN_POINT('Ctrl Pts',(0.0468487302272742,-3.22284172256959,
-32.2482042174224));
#15438=CARTESIAN_POINT('Ctrl Pts',(0.0996231243880949,-3.2216421735617,
-32.2448934835205));
#15439=CARTESIAN_POINT('Ctrl Pts',(0.268627209632442,-3.21364427555639,
-32.2341573191384));
#15440=CARTESIAN_POINT('Ctrl Pts',(0.384517066310479,-3.20184506847776,
-32.2265879972149));
#15441=CARTESIAN_POINT('Ctrl Pts',(0.710789779902625,-3.15065637098371,
-32.2047329711291));
#15442=CARTESIAN_POINT('Ctrl Pts',(0.918234945117026,-3.09656167630718,
-32.190151127381));
#15443=CARTESIAN_POINT('Ctrl Pts',(1.19447700207898,-2.99430400275913,-32.170571244194));
#15444=CARTESIAN_POINT('Ctrl Pts',(1.2690948516739,-2.96344934072554,-32.1652710526442));
#15445=CARTESIAN_POINT('Ctrl Pts',(1.37194288818179,-2.91632312282324,-32.1580197509992));
#15446=CARTESIAN_POINT('Ctrl Pts',(1.40120130314866,-2.90237884179815,-32.155963304045));
#15447=CARTESIAN_POINT('Ctrl Pts',(1.45262365682647,-2.8769125237363,-32.1523667801924));
#15448=CARTESIAN_POINT('Ctrl Pts',(1.47487137825699,-2.86557073950386,-32.1508172576355));
#15449=CARTESIAN_POINT('Ctrl Pts',(1.52708523768021,-2.83818310935327,-32.1471950767989));
#15450=CARTESIAN_POINT('Ctrl Pts',(1.55693294504448,-2.82192003791012,-32.1451350262465));
#15451=CARTESIAN_POINT('Ctrl Pts',(1.6713397190822,-2.75721542873139,-32.1372584150021));
#15452=CARTESIAN_POINT('Ctrl Pts',(1.75394834572748,-2.70541711894681,-32.1316123486419));
#15453=CARTESIAN_POINT('Ctrl Pts',(1.98935590321743,-2.54248639838375,-32.115275583791));
#15454=CARTESIAN_POINT('Ctrl Pts',(2.13480069364762,-2.42163817331102,-32.1048365903351));
#15455=CARTESIAN_POINT('Ctrl Pts',(2.26878022305635,-2.28883242330415,-32.0941031001172));
#15456=CARTESIAN_POINT('Origin',(0.,0.,-39.));
#15457=CARTESIAN_POINT('',(3.9333499476854,-0.00313792129108339,-38.595836477965));
#15458=CARTESIAN_POINT('',(-1.7510912850176,-3.52776001450859,-38.9999028013849));
#15459=CARTESIAN_POINT('Ctrl Pts',(3.93554779283278,-0.00313967467311022,
-38.595836477965));
#15460=CARTESIAN_POINT('Ctrl Pts',(3.93730083378416,-0.212909402327876,
-38.6064681800308));
#15461=CARTESIAN_POINT('Ctrl Pts',(3.82770051767509,-1.70709904727174,-38.6822941691407));
#15462=CARTESIAN_POINT('Ctrl Pts',(2.00357591915369,-4.09649302512289,-38.8169829436141));
#15463=CARTESIAN_POINT('Ctrl Pts',(-0.708776008939174,-4.0366411418627,
-38.9410400160216));
#15464=CARTESIAN_POINT('Ctrl Pts',(-1.7510912850176,-3.52776001450859,-38.9999028013849));
#15465=CARTESIAN_POINT('',(1.74869447533106,-3.52286199445091,-39.));
#15466=CARTESIAN_POINT('Origin',(0.,0.,-39.));
#15467=CARTESIAN_POINT('',(3.9346390333135,-0.00367440651247183,-38.779163522035));
#15468=CARTESIAN_POINT('Ctrl Pts',(1.74869447533105,-3.52286199445091,-39.));
#15469=CARTESIAN_POINT('Ctrl Pts',(2.9031442039855,-2.94981091674041,-38.9348057129559));
#15470=CARTESIAN_POINT('Ctrl Pts',(3.85357960338317,-1.6179858509449,-38.8611935536343));
#15471=CARTESIAN_POINT('Ctrl Pts',(3.9372815668327,-0.169521116836944,-38.7875813943125));
#15472=CARTESIAN_POINT('Ctrl Pts',(3.93601136498645,-0.00367568807969895,
-38.779163522035));
#15473=CARTESIAN_POINT('',(3.93299998071207,0.000389511058544483,-37.529163521997));
#15474=CARTESIAN_POINT('Ctrl Pts',(3.93299828502308,-0.00367287428139504,
-38.779163522035));
#15475=CARTESIAN_POINT('Ctrl Pts',(3.93310403942478,0.109571372226196,-38.7734110959793));
#15476=CARTESIAN_POINT('Ctrl Pts',(3.9283146543598,0.223023809436804,-38.7676586699237));
#15477=CARTESIAN_POINT('Ctrl Pts',(3.91860284299163,0.336215346017903,-38.761906243868));
#15478=CARTESIAN_POINT('Ctrl Pts',(3.90890215755498,0.449277209437349,-38.7561604078393));
#15479=CARTESIAN_POINT('Ctrl Pts',(3.89429028806077,0.5620783406858,-38.7504145718106));
#15480=CARTESIAN_POINT('Ctrl Pts',(3.87479196582847,0.674148515945203,-38.7446687357818));
#15481=CARTESIAN_POINT('Ctrl Pts',(3.85531062193827,0.786121105076323,-38.7389279029923));
#15482=CARTESIAN_POINT('Ctrl Pts',(3.83095135722373,0.897363581263983,-38.7331870702027));
#15483=CARTESIAN_POINT('Ctrl Pts',(3.80179073465061,1.00741064612441,-38.7274462374132));
#15484=CARTESIAN_POINT('Ctrl Pts',(3.77264376560108,1.11740618498629,-38.7217080925839));
#15485=CARTESIAN_POINT('Ctrl Pts',(3.73870001351969,1.22620700873158,-38.7159699477547));
#15486=CARTESIAN_POINT('Ctrl Pts',(3.70008701768355,1.33335856451655,-38.7102318029254));
#15487=CARTESIAN_POINT('Ctrl Pts',(3.66148195017559,1.44048811908973,-38.7044948362978));
#15488=CARTESIAN_POINT('Ctrl Pts',(3.61820968976194,1.54596867354476,-38.6987578696702));
#15489=CARTESIAN_POINT('Ctrl Pts',(3.57044717408169,1.64936229406763,-38.6930209030426));
#15490=CARTESIAN_POINT('Ctrl Pts',(3.52268190956214,1.75276186512397,-38.6872836062398));
#15491=CARTESIAN_POINT('Ctrl Pts',(3.47042605816341,1.85407387317384,-38.681546309437));
#15492=CARTESIAN_POINT('Ctrl Pts',(3.41390368481467,1.95288264645083,-38.6758090126341));
#15493=CARTESIAN_POINT('Ctrl Pts',(3.35732852695473,2.0517836942112,-38.6700663579458));
#15494=CARTESIAN_POINT('Ctrl Pts',(3.2964791044753,2.14817646423882,-38.6643237032574));
#15495=CARTESIAN_POINT('Ctrl Pts',(3.23162418551736,2.24167217129965,-38.658581048569));
#15496=CARTESIAN_POINT('Ctrl Pts',(3.16673908556028,2.33521138768714,-38.6528357214688));
#15497=CARTESIAN_POINT('Ctrl Pts',(3.09784504016324,2.42585051537552,-38.6470903943685));
#15498=CARTESIAN_POINT('Ctrl Pts',(3.02525145244781,2.51323350476282,-38.6413450672682));
#15499=CARTESIAN_POINT('Ctrl Pts',(2.95254227015903,2.60075563866267,-38.6355905915826));
#15500=CARTESIAN_POINT('Ctrl Pts',(2.87612206962711,2.68501096021976,-38.629836115897));
#15501=CARTESIAN_POINT('Ctrl Pts',(2.79633764742713,2.76567980098595,-38.6240816402113));
#15502=CARTESIAN_POINT('Ctrl Pts',(2.72587064216683,2.83692794028269,-38.6189991860526));
#15503=CARTESIAN_POINT('Ctrl Pts',(2.65277997360696,2.9053788043207,-38.6139167318939));
#15504=CARTESIAN_POINT('Ctrl Pts',(2.57732468195596,2.97083935677791,-38.6088342777352));
#15505=CARTESIAN_POINT('Ctrl Pts',(2.48987138838526,3.04670866675049,-38.6029436722406));
#15506=CARTESIAN_POINT('Ctrl Pts',(2.39892754289888,3.11883256847447,-38.5970530667459));
#15507=CARTESIAN_POINT('Ctrl Pts',(2.30484669155908,3.1868747588208,-38.5911624612512));
#15508=CARTESIAN_POINT('Ctrl Pts',(2.21088382408729,3.25483161957359,-38.5852792429816));
#15509=CARTESIAN_POINT('Ctrl Pts',(2.1137921052492,3.31871671175555,-38.579396024712));
#15510=CARTESIAN_POINT('Ctrl Pts',(2.01395958894456,3.37823264061228,-38.5735128064424));
#15511=CARTESIAN_POINT('Ctrl Pts',(1.91422606988959,3.43768955149085,-38.5676354221681));
#15512=CARTESIAN_POINT('Ctrl Pts',(1.81175751084977,3.49278570946986,-38.5617580378937));
#15513=CARTESIAN_POINT('Ctrl Pts',(1.70697198469082,3.54326623942947,-38.5558806536194));
#15514=CARTESIAN_POINT('Ctrl Pts',(1.60101867459009,3.59430935044794,-38.5499377687437));
#15515=CARTESIAN_POINT('Ctrl Pts',(1.49269678112721,3.64063307271995,-38.543994883868));
#15516=CARTESIAN_POINT('Ctrl Pts',(1.38246565758099,3.68202087251134,-38.5380519989923));
#15517=CARTESIAN_POINT('Ctrl Pts',(1.2735689627828,3.72290764257462,-38.5321810571049));
#15518=CARTESIAN_POINT('Ctrl Pts',(1.16280940652878,3.75897720033455,-38.5263101152174));
#15519=CARTESIAN_POINT('Ctrl Pts',(1.05065053183007,3.79006892549004,-38.5204391733299));
#15520=CARTESIAN_POINT('Ctrl Pts',(0.938507535572435,3.82115624895972,-38.5145690625975));
#15521=CARTESIAN_POINT('Ctrl Pts',(0.824966010151,3.84726703192967,-38.508698951865));
#15522=CARTESIAN_POINT('Ctrl Pts',(0.710504059987592,3.86829070530398,-38.5028288411325));
#15523=CARTESIAN_POINT('Ctrl Pts',(0.5960311126015,3.88931639858113,-38.4969581664142));
#15524=CARTESIAN_POINT('Ctrl Pts',(0.480637968203892,3.90525393657037,-38.4910874916959));
#15525=CARTESIAN_POINT('Ctrl Pts',(0.364811642391675,3.91604410924794,-38.4852168169776));
#15526=CARTESIAN_POINT('Ctrl Pts',(0.246490661258306,3.92706667953889,-38.4792197002797));
#15527=CARTESIAN_POINT('Ctrl Pts',(0.127718069625044,3.93271755714998,-38.4732225835818));
#15528=CARTESIAN_POINT('Ctrl Pts',(0.00901585574032525,3.93298966618847,
-38.4672254668839));
#15529=CARTESIAN_POINT('Ctrl Pts',(-0.107349584636595,3.93325641848447,
-38.4613464095125));
#15530=CARTESIAN_POINT('Ctrl Pts',(-0.223646980528024,3.92835430643586,
-38.4554673521411));
#15531=CARTESIAN_POINT('Ctrl Pts',(-0.339388193689483,3.91832931923597,
-38.4495882947697));
#15532=CARTESIAN_POINT('Ctrl Pts',(-0.458615764137953,3.90800235933144,
-38.4435321484085));
#15533=CARTESIAN_POINT('Ctrl Pts',(-0.577252643695642,3.8922390778494,-38.4374760020474));
#15534=CARTESIAN_POINT('Ctrl Pts',(-0.69477607476468,3.87114649760695,-38.4314198556863));
#15535=CARTESIAN_POINT('Ctrl Pts',(-0.812299505833717,3.85005391736451,
-38.4253637093252));
#15536=CARTESIAN_POINT('Ctrl Pts',(-0.92870904423043,3.8236322024653,-38.419307562964));
#15537=CARTESIAN_POINT('Ctrl Pts',(-1.0434996866262,3.79204396124452,-38.4132514166029));
#15538=CARTESIAN_POINT('Ctrl Pts',(-1.15520854495649,3.76130376945023,-38.4073578595867));
#15539=CARTESIAN_POINT('Ctrl Pts',(-1.26572912502489,3.7255761015192,-38.4014643025705));
#15540=CARTESIAN_POINT('Ctrl Pts',(-1.37458525047183,3.68497006625363,-38.3955707455544));
#15541=CARTESIAN_POINT('Ctrl Pts',(-1.48330825929835,3.6444136867898,-38.3896843955777));
#15542=CARTESIAN_POINT('Ctrl Pts',(-1.59037048124739,3.59899094817998,-38.383798045601));
#15543=CARTESIAN_POINT('Ctrl Pts',(-1.69530914157331,3.54886121375547,-38.3779116956242));
#15544=CARTESIAN_POINT('Ctrl Pts',(-1.80014692174289,3.49877967029729,-38.3720310043429));
#15545=CARTESIAN_POINT('Ctrl Pts',(-1.90286483388534,3.44400030914931,-38.3661503130615));
#15546=CARTESIAN_POINT('Ctrl Pts',(-2.00301898693927,3.38473099934999,-38.3602696217801));
#15547=CARTESIAN_POINT('Ctrl Pts',(-2.10421236949566,3.32484669343263,-38.3543279106838));
#15548=CARTESIAN_POINT('Ctrl Pts',(-2.20278808548508,3.26037887490091,-38.3483861995876));
#15549=CARTESIAN_POINT('Ctrl Pts',(-2.29831241675886,3.19159036139853,-38.3424444884914));
#15550=CARTESIAN_POINT('Ctrl Pts',(-2.3927587841673,3.12357810595437,-38.33656982785));
#15551=CARTESIAN_POINT('Ctrl Pts',(-2.48422194944399,3.05134242750369,-38.3306951672086));
#15552=CARTESIAN_POINT('Ctrl Pts',(-2.57231145605353,2.97518113281456,-38.3248205065672));
#15553=CARTESIAN_POINT('Ctrl Pts',(-2.66039072498379,2.89902868951919,-38.3189465286733));
#15554=CARTESIAN_POINT('Ctrl Pts',(-2.74509680518825,2.81895180536477,-38.3130725507795));
#15555=CARTESIAN_POINT('Ctrl Pts',(-2.82607291940948,2.73528807517241,-38.3071985728856));
#15556=CARTESIAN_POINT('Ctrl Pts',(-2.90705880239056,2.65161425199279,-38.3013238863694));
#15557=CARTESIAN_POINT('Ctrl Pts',(-2.98431353973336,2.56435301685264,-38.2954491998533));
#15558=CARTESIAN_POINT('Ctrl Pts',(-3.05751823924298,2.47387776915039,-38.2895745133371));
#15559=CARTESIAN_POINT('Ctrl Pts',(-3.13218681977183,2.38159327970945,-38.2835823501815));
#15560=CARTESIAN_POINT('Ctrl Pts',(-3.20264136328559,2.2859651996263,-38.277590187026));
#15561=CARTESIAN_POINT('Ctrl Pts',(-3.26858839065875,2.1874228974871,-38.2715980238705));
#15562=CARTESIAN_POINT('Ctrl Pts',(-3.33333834646129,2.09066933690446,-38.2657146305632));
#15563=CARTESIAN_POINT('Ctrl Pts',(-3.39374288383936,1.99110684518476,-38.2598312372559));
#15564=CARTESIAN_POINT('Ctrl Pts',(-3.44957008258935,1.88916787112859,-38.2539478439486));
#15565=CARTESIAN_POINT('Ctrl Pts',(-3.50694544809086,1.78440198592781,-38.2479012958689));
#15566=CARTESIAN_POINT('Ctrl Pts',(-3.55948568566393,1.67712630679095,-38.2418547477893));
#15567=CARTESIAN_POINT('Ctrl Pts',(-3.60699189470479,1.56783241181383,-38.2358081997096));
#15568=CARTESIAN_POINT('Ctrl Pts',(-3.65449810374564,1.45853851683671,-38.2297616516299));
#15569=CARTESIAN_POINT('Ctrl Pts',(-3.69697017722673,1.34722686104502,-38.2237151035502));
#15570=CARTESIAN_POINT('Ctrl Pts',(-3.7342648234265,1.23440480739482,-38.2176685554706));
#15571=CARTESIAN_POINT('Ctrl Pts',(-3.77052159073377,1.12472249738144,-38.2117902777799));
#15572=CARTESIAN_POINT('Ctrl Pts',(-3.80200079442422,1.0132633042238,-38.2059120000893));
#15573=CARTESIAN_POINT('Ctrl Pts',(-3.82852756824506,0.900480793347386,
-38.2000337223986));
#15574=CARTESIAN_POINT('Ctrl Pts',(-3.85502069485874,0.787841338559683,
-38.1941629008588));
#15575=CARTESIAN_POINT('Ctrl Pts',(-3.87657379121321,0.67388230218471,-38.188292079319));
#15576=CARTESIAN_POINT('Ctrl Pts',(-3.89306112942339,0.559074272858875,
-38.1824212577792));
#15577=CARTESIAN_POINT('Ctrl Pts',(-3.90953193684349,0.444381354135343,
-38.1765563225334));
#15578=CARTESIAN_POINT('Ctrl Pts',(-3.92094703126756,0.328841541576567,
-38.1706913872875));
#15579=CARTESIAN_POINT('Ctrl Pts',(-3.92723145224885,0.212936893157096,
-38.1648264520416));
#15580=CARTESIAN_POINT('Ctrl Pts',(-3.93360437720446,0.0953999508386366,
-38.1588789204706));
#15581=CARTESIAN_POINT('Ctrl Pts',(-3.93470090624358,-0.0225117637689814,
-38.1529313888996));
#15582=CARTESIAN_POINT('Ctrl Pts',(-3.93049719147084,-0.140288373858487,
-38.1469838573286));
#15583=CARTESIAN_POINT('Ctrl Pts',(-3.92635644108237,-0.25630089381883,
-38.1411254095047));
#15584=CARTESIAN_POINT('Ctrl Pts',(-3.91707315609044,-0.372181903431668,
-38.1352669616807));
#15585=CARTESIAN_POINT('Ctrl Pts',(-3.90267701153491,-0.487443477376551,
-38.1294085138568));
#15586=CARTESIAN_POINT('Ctrl Pts',(-3.88828289391023,-0.602688822862551,
-38.1235508908834));
#15587=CARTESIAN_POINT('Ctrl Pts',(-3.86877739943271,-0.717314497090862,
-38.1176932679101));
#15588=CARTESIAN_POINT('Ctrl Pts',(-3.84424200732712,-0.830838365208051,
-38.1118356449367));
#15589=CARTESIAN_POINT('Ctrl Pts',(-3.81970416507145,-0.944373570030658,
-38.1059774370102));
#15590=CARTESIAN_POINT('Ctrl Pts',(-3.79013551385952,-1.05680634701712,
-38.1001192290837));
#15591=CARTESIAN_POINT('Ctrl Pts',(-3.75566836719429,-1.16766609767356,
-38.0942610211572));
#15592=CARTESIAN_POINT('Ctrl Pts',(-3.72028101543238,-1.28148558586095,
-38.0882464105889));
#15593=CARTESIAN_POINT('Ctrl Pts',(-3.67973004258524,-1.39364642639785,
-38.0822318000207));
#15594=CARTESIAN_POINT('Ctrl Pts',(-3.63421238298233,-1.50365865653675,
-38.0762171894524));
#15595=CARTESIAN_POINT('Ctrl Pts',(-3.58981364157883,-1.61096655856358,
-38.0703504304496));
#15596=CARTESIAN_POINT('Ctrl Pts',(-3.54068979591582,-1.71622990698234,
-38.0644836714468));
#15597=CARTESIAN_POINT('Ctrl Pts',(-3.48707090017794,-1.81901773964198,
-38.058616912444));
#15598=CARTESIAN_POINT('Ctrl Pts',(-3.43142508352822,-1.92569119517083,
-38.052528376093));
#15599=CARTESIAN_POINT('Ctrl Pts',(-3.37093791991247,-2.02969785558404,
-38.046439839742));
#15600=CARTESIAN_POINT('Ctrl Pts',(-3.30591594764488,-2.1305888263828,-38.0403513033911));
#15601=CARTESIAN_POINT('Ctrl Pts',(-3.24089397537729,-2.23147979718156,
-38.0342627670401));
#15602=CARTESIAN_POINT('Ctrl Pts',(-3.17133753228712,-2.32925471819556,
-38.0281742306891));
#15603=CARTESIAN_POINT('Ctrl Pts',(-3.09759881119903,-2.4235037868463,-38.0220856943382));
#15604=CARTESIAN_POINT('Ctrl Pts',(-3.02631412947532,-2.5146162276696,-38.0161997856929));
#15605=CARTESIAN_POINT('Ctrl Pts',(-2.95089313000904,-2.60272526257842,
-38.0103138770477));
#15606=CARTESIAN_POINT('Ctrl Pts',(-2.87161794774054,-2.68743360145221,
-38.0044279684024));
#15607=CARTESIAN_POINT('Ctrl Pts',(-2.79244200045035,-2.77203590423842,
-37.9985494276118));
#15608=CARTESIAN_POINT('Ctrl Pts',(-2.70942174467608,-2.85324568012192,
-37.9926708868211));
#15609=CARTESIAN_POINT('Ctrl Pts',(-2.62288064297686,-2.9306972093168,-37.9867923460305));
#15610=CARTESIAN_POINT('Ctrl Pts',(-2.53642504872363,-3.00807221207143,
-37.9809196135667));
#15611=CARTESIAN_POINT('Ctrl Pts',(-2.44645583372397,-3.08169608266493,
-37.975046881103));
#15612=CARTESIAN_POINT('Ctrl Pts',(-2.35333406803029,-3.15123908395539,
-37.9691741486393));
#15613=CARTESIAN_POINT('Ctrl Pts',(-2.25907212034071,-3.22163356907911,
-37.9632295104962));
#15614=CARTESIAN_POINT('Ctrl Pts',(-2.16158019445166,-3.28784626766858,
-37.9572848723531));
#15615=CARTESIAN_POINT('Ctrl Pts',(-2.06126854352396,-3.34957624058307,
-37.9513402342101));
#15616=CARTESIAN_POINT('Ctrl Pts',(-1.96227733703284,-3.4104936359101,-37.9454738478383));
#15617=CARTESIAN_POINT('Ctrl Pts',(-1.86054055956049,-3.46704540009716,
-37.9396074614665));
#15618=CARTESIAN_POINT('Ctrl Pts',(-1.75648197291948,-3.51898566050061,
-37.9337410750947));
#15619=CARTESIAN_POINT('Ctrl Pts',(-1.65243732970433,-3.57091896112118,
-37.9278754747947));
#15620=CARTESIAN_POINT('Ctrl Pts',(-1.54607186377699,-3.61824180339004,
-37.9220098744947));
#15621=CARTESIAN_POINT('Ctrl Pts',(-1.43783318258035,-3.66075466797092,
-37.9161442741948));
#15622=CARTESIAN_POINT('Ctrl Pts',(-1.32958315663315,-3.70327198842505,
-37.9102780591075));
#15623=CARTESIAN_POINT('Ctrl Pts',(-1.21945990771322,-3.74097817870569,
-37.9044118440201));
#15624=CARTESIAN_POINT('Ctrl Pts',(-1.10792958207428,-3.77372243827825,
-37.8985456289328));
#15625=CARTESIAN_POINT('Ctrl Pts',(-0.993787891794018,-3.80723337006452,
-37.8925420626222));
#15626=CARTESIAN_POINT('Ctrl Pts',(-0.878172845458401,-3.83554698500218,
-37.8865384963116));
#15627=CARTESIAN_POINT('Ctrl Pts',(-0.761597616398928,-3.85855647499106,
-37.8805349300011));
#15628=CARTESIAN_POINT('Ctrl Pts',(-0.647523367456019,-3.88107232428614,
-37.8746601629225));
#15629=CARTESIAN_POINT('Ctrl Pts',(-0.532530140825998,-3.89850934457288,
-37.8687853958439));
#15630=CARTESIAN_POINT('Ctrl Pts',(-0.417105225738954,-3.91081989238334,
-37.8629106287653));
#15631=CARTESIAN_POINT('Ctrl Pts',(-0.297884422181058,-3.92353528750487,
-37.8568426628387));
#15632=CARTESIAN_POINT('Ctrl Pts',(-0.178203529785833,-3.93078119112377,
-37.8507746969121));
#15633=CARTESIAN_POINT('Ctrl Pts',(-0.0585996244716005,-3.93256342402914,
-37.8447067309855));
#15634=CARTESIAN_POINT('Ctrl Pts',(0.0610042808426331,-3.93434565693451,
-37.8386387650589));
#15635=CARTESIAN_POINT('Ctrl Pts',(0.180530724763209,-3.93066429775285,
-37.8325707991324));
#15636=CARTESIAN_POINT('Ctrl Pts',(0.299449635869794,-3.92158372543255,
-37.8265028332058));
#15637=CARTESIAN_POINT('Ctrl Pts',(0.41479306394575,-3.91277617471948,-37.820617310164));
#15638=CARTESIAN_POINT('Ctrl Pts',(0.529930234432639,-3.89886158014946,
-37.8147317871223));
#15639=CARTESIAN_POINT('Ctrl Pts',(0.644374131683919,-3.87985450479997,
-37.8088462640805));
#15640=CARTESIAN_POINT('Ctrl Pts',(0.758675010952778,-3.86087118216803,
-37.8029680960454));
#15641=CARTESIAN_POINT('Ctrl Pts',(0.872283937964804,-3.83680810304319,
-37.7970899280104));
#15642=CARTESIAN_POINT('Ctrl Pts',(0.984717262339541,-3.80773172810934,
-37.7912117599753));
#15643=CARTESIAN_POINT('Ctrl Pts',(1.09703974336824,-3.77868401836622,-37.785339386982));
#15644=CARTESIAN_POINT('Ctrl Pts',(1.20818853149974,-3.74463294734043,-37.7794670139888));
#15645=CARTESIAN_POINT('Ctrl Pts',(1.31768907691635,-3.70569622292159,-37.7735946409955));
#15646=CARTESIAN_POINT('Ctrl Pts',(1.42853973645088,-3.66627941850731,-37.7676498631237));
#15647=CARTESIAN_POINT('Ctrl Pts',(1.53770081122438,-3.62185573636504,-37.761705085252));
#15648=CARTESIAN_POINT('Ctrl Pts',(1.64469434049997,-3.57259982734246,-37.7557603073802));
#15649=CARTESIAN_POINT('Ctrl Pts',(1.75027115444445,-3.52399612226092,-37.7498942450907));
#15650=CARTESIAN_POINT('Ctrl Pts',(1.85373709783592,-3.47068757164734,-37.7440281828012));
#15651=CARTESIAN_POINT('Ctrl Pts',(1.95465267010927,-3.41289055482808,-37.7381621205116));
#15652=CARTESIAN_POINT('Ctrl Pts',(2.05555495924655,-3.35510114561209,-37.7322968303498));
#15653=CARTESIAN_POINT('Ctrl Pts',(2.15390718824994,-3.29282464947338,-37.7264315401879));
#15654=CARTESIAN_POINT('Ctrl Pts',(2.24929521998674,-3.22632298651961,-37.720566250026));
#15655=CARTESIAN_POINT('Ctrl Pts',(2.34469348397095,-3.1598141899511,-37.7147003306961));
#15656=CARTESIAN_POINT('Ctrl Pts',(2.4371265813273,-3.08907956066971,-37.7088344113662));
#15657=CARTESIAN_POINT('Ctrl Pts',(2.52621064934735,-3.01442345318704,-37.7029684920363));
#15658=CARTESIAN_POINT('Ctrl Pts',(2.61739236773523,-2.93800942855034,-37.696964448706));
#15659=CARTESIAN_POINT('Ctrl Pts',(2.70506501123355,-2.85748722065425,-37.6909604053758));
#15660=CARTESIAN_POINT('Ctrl Pts',(2.78885512983911,-2.77322484929911,-37.6849563620456));
#15661=CARTESIAN_POINT('Ctrl Pts',(2.87083753200744,-2.6907803829222,-37.6790818519825));
#15662=CARTESIAN_POINT('Ctrl Pts',(2.9491030055128,-2.60475585219117,-37.6732073419194));
#15663=CARTESIAN_POINT('Ctrl Pts',(3.02334183484842,-2.51553039132016,-37.6673328318563));
#15664=CARTESIAN_POINT('Ctrl Pts',(3.10003611953523,-2.4233537910344,-37.6612640218925));
#15665=CARTESIAN_POINT('Ctrl Pts',(3.1724324905158,-2.32776123575489,-37.6551952119287));
#15666=CARTESIAN_POINT('Ctrl Pts',(3.24023798824153,-2.22920317143962,-37.6491264019649));
#15667=CARTESIAN_POINT('Ctrl Pts',(3.30804348596726,-2.13064510712436,-37.6430575920011));
#15668=CARTESIAN_POINT('Ctrl Pts',(3.37125791289597,-2.02912197265364,-37.6369887820373));
#15669=CARTESIAN_POINT('Ctrl Pts',(3.42964097392287,-1.925110851351,-37.6309199720735));
#15670=CARTESIAN_POINT('Ctrl Pts',(3.48856666349948,-1.82013302150459,-37.6247947568871));
#15671=CARTESIAN_POINT('Ctrl Pts',(3.54274534667089,-1.71231104743553,-37.6186695417008));
#15672=CARTESIAN_POINT('Ctrl Pts',(3.59190567969494,-1.6020931896039,-37.6125443265145));
#15673=CARTESIAN_POINT('Ctrl Pts',(3.64098595593051,-1.4920548197291,-37.6064290861396));
#15674=CARTESIAN_POINT('Ctrl Pts',(3.68506401051628,-1.37962866589796,-37.6003138457648));
#15675=CARTESIAN_POINT('Ctrl Pts',(3.72391385284358,-1.26528835314314,-37.59419860539));
#15676=CARTESIAN_POINT('Ctrl Pts',(3.76268577704808,-1.15117736390669,-37.5880956298797));
#15677=CARTESIAN_POINT('Ctrl Pts',(3.79625027498637,-1.03516021058229,-37.5819926543693));
#15678=CARTESIAN_POINT('Ctrl Pts',(3.82442934891155,-0.917730437102317,
-37.575889678859));
#15679=CARTESIAN_POINT('Ctrl Pts',(3.85257463465805,-0.80044146804261,-37.5697940211344));
#15680=CARTESIAN_POINT('Ctrl Pts',(3.87534726934537,-0.681743602605054,
-37.5636983634099));
#15681=CARTESIAN_POINT('Ctrl Pts',(3.89261871291701,-0.562146382936252,
-37.5576027056853));
#15682=CARTESIAN_POINT('Ctrl Pts',(3.90986570691575,-0.442718465904437,
-37.5515156770153));
#15683=CARTESIAN_POINT('Ctrl Pts',(3.92162697995051,-0.322394090351545,
-37.5454286483452));
#15684=CARTESIAN_POINT('Ctrl Pts',(3.92782495184999,-0.201693201731384,
-37.5393416196752));
#15685=CARTESIAN_POINT('Ctrl Pts',(3.93127948698162,-0.134418701794884,
-37.5359489204618));
#15686=CARTESIAN_POINT('Ctrl Pts',(3.93300665744572,-0.0670274303798492,
-37.5325562212484));
#15687=CARTESIAN_POINT('Ctrl Pts',(3.93299998071214,0.000389510303426849,
-37.529163522035));
#15688=CARTESIAN_POINT('',(3.93299955983151,0.00186074317507175,-36.2791635220746));
#15689=CARTESIAN_POINT('Ctrl Pts',(3.93299998071207,0.000389511058542827,
-37.529163521997));
#15690=CARTESIAN_POINT('Ctrl Pts',(3.93298780586095,0.12332232175523,-37.5229770346553));
#15691=CARTESIAN_POINT('Ctrl Pts',(3.92720762809877,0.246130529403216,-37.5167905473136));
#15692=CARTESIAN_POINT('Ctrl Pts',(3.91572001853827,0.368273996392117,-37.5106040599719));
#15693=CARTESIAN_POINT('Ctrl Pts',(3.9040731652767,0.492110642248457,-37.5043318142194));
#15694=CARTESIAN_POINT('Ctrl Pts',(3.88655953275626,0.615263622070913,-37.4980595684668));
#15695=CARTESIAN_POINT('Ctrl Pts',(3.86329543211516,0.737182069910901,-37.4917873227142));
#15696=CARTESIAN_POINT('Ctrl Pts',(3.8402520103762,0.857944022185726,-37.4855745743103));
#15697=CARTESIAN_POINT('Ctrl Pts',(3.81156691509454,0.977494457883954,-37.4793618259063));
#15698=CARTESIAN_POINT('Ctrl Pts',(3.77740317841339,1.09531467063689,-37.4731490775024));
#15699=CARTESIAN_POINT('Ctrl Pts',(3.74274868024797,1.21482736870041,-37.4668470830755));
#15700=CARTESIAN_POINT('Ctrl Pts',(3.70245706381593,1.33255941114986,-37.4605450886486));
#15701=CARTESIAN_POINT('Ctrl Pts',(3.6567484231738,1.44799170219167,-37.4542430942217));
#15702=CARTESIAN_POINT('Ctrl Pts',(3.61103978253167,1.56342399323349,-37.4479410997948));
#15703=CARTESIAN_POINT('Ctrl Pts',(3.55991432357928,1.67655623474915,-37.441639105368));
#15704=CARTESIAN_POINT('Ctrl Pts',(3.50363957301195,1.78689639946602,-37.4353371109411));
#15705=CARTESIAN_POINT('Ctrl Pts',(3.4510897069913,1.88993303337576,-37.4294522521108));
#15706=CARTESIAN_POINT('Ctrl Pts',(3.39390730272993,1.99081327251063,-37.4235673932806));
#15707=CARTESIAN_POINT('Ctrl Pts',(3.33229321363909,2.08909332925431,-37.4176825344503));
#15708=CARTESIAN_POINT('Ctrl Pts',(3.27075630360959,2.18725027839971,-37.411805047114));
#15709=CARTESIAN_POINT('Ctrl Pts',(3.20479896627598,2.28281317765645,-37.4059275597776));
#15710=CARTESIAN_POINT('Ctrl Pts',(3.1346686596137,2.37536131871251,-37.4000500724412));
#15711=CARTESIAN_POINT('Ctrl Pts',(3.06460768476465,2.46781796536715,-37.394178395672));
#15712=CARTESIAN_POINT('Ctrl Pts',(2.99038219450984,2.55726545692151,-37.3883067189027));
#15713=CARTESIAN_POINT('Ctrl Pts',(2.91228344309494,2.64331120889597,-37.3824350421335));
#15714=CARTESIAN_POINT('Ctrl Pts',(2.83320898553806,2.73043195076685,-37.37649000912));
#15715=CARTESIAN_POINT('Ctrl Pts',(2.75016405047795,2.81406500967108,-37.3705449761064));
#15716=CARTESIAN_POINT('Ctrl Pts',(2.66349393190528,2.89383639390753,-37.3645999430929));
#15717=CARTESIAN_POINT('Ctrl Pts',(2.57798573639555,2.97253834138038,-37.3587346108007));
#15718=CARTESIAN_POINT('Ctrl Pts',(2.4889492809948,3.04748124265705,-37.3528692785085));
#15719=CARTESIAN_POINT('Ctrl Pts',(2.39675340126518,3.11834285054158,-37.3470039462163));
#15720=CARTESIAN_POINT('Ctrl Pts',(2.30456983732484,3.18919499252988,-37.341139397432));
#15721=CARTESIAN_POINT('Ctrl Pts',(2.20922801440525,3.25596667488358,-37.3352748486476));
#15722=CARTESIAN_POINT('Ctrl Pts',(2.11112903414671,3.3183765912239,-37.3294102998633));
#15723=CARTESIAN_POINT('Ctrl Pts',(2.01301970639734,3.38079309056882,-37.3235451324857));
#15724=CARTESIAN_POINT('Ctrl Pts',(1.91215299013068,3.43884668855458,-37.3176799651081));
#15725=CARTESIAN_POINT('Ctrl Pts',(1.80895749424776,3.49230035707195,-37.3118147977306));
#15726=CARTESIAN_POINT('Ctrl Pts',(1.70330089064088,3.54702884127131,-37.3058097520704));
#15727=CARTESIAN_POINT('Ctrl Pts',(1.59520342017676,3.59693499162826,-37.2998047064102));
#15728=CARTESIAN_POINT('Ctrl Pts',(1.48514886698982,3.64181573433896,-37.2937996607501));
#15729=CARTESIAN_POINT('Ctrl Pts',(1.37750077943175,3.68571510952235,-37.2879259221151));
#15730=CARTESIAN_POINT('Ctrl Pts',(1.26798073092691,3.72480651193384,-37.28205218348));
#15731=CARTESIAN_POINT('Ctrl Pts',(1.15705779767805,3.75895015301246,-37.276178444845));
#15732=CARTESIAN_POINT('Ctrl Pts',(1.042415352559,3.79423871222987,-37.2701077456723));
#15733=CARTESIAN_POINT('Ctrl Pts',(0.926274756106329,3.82424174301004,-37.2640370464995));
#15734=CARTESIAN_POINT('Ctrl Pts',(0.809165139064767,3.84886227055766,-37.2579663473268));
#15735=CARTESIAN_POINT('Ctrl Pts',(0.692055522023205,3.87348279810528,-37.2518956481541));
#15736=CARTESIAN_POINT('Ctrl Pts',(0.573977366695297,3.89272080910603,-37.2458249489814));
#15737=CARTESIAN_POINT('Ctrl Pts',(0.455464109096355,3.90653829436306,-37.2397542498086));
#15738=CARTESIAN_POINT('Ctrl Pts',(0.340581901548086,3.91993243474241,-37.2338695468104));
#15739=CARTESIAN_POINT('Ctrl Pts',(0.224925811904918,3.92827595135078,-37.2279848438122));
#15740=CARTESIAN_POINT('Ctrl Pts',(0.108976507804059,3.93148993649314,-37.2221001408139));
#15741=CARTESIAN_POINT('Ctrl Pts',(-0.00682755354633928,3.93469989566876,
-37.2162228092308));
#15742=CARTESIAN_POINT('Ctrl Pts',(-0.122923691200477,3.93279309178156,
-37.2103454776476));
#15743=CARTESIAN_POINT('Ctrl Pts',(-0.238824603734641,3.9257421984449,-37.2044681460644));
#15744=CARTESIAN_POINT('Ctrl Pts',(-0.354610937519859,3.91869827556706,
-37.198596624766));
#15745=CARTESIAN_POINT('Ctrl Pts',(-0.470202021859575,3.90652040463552,
-37.1927251034675));
#15746=CARTESIAN_POINT('Ctrl Pts',(-0.58510967706775,3.88923330051074,-37.1868535821691));
#15747=CARTESIAN_POINT('Ctrl Pts',(-0.701457123927851,3.87172958916202,
-37.1809084907736));
#15748=CARTESIAN_POINT('Ctrl Pts',(-0.817103469411767,3.8489877140398,-37.174963399378));
#15749=CARTESIAN_POINT('Ctrl Pts',(-0.931545990870102,3.82108768113136,
-37.1690183079825));
#15750=CARTESIAN_POINT('Ctrl Pts',(-1.04445019708959,3.79356267531286,-37.1631531294076));
#15751=CARTESIAN_POINT('Ctrl Pts',(-1.15618233507013,3.76101744065471,-37.1572879508327));
#15752=CARTESIAN_POINT('Ctrl Pts',(-1.26626974629447,3.72358025690589,-37.1514227722578));
#15753=CARTESIAN_POINT('Ctrl Pts',(-1.37634246908157,3.68614806822161,-37.1455583762456));
#15754=CARTESIAN_POINT('Ctrl Pts',(-1.48477051229725,3.64382536095392,-37.1396939802335));
#15755=CARTESIAN_POINT('Ctrl Pts',(-1.59109739978839,3.59678996667676,-37.1338295842213));
#15756=CARTESIAN_POINT('Ctrl Pts',(-1.69743552339359,3.54974960192537,-37.127964568488));
#15757=CARTESIAN_POINT('Ctrl Pts',(-1.80167167377429,3.49799572651596,-37.1220995527547));
#15758=CARTESIAN_POINT('Ctrl Pts',(-1.90337097343573,3.44175361370949,-37.1162345370214));
#15759=CARTESIAN_POINT('Ctrl Pts',(-2.00750214789092,3.38416661675006,-37.1102292746593));
#15760=CARTESIAN_POINT('Ctrl Pts',(-2.10897320448926,3.32187421780444,-37.1042240122972));
#15761=CARTESIAN_POINT('Ctrl Pts',(-2.20734685422763,3.25516648808189,-37.0982187499351));
#15762=CARTESIAN_POINT('Ctrl Pts',(-2.30356356729778,3.18992138934512,-37.0923451587129));
#15763=CARTESIAN_POINT('Ctrl Pts',(-2.39681700584095,3.12045288570387,-37.0864715674906));
#15764=CARTESIAN_POINT('Ctrl Pts',(-2.48673078417477,3.04707384338442,-37.0805979762683));
#15765=CARTESIAN_POINT('Ctrl Pts',(-2.57966802359885,2.97122734075573,-37.0745268783363));
#15766=CARTESIAN_POINT('Ctrl Pts',(-2.66903668757966,2.89120300019649,-37.0684557804043));
#15767=CARTESIAN_POINT('Ctrl Pts',(-2.75446262885671,2.80738750909663,-37.0623846824723));
#15768=CARTESIAN_POINT('Ctrl Pts',(-2.83988857013377,2.72357201799677,-37.0563135845403));
#15769=CARTESIAN_POINT('Ctrl Pts',(-2.92137151010482,2.63596577058062,-37.0502424866083));
#15770=CARTESIAN_POINT('Ctrl Pts',(-2.9985840061201,2.54499174030894,-37.0441713886763));
#15771=CARTESIAN_POINT('Ctrl Pts',(-3.07342358424983,2.45681355157449,-37.0382868695704));
#15772=CARTESIAN_POINT('Ctrl Pts',(-3.14448935456177,2.36519118784049,-37.0324023504645));
#15773=CARTESIAN_POINT('Ctrl Pts',(-3.21144914123017,2.27048087710335,-37.0265178313586));
#15774=CARTESIAN_POINT('Ctrl Pts',(-3.27832500925433,2.17588926389002,-37.0206406871397));
#15775=CARTESIAN_POINT('Ctrl Pts',(-3.34110489296003,2.0782177338312,-37.0147635429209));
#15776=CARTESIAN_POINT('Ctrl Pts',(-3.39949586273868,1.97785663768197,-37.0088863987021));
#15777=CARTESIAN_POINT('Ctrl Pts',(-3.45782907389752,1.87759481575984,-37.0030150679804));
#15778=CARTESIAN_POINT('Ctrl Pts',(-3.51178180185997,1.77464907379141,-36.9971437372588));
#15779=CARTESIAN_POINT('Ctrl Pts',(-3.56110393773355,1.66943935039839,-36.9912724065372));
#15780=CARTESIAN_POINT('Ctrl Pts',(-3.61104629038695,1.56290663409979,-36.9853272449124));
#15781=CARTESIAN_POINT('Ctrl Pts',(-3.6562405417712,1.45405295409796,-36.9793820832877));
#15782=CARTESIAN_POINT('Ctrl Pts',(-3.69647450474803,1.34334107200957,-36.973436921663));
#15783=CARTESIAN_POINT('Ctrl Pts',(-3.73616584641738,1.23412232213505,-36.9675719403421));
#15784=CARTESIAN_POINT('Ctrl Pts',(-3.77102973583569,1.12309558453723,-36.9617069590211));
#15785=CARTESIAN_POINT('Ctrl Pts',(-3.80091085821922,1.01072530782168,-36.9558419777002));
#15786=CARTESIAN_POINT('Ctrl Pts',(-3.83078798260546,0.898370065884793,
-36.9499777810948));
#15787=CARTESIAN_POINT('Ctrl Pts',(-3.85568356019966,0.78467203972006,-36.9441135844893));
#15788=CARTESIAN_POINT('Ctrl Pts',(-3.87549248587364,0.670109686496867,
-36.9382493878839));
#15789=CARTESIAN_POINT('Ctrl Pts',(-3.89530349840427,0.555535264208808,
-36.9323845734893));
#15790=CARTESIAN_POINT('Ctrl Pts',(-3.91002672365672,0.440096739119747,
-36.9265197590948));
#15791=CARTESIAN_POINT('Ctrl Pts',(-3.9196085134202,0.324280899104241,-36.9206549447003));
#15792=CARTESIAN_POINT('Ctrl Pts',(-3.92942020866677,0.205686173587696,
-36.9146494099373));
#15793=CARTESIAN_POINT('Ctrl Pts',(-3.93384054987489,0.0866962472526169,
-36.9086438751742));
#15794=CARTESIAN_POINT('Ctrl Pts',(-3.93286847923819,-0.0321640329351796,
-36.9026383404112));
#15795=CARTESIAN_POINT('Ctrl Pts',(-3.93191779837726,-0.148408870742695,
-36.8967649534953));
#15796=CARTESIAN_POINT('Ctrl Pts',(-3.9258096503033,-0.26452929666638,-36.8908915665794));
#15797=CARTESIAN_POINT('Ctrl Pts',(-3.91459571819556,-0.380038633674274,
-36.8850181796635));
#15798=CARTESIAN_POINT('Ctrl Pts',(-3.9030033254976,-0.499446311731457,
-36.8789465709769));
#15799=CARTESIAN_POINT('Ctrl Pts',(-3.88595449812792,-0.618200444421965,
-36.8728749622903));
#15800=CARTESIAN_POINT('Ctrl Pts',(-3.86356363957789,-0.735775103500807,
-36.8668033536037));
#15801=CARTESIAN_POINT('Ctrl Pts',(-3.84117278102787,-0.853349762579648,
-36.8607317449171));
#15802=CARTESIAN_POINT('Ctrl Pts',(-3.81344006503029,-0.969744497313235,
-36.8546601362305));
#15803=CARTESIAN_POINT('Ctrl Pts',(-3.78053601460536,-1.08445213922598,
-36.8485885275439));
#15804=CARTESIAN_POINT('Ctrl Pts',(-3.74864509202635,-1.19562789054591,
-36.8427038659276));
#15805=CARTESIAN_POINT('Ctrl Pts',(-3.71179525530777,-1.30557241359153,
-36.8368192043114));
#15806=CARTESIAN_POINT('Ctrl Pts',(-3.67009882187724,-1.41381174052817,
-36.8309345426952));
#15807=CARTESIAN_POINT('Ctrl Pts',(-3.62845463042516,-1.52191545306999,
-36.8250572540444));
#15808=CARTESIAN_POINT('Ctrl Pts',(-3.58197606627379,-1.62831783820295,
-36.8191799653937));
#15809=CARTESIAN_POINT('Ctrl Pts',(-3.53082560359532,-1.73255867346411,
-36.813302676743));
#15810=CARTESIAN_POINT('Ctrl Pts',(-3.47972572118794,-1.83669642989805,
-36.8074311998648));
#15811=CARTESIAN_POINT('Ctrl Pts',(-3.42396331078167,-1.93867652136449,
-36.8015597229865));
#15812=CARTESIAN_POINT('Ctrl Pts',(-3.36374921089127,-2.038057959487,-36.7956882461083));
#15813=CARTESIAN_POINT('Ctrl Pts',(-3.30278000271274,-2.13868567958914,
-36.789743138621));
#15814=CARTESIAN_POINT('Ctrl Pts',(-3.23724683771426,-2.23664872183403,
-36.7837980311336));
#15815=CARTESIAN_POINT('Ctrl Pts',(-3.16741718972646,-2.33151396011805,
-36.7778529236462));
#15816=CARTESIAN_POINT('Ctrl Pts',(-3.09852692699529,-2.42510302117965,
-36.7719877928806));
#15817=CARTESIAN_POINT('Ctrl Pts',(-3.02545532729194,-2.5156767780483,-36.7661226621149));
#15818=CARTESIAN_POINT('Ctrl Pts',(-2.94850282556456,-2.60284845652562,
-36.7602575313492));
#15819=CARTESIAN_POINT('Ctrl Pts',(-2.87156060692803,-2.69000848633306,
-36.7543931843355));
#15820=CARTESIAN_POINT('Ctrl Pts',(-2.79073878978542,-2.77376703366651,
-36.7485288373217));
#15821=CARTESIAN_POINT('Ctrl Pts',(-2.70637730467253,-2.85377134416082,
-36.742664490308));
#15822=CARTESIAN_POINT('Ctrl Pts',(-2.6220069209459,-2.9337840936656,-36.7367995247115));
#15823=CARTESIAN_POINT('Ctrl Pts',(-2.53409642542111,-3.01004153610371,
-36.7309345591151));
#15824=CARTESIAN_POINT('Ctrl Pts',(-2.44302121061884,-3.08222912264265,
-36.7250695935186));
#15825=CARTESIAN_POINT('Ctrl Pts',(-2.34976636349886,-3.15614431857455,
-36.7190642662597));
#15826=CARTESIAN_POINT('Ctrl Pts',(-2.25319374342195,-3.22579209143481,
-36.7130589390007));
#15827=CARTESIAN_POINT('Ctrl Pts',(-2.15373949565974,-3.29088060932561,
-36.7070536117418));
#15828=CARTESIAN_POINT('Ctrl Pts',(-2.05646779870621,-3.35454074179745,
-36.7011800730406));
#15829=CARTESIAN_POINT('Ctrl Pts',(-1.95644003669387,-3.41383950676763,
-36.6953065343393));
#15830=CARTESIAN_POINT('Ctrl Pts',(-1.8540899073174,-3.46855007396228,-36.6894329956381));
#15831=CARTESIAN_POINT('Ctrl Pts',(-1.74829502939687,-3.52510200811794,
-36.6833617741003));
#15832=CARTESIAN_POINT('Ctrl Pts',(-1.640019142131,-3.57675124888194,-36.6772905525626));
#15833=CARTESIAN_POINT('Ctrl Pts',(-1.52976325021857,-3.62330145009778,
-36.6712193310248));
#15834=CARTESIAN_POINT('Ctrl Pts',(-1.41950735830614,-3.66985165131363,
-36.6651481094871));
#15835=CARTESIAN_POINT('Ctrl Pts',(-1.30727193294276,-3.71130270770446,
-36.6590768879493));
#15836=CARTESIAN_POINT('Ctrl Pts',(-1.19357347707007,-3.74751535751821,
-36.6530056664116));
#15837=CARTESIAN_POINT('Ctrl Pts',(-1.08336942808624,-3.78261504821566,
-36.6471210377189));
#15838=CARTESIAN_POINT('Ctrl Pts',(-0.971440620823848,-3.81290523254181,
-36.6412364090263));
#15839=CARTESIAN_POINT('Ctrl Pts',(-0.85824376992436,-3.83821659516318,
-36.6353517803337));
#15840=CARTESIAN_POINT('Ctrl Pts',(-0.745188749241536,-3.86349624386304,
-36.6294745247981));
#15841=CARTESIAN_POINT('Ctrl Pts',(-0.630869242885877,-3.88380938917106,
-36.6235972692625));
#15842=CARTESIAN_POINT('Ctrl Pts',(-0.515758335612414,-3.89903607821809,
-36.617720013727));
#15843=CARTESIAN_POINT('Ctrl Pts',(-0.400761259595107,-3.91424770984631,
-36.6118485701114));
#15844=CARTESIAN_POINT('Ctrl Pts',(-0.284974745011976,-3.92438283772759,
-36.6059771264958));
#15845=CARTESIAN_POINT('Ctrl Pts',(-0.168882685058675,-3.92937242300693,
-36.6001056828802));
#15846=CARTESIAN_POINT('Ctrl Pts',(-0.0513338740589549,-3.93442461880055,
-36.5941605629802));
#15847=CARTESIAN_POINT('Ctrl Pts',(0.0665277857892527,-3.9342011533646,
-36.5882154430801));
#15848=CARTESIAN_POINT('Ctrl Pts',(0.184193531576616,-3.9286844799405,-36.5822703231801));
#15849=CARTESIAN_POINT('Ctrl Pts',(0.300275472207089,-3.92324206207615,
-36.5764052258175));
#15850=CARTESIAN_POINT('Ctrl Pts',(0.41616631817684,-3.91264808560998,-36.570540128455));
#15851=CARTESIAN_POINT('Ctrl Pts',(0.531377618227846,-3.89693813484978,
-36.5646750310925));
#15852=CARTESIAN_POINT('Ctrl Pts',(0.646573522784248,-3.8812302833842,-36.5588107174732));
#15853=CARTESIAN_POINT('Ctrl Pts',(0.761089654624889,-3.86040787282167,
-36.5529464038538));
#15854=CARTESIAN_POINT('Ctrl Pts',(0.874443976543163,-3.83455821860712,
-36.5470820902345));
#15855=CARTESIAN_POINT('Ctrl Pts',(0.987810256284547,-3.80870583749528,
-36.5412171579848));
#15856=CARTESIAN_POINT('Ctrl Pts',(1.10001408148965,-3.77782524991446,-36.5353522257352));
#15857=CARTESIAN_POINT('Ctrl Pts',(1.21058554890604,-3.74205446630322,-36.5294872934855));
#15858=CARTESIAN_POINT('Ctrl Pts',(1.32380476256398,-3.70542711489852,-36.5234819194683));
#15859=CARTESIAN_POINT('Ctrl Pts',(1.43531201249615,-3.66367251754737,-36.5174765454511));
#15860=CARTESIAN_POINT('Ctrl Pts',(1.54462259819798,-3.61699184808815,-36.5114711714339));
#15861=CARTESIAN_POINT('Ctrl Pts',(1.65153290144412,-3.57133621011333,-36.5055976656507));
#15862=CARTESIAN_POINT('Ctrl Pts',(1.75634166794661,-3.52096884273536,-36.4997241598675));
#15863=CARTESIAN_POINT('Ctrl Pts',(1.85861966962177,-3.46612491461215,-36.4938506540843));
#15864=CARTESIAN_POINT('Ctrl Pts',(1.96434209272642,-3.40943400475082,-36.4877793459501));
#15865=CARTESIAN_POINT('Ctrl Pts',(2.06735987213064,-3.34795995271331,-36.4817080378159));
#15866=CARTESIAN_POINT('Ctrl Pts',(2.16723180649855,-3.28201086178901,-36.4756367296817));
#15867=CARTESIAN_POINT('Ctrl Pts',(2.26710374086646,-3.2160617708647,-36.4695654215475));
#15868=CARTESIAN_POINT('Ctrl Pts',(2.36382948129902,-3.14563797486531,-36.4634941134134));
#15869=CARTESIAN_POINT('Ctrl Pts',(2.45700674411374,-3.07109212811657,-36.4574228052792));
#15870=CARTESIAN_POINT('Ctrl Pts',(2.54629870464434,-2.99965469150884,-36.4516046583417));
#15871=CARTESIAN_POINT('Ctrl Pts',(2.63263057261756,-2.92419311716659,-36.4457865114042));
#15872=CARTESIAN_POINT('Ctrl Pts',(2.71561293937094,-2.84498424662091,-36.4399683644668));
#15873=CARTESIAN_POINT('Ctrl Pts',(2.79849071779156,-2.76587520841352,-36.4341575505364));
#15874=CARTESIAN_POINT('Ctrl Pts',(2.8780270851052,-2.68302855163472,-36.4283467366061));
#15875=CARTESIAN_POINT('Ctrl Pts',(2.95386421551895,-2.59676244509902,-36.4225359226758));
#15876=CARTESIAN_POINT('Ctrl Pts',(3.03182913555492,-2.50807593941009,-36.4165620726507));
#15877=CARTESIAN_POINT('Ctrl Pts',(3.10588379397672,-2.4157755201198,-36.4105882226257));
#15878=CARTESIAN_POINT('Ctrl Pts',(3.17567818472388,-2.32024935450241,-36.4046143726006));
#15879=CARTESIAN_POINT('Ctrl Pts',(3.24345393473171,-2.22748606148154,-36.3988133023205));
#15880=CARTESIAN_POINT('Ctrl Pts',(3.30721219521597,-2.13168141618424,-36.3930122320404));
#15881=CARTESIAN_POINT('Ctrl Pts',(3.36667258369661,-2.03322520006654,-36.3872111617603));
#15882=CARTESIAN_POINT('Ctrl Pts',(3.42611307370171,-1.93480193241516,-36.3814120328139));
#15883=CARTESIAN_POINT('Ctrl Pts',(3.48125833276999,-1.83372921829553,-36.3756129038674));
#15884=CARTESIAN_POINT('Ctrl Pts',(3.53187167650335,-1.73042522540368,-36.369813774921));
#15885=CARTESIAN_POINT('Ctrl Pts',(3.58248089321154,-1.6271296559462,-36.3640151188371));
#15886=CARTESIAN_POINT('Ctrl Pts',(3.62855874456104,-1.52160354849334,-36.3582164627531));
#15887=CARTESIAN_POINT('Ctrl Pts',(3.66991520746485,-1.41428829098534,-36.3524178066691));
#15888=CARTESIAN_POINT('Ctrl Pts',(3.7134531419379,-1.30131236603235,-36.3463132829529));
#15889=CARTESIAN_POINT('Ctrl Pts',(3.7517578077341,-1.18635386797593,-36.3402087592367));
#15890=CARTESIAN_POINT('Ctrl Pts',(3.78466629066775,-1.06994862880571,-36.3341042355205));
#15891=CARTESIAN_POINT('Ctrl Pts',(3.81596056636101,-0.959253229869264,
-36.3282991472539));
#15892=CARTESIAN_POINT('Ctrl Pts',(3.84237541622021,-0.847250085037127,
-36.3224940589872));
#15893=CARTESIAN_POINT('Ctrl Pts',(3.86382307213103,-0.734411510849277,
-36.3166889707206));
#15894=CARTESIAN_POINT('Ctrl Pts',(3.88528287947158,-0.62150900659791,-36.3108805935107));
#15895=CARTESIAN_POINT('Ctrl Pts',(3.90176983066044,-0.507770547286545,
-36.3050722163009));
#15896=CARTESIAN_POINT('Ctrl Pts',(3.9132479705996,-0.39367412995792,-36.299263839091));
#15897=CARTESIAN_POINT('Ctrl Pts',(3.92474076857546,-0.279432007011314,
-36.2934480443547));
#15898=CARTESIAN_POINT('Ctrl Pts',(3.93121197153682,-0.164831433445106,
-36.2876322496185));
#15899=CARTESIAN_POINT('Ctrl Pts',(3.93267768806338,-0.0503507875654495,
-36.2818164548822));
#15900=CARTESIAN_POINT('Ctrl Pts',(3.93290055513694,-0.032943624540109,
-36.2809321439463));
#15901=CARTESIAN_POINT('Ctrl Pts',(3.93300779193799,-0.0155392245317547,
-36.2800478330105));
#15902=CARTESIAN_POINT('Ctrl Pts',(3.93299955983151,0.00186074317507913,
-36.2791635220746));
#15903=CARTESIAN_POINT('',(3.93270531513622,-0.00309687980344829,-35.0291635502465));
#15904=CARTESIAN_POINT('Ctrl Pts',(3.93299955983114,0.0018607439544177,
-36.279163522035));
#15905=CARTESIAN_POINT('Ctrl Pts',(3.93294580438091,0.1154820520235,-36.2733889960723));
#15906=CARTESIAN_POINT('Ctrl Pts',(3.92796871631761,0.22897989575827,-36.2676144701095));
#15907=CARTESIAN_POINT('Ctrl Pts',(3.91809833470597,0.34204449940656,-36.2618399441467));
#15908=CARTESIAN_POINT('Ctrl Pts',(3.90803975391883,0.457264912832259,-36.2559553149409));
#15909=CARTESIAN_POINT('Ctrl Pts',(3.89287842309005,0.572224409020614,-36.2500706857351));
#15910=CARTESIAN_POINT('Ctrl Pts',(3.87263401463472,0.686436296166057,-36.2441860565294));
#15911=CARTESIAN_POINT('Ctrl Pts',(3.85241497185978,0.800505078995474,-36.2383088006002));
#15912=CARTESIAN_POINT('Ctrl Pts',(3.82712558994851,0.913827714317787,-36.2324315446711));
#15913=CARTESIAN_POINT('Ctrl Pts',(3.79683740043307,1.02592141739639,-36.226554288742));
#15914=CARTESIAN_POINT('Ctrl Pts',(3.76657916301714,1.13790427060902,-36.2206828448524));
#15915=CARTESIAN_POINT('Ctrl Pts',(3.73133205862219,1.24866021433365,-36.2148114009628));
#15916=CARTESIAN_POINT('Ctrl Pts',(3.6912187674152,1.35771610106155,-36.2089399570732));
#15917=CARTESIAN_POINT('Ctrl Pts',(3.65060212790096,1.46814043935075,-36.2029948373208));
#15918=CARTESIAN_POINT('Ctrl Pts',(3.60499641086151,1.57682134006441,-36.1970497175683));
#15919=CARTESIAN_POINT('Ctrl Pts',(3.55458139483645,1.68328253941,-36.1911045978158));
#15920=CARTESIAN_POINT('Ctrl Pts',(3.50484497427593,1.78831075127046,-36.1852395004777));
#15921=CARTESIAN_POINT('Ctrl Pts',(3.45042811731104,1.89117827149154,-36.1793744031396));
#15922=CARTESIAN_POINT('Ctrl Pts',(3.39155180991,1.99144804619558,-36.1735093058015));
#15923=CARTESIAN_POINT('Ctrl Pts',(3.3326833711807,2.09170442009413,-36.167644992319));
#15924=CARTESIAN_POINT('Ctrl Pts',(3.26935687554114,2.18936338440196,-36.1617806788365));
#15925=CARTESIAN_POINT('Ctrl Pts',(3.20183857770775,2.28401373076048,-36.155916365354));
#15926=CARTESIAN_POINT('Ctrl Pts',(3.13431315862322,2.37867406002599,-36.150051433354));
#15927=CARTESIAN_POINT('Ctrl Pts',(3.06259529728359,2.4703248057144,-36.1441865013541));
#15928=CARTESIAN_POINT('Ctrl Pts',(2.98699335770534,2.55858548440817,-36.1383215693541));
#15929=CARTESIAN_POINT('Ctrl Pts',(2.90958105150426,2.64895965632323,-36.1323161954925));
#15930=CARTESIAN_POINT('Ctrl Pts',(2.82809657227961,2.73577898797125,-36.1263108216309));
#15931=CARTESIAN_POINT('Ctrl Pts',(2.74291227337743,2.81867367046195,-36.1203054477693));
#15932=CARTESIAN_POINT('Ctrl Pts',(2.65959848831895,2.89974811550085,-36.1144319425159));
#15933=CARTESIAN_POINT('Ctrl Pts',(2.57274604487698,2.97706826223606,-36.1085584372626));
#15934=CARTESIAN_POINT('Ctrl Pts',(2.48273730049492,3.05032858832146,-36.1026849320093));
#15935=CARTESIAN_POINT('Ctrl Pts',(2.38969731820365,3.1260561133351,-36.0966136238435));
#15936=CARTESIAN_POINT('Ctrl Pts',(2.29328508670429,3.19744526217168,-36.0905423156778));
#15937=CARTESIAN_POINT('Ctrl Pts',(2.19395488236274,3.26420755684388,-36.084471007512));
#15938=CARTESIAN_POINT('Ctrl Pts',(2.0946246780212,3.33096985151608,-36.0783996993462));
#15939=CARTESIAN_POINT('Ctrl Pts',(1.99237694328402,3.39310509862785,-36.0723283911805));
#15940=CARTESIAN_POINT('Ctrl Pts',(1.88769207713821,3.45037789552241,-36.0662570830147));
#15941=CARTESIAN_POINT('Ctrl Pts',(1.78622613205874,3.50588962972243,-36.0603724595386));
#15942=CARTESIAN_POINT('Ctrl Pts',(1.68214816344238,3.55701008158881,-36.0544878360626));
#15943=CARTESIAN_POINT('Ctrl Pts',(1.57587411384908,3.6034857814761,-36.0486032125865));
#15944=CARTESIAN_POINT('Ctrl Pts',(1.46973322370741,3.64990324815655,-36.0427259624367));
#15945=CARTESIAN_POINT('Ctrl Pts',(1.36140209902872,3.69168737452847,-36.0368487122868));
#15946=CARTESIAN_POINT('Ctrl Pts',(1.25132218365477,3.72863001552761,-36.0309714621369));
#15947=CARTESIAN_POINT('Ctrl Pts',(1.1413511275954,3.7655361235174,-36.0251000240684));
#15948=CARTESIAN_POINT('Ctrl Pts',(1.02963510896131,3.79761014051247,-36.0192285859999));
#15949=CARTESIAN_POINT('Ctrl Pts',(0.916635910175047,3.82469183179215,-36.0133571479314));
#15950=CARTESIAN_POINT('Ctrl Pts',(0.802218623360296,3.85211338585499,-36.0074120260127));
#15951=CARTESIAN_POINT('Ctrl Pts',(0.686486119662203,3.87441627606722,-36.0014669040939));
#15952=CARTESIAN_POINT('Ctrl Pts',(0.569934434622809,3.89148605808002,-35.9955217821752));
#15953=CARTESIAN_POINT('Ctrl Pts',(0.454951714153902,3.9083260546273,-35.9896566907224));
#15954=CARTESIAN_POINT('Ctrl Pts',(0.339172151849051,3.92007291688466,-35.9837915992696));
#15955=CARTESIAN_POINT('Ctrl Pts',(0.223081996925893,3.92666823434926,-35.9779265078168));
#15956=CARTESIAN_POINT('Ctrl Pts',(0.107007357442921,3.9332626703502,-35.972062200233));
#15957=CARTESIAN_POINT('Ctrl Pts',(-0.00937738159519706,3.93470690755665,
-35.9661978926492));
#15958=CARTESIAN_POINT('Ctrl Pts',(-0.125582381397877,3.93099453897896,
-35.9603335850654));
#15959=CARTESIAN_POINT('Ctrl Pts',(-0.241799637389512,3.92728177885624,
-35.9544686589707));
#15960=CARTESIAN_POINT('Ctrl Pts',(-0.357836705402596,3.91841134490497,
-35.948603732876));
#15961=CARTESIAN_POINT('Ctrl Pts',(-0.473205969581352,3.90442890962975,
-35.9427388067813));
#15962=CARTESIAN_POINT('Ctrl Pts',(-0.591338150602947,3.89011161648575,
-35.9367334247064));
#15963=CARTESIAN_POINT('Ctrl Pts',(-0.708769683599898,3.87043440316512,
-35.9307280426314));
#15964=CARTESIAN_POINT('Ctrl Pts',(-0.824986354483205,3.84550211479808,
-35.9247226605565));
#15965=CARTESIAN_POINT('Ctrl Pts',(-0.938650820224721,3.82111735815849,
-35.9188491611701));
#15966=CARTESIAN_POINT('Ctrl Pts',(-1.0511528452843,3.79170612251139,-35.9129756617836));
#15967=CARTESIAN_POINT('Ctrl Pts',(-1.16202617332701,3.75741722097813,-35.9071021623973));
#15968=CARTESIAN_POINT('Ctrl Pts',(-1.27663380139134,3.72197344254167,-35.901030838978));
#15969=CARTESIAN_POINT('Ctrl Pts',(-1.38950063021121,3.6813178026479,-35.8949595155588));
#15970=CARTESIAN_POINT('Ctrl Pts',(-1.50013470844846,3.63566841949431,-35.8888881921396));
#15971=CARTESIAN_POINT('Ctrl Pts',(-1.61076878668571,3.59001903634072,-35.8828168687204));
#15972=CARTESIAN_POINT('Ctrl Pts',(-1.71916970807392,3.53937617092121,-35.8767455453012));
#15973=CARTESIAN_POINT('Ctrl Pts',(-1.8248752088951,3.48400910905239,-35.870674221882));
#15974=CARTESIAN_POINT('Ctrl Pts',(-1.92733012257181,3.43034465923442,-35.8647895998709));
#15975=CARTESIAN_POINT('Ctrl Pts',(-2.02757871867464,3.37207172169912,-35.8589049778599));
#15976=CARTESIAN_POINT('Ctrl Pts',(-2.1251794386981,3.30939591970118,-35.8530203558489));
#15977=CARTESIAN_POINT('Ctrl Pts',(-2.22265786611653,3.24679864977858,-35.8471431072031));
#15978=CARTESIAN_POINT('Ctrl Pts',(-2.31749467305084,3.17980970808052,-35.8412658585573));
#15979=CARTESIAN_POINT('Ctrl Pts',(-2.40927188222961,3.10868107040555,-35.8353886099115));
#15980=CARTESIAN_POINT('Ctrl Pts',(-2.50095833125454,3.03762277313595,-35.829517173384));
#15981=CARTESIAN_POINT('Ctrl Pts',(-2.58959087832125,2.9624331744105,-35.8236457368564));
#15982=CARTESIAN_POINT('Ctrl Pts',(-2.67478014173756,2.88340773970079,-35.8177743003289));
#15983=CARTESIAN_POINT('Ctrl Pts',(-2.76103852208886,2.8033905435043,-35.8118291778464));
#15984=CARTESIAN_POINT('Ctrl Pts',(-2.84376623716277,2.71944079991931,-35.8058840553639));
#15985=CARTESIAN_POINT('Ctrl Pts',(-2.92259302138893,2.63190786908066,-35.7999389328815));
#15986=CARTESIAN_POINT('Ctrl Pts',(-3.00035864723054,2.54555329791248,-35.7940738430508));
#15987=CARTESIAN_POINT('Ctrl Pts',(-3.07432744876471,2.45571174070017,-35.78820875322));
#15988=CARTESIAN_POINT('Ctrl Pts',(-3.1441812194431,2.36275548021824,-35.7823436633893));
#15989=CARTESIAN_POINT('Ctrl Pts',(-3.21402565383958,2.26981164377361,-35.7764793574551));
#15990=CARTESIAN_POINT('Ctrl Pts',(-3.2797559042162,2.17375426070261,-35.770615051521));
#15991=CARTESIAN_POINT('Ctrl Pts',(-3.34109505236939,2.07498743394576,-35.7647507455869));
#15992=CARTESIAN_POINT('Ctrl Pts',(-3.40244066971976,1.97621019064259,-35.7588858211676));
#15993=CARTESIAN_POINT('Ctrl Pts',(-3.4593940472322,1.87472328496582,-35.7530208967483));
#15994=CARTESIAN_POINT('Ctrl Pts',(-3.51172284097113,1.77095784484036,-35.747155972329));
#15995=CARTESIAN_POINT('Ctrl Pts',(-3.56530486416553,1.66470731196324,-35.7411505880307));
#15996=CARTESIAN_POINT('Ctrl Pts',(-3.61403776324045,1.55606811915416,-35.7351452037325));
#15997=CARTESIAN_POINT('Ctrl Pts',(-3.6577236916246,1.44552633864904,-35.7291398194342));
#15998=CARTESIAN_POINT('Ctrl Pts',(-3.7004502159369,1.33741221021058,-35.7232663217722));
#15999=CARTESIAN_POINT('Ctrl Pts',(-3.73834908375054,1.2274786129651,-35.7173928241103));
#16000=CARTESIAN_POINT('Ctrl Pts',(-3.77128562979908,1.11619608423921,-35.7115193264483));
#16001=CARTESIAN_POINT('Ctrl Pts',(-3.80533153789732,1.00116535999881,-35.7054479988319));
#16002=CARTESIAN_POINT('Ctrl Pts',(-3.83407483448959,0.884693704268451,
-35.6993766712155));
#16003=CARTESIAN_POINT('Ctrl Pts',(-3.85742428506768,0.767311465423337,
-35.693305343599));
#16004=CARTESIAN_POINT('Ctrl Pts',(-3.88077373564577,0.649929226578227,
-35.6872340159826));
#16005=CARTESIAN_POINT('Ctrl Pts',(-3.89872933216462,0.53163688743102,-35.6811626883662));
#16006=CARTESIAN_POINT('Ctrl Pts',(-3.91125888325936,0.412968458995048,
-35.6750913607497));
#16007=CARTESIAN_POINT('Ctrl Pts',(-3.92340313000817,0.297949280309227,
-35.6692067364636));
#16008=CARTESIAN_POINT('Ctrl Pts',(-3.93048880854725,0.18221112392774,-35.6633221121774));
#16009=CARTESIAN_POINT('Ctrl Pts',(-3.93244222618923,0.0662354714927022,
-35.6574374878913));
#16010=CARTESIAN_POINT('Ctrl Pts',(-3.93439319623325,-0.0495948654887856,
-35.6515602369359));
#16011=CARTESIAN_POINT('Ctrl Pts',(-3.93122468849843,-0.165661698915492,
-35.6456829859805));
#16012=CARTESIAN_POINT('Ctrl Pts',(-3.92291466037067,-0.28147747236472,
-35.6398057350251));
#16013=CARTESIAN_POINT('Ctrl Pts',(-3.91461285013363,-0.397178714147654,
-35.6339342961567));
#16014=CARTESIAN_POINT('Ctrl Pts',(-3.90117966355049,-0.512628981876277,
-35.6280628572882));
#16015=CARTESIAN_POINT('Ctrl Pts',(-3.88264510567778,-0.627340404689822,
-35.6221914184198));
#16016=CARTESIAN_POINT('Ctrl Pts',(-3.86387795112926,-0.743491381433198,
-35.616246296803));
#16017=CARTESIAN_POINT('Ctrl Pts',(-3.83988049751041,-0.858884413607845,
-35.6103011751863));
#16018=CARTESIAN_POINT('Ctrl Pts',(-3.81073820089442,-0.973017658752366,
-35.6043560535695));
#16019=CARTESIAN_POINT('Ctrl Pts',(-3.78198819903342,-1.08561451594403,
-35.5984909613361));
#16020=CARTESIAN_POINT('Ctrl Pts',(-3.74823113030102,-1.19698488693604,
-35.5926258691027));
#16021=CARTESIAN_POINT('Ctrl Pts',(-3.70960039123802,-1.30665754401324,
-35.5867607768693));
#16022=CARTESIAN_POINT('Ctrl Pts',(-3.67097481522704,-1.41631554318725,
-35.5808964685136));
#16023=CARTESIAN_POINT('Ctrl Pts',(-3.62747700096022,-1.5242758919045,-35.5750321601579));
#16024=CARTESIAN_POINT('Ctrl Pts',(-3.57928971837202,-1.63008408125358,
-35.5691678518023));
#16025=CARTESIAN_POINT('Ctrl Pts',(-3.53109735353148,-1.73590343005989,
-35.5633029249453));
#16026=CARTESIAN_POINT('Ctrl Pts',(-3.47821470760771,-1.83956979398554,
-35.5574379980884));
#16027=CARTESIAN_POINT('Ctrl Pts',(-3.42087175511027,-1.94065077618019,
-35.5515730712315));
#16028=CARTESIAN_POINT('Ctrl Pts',(-3.36215554534861,-2.04415246025761,
-35.5455676902637));
#16029=CARTESIAN_POINT('Ctrl Pts',(-3.29876289481269,-2.14494295784491,
-35.5395623092958));
#16030=CARTESIAN_POINT('Ctrl Pts',(-3.23098862981859,-2.24258811955806,
-35.533556928328));
#16031=CARTESIAN_POINT('Ctrl Pts',(-3.16470271797934,-2.33808894987192,
-35.5276834282106));
#16032=CARTESIAN_POINT('Ctrl Pts',(-3.09422595330723,-2.43058087239799,
-35.5218099280933));
#16033=CARTESIAN_POINT('Ctrl Pts',(-3.01987526464141,-2.51969093065141,
-35.5159364279759));
#16034=CARTESIAN_POINT('Ctrl Pts',(-2.94302042209953,-2.61180224285117,
-35.5098651065828));
#16035=CARTESIAN_POINT('Ctrl Pts',(-2.86202643257968,-2.70029951224006,
-35.5037937851897));
#16036=CARTESIAN_POINT('Ctrl Pts',(-2.77728407914598,-2.78481276636729,
-35.4977224637966));
#16037=CARTESIAN_POINT('Ctrl Pts',(-2.69254172571229,-2.86932602049453,
-35.4916511424035));
#16038=CARTESIAN_POINT('Ctrl Pts',(-2.60405140570917,-2.9498549849764,-35.4855798210104));
#16039=CARTESIAN_POINT('Ctrl Pts',(-2.51223968600886,-3.02607679348064,
-35.4795084996174));
#16040=CARTESIAN_POINT('Ctrl Pts',(-2.4232512504495,-3.09995472013793,-35.4736238762347));
#16041=CARTESIAN_POINT('Ctrl Pts',(-2.3308597938181,-3.17002141713106,-35.4677392528521));
#16042=CARTESIAN_POINT('Ctrl Pts',(-2.23542515827695,-3.23594860307491,
-35.4618546294694));
#16043=CARTESIAN_POINT('Ctrl Pts',(-2.14011010082685,-3.30179318329602,
-35.4559773794269));
#16044=CARTESIAN_POINT('Ctrl Pts',(-2.04175978384362,-3.36350833667166,
-35.4501001293844));
#16045=CARTESIAN_POINT('Ctrl Pts',(-1.9407677419334,-3.42080539812933,-35.4442228793419));
#16046=CARTESIAN_POINT('Ctrl Pts',(-1.83987557247139,-3.47804579771845,
-35.4383514413945));
#16047=CARTESIAN_POINT('Ctrl Pts',(-1.73634723084554,-3.53087659515673,
-35.4324800034471));
#16048=CARTESIAN_POINT('Ctrl Pts',(-1.6306053706547,-3.5790522663398,-35.4266085654997));
#16049=CARTESIAN_POINT('Ctrl Pts',(-1.52353649576712,-3.62783252139882,
-35.4206634435408));
#16050=CARTESIAN_POINT('Ctrl Pts',(-1.4141985138439,-3.67183976181265,-35.4147183215818));
#16051=CARTESIAN_POINT('Ctrl Pts',(-1.30305645053974,-3.71086686458929,
-35.4087731996229));
#16052=CARTESIAN_POINT('Ctrl Pts',(-1.19341053362311,-3.74936860138749,
-35.4029081083245));
#16053=CARTESIAN_POINT('Ctrl Pts',(-1.08200921092332,-3.78302332655099,
-35.3970430170261));
#16054=CARTESIAN_POINT('Ctrl Pts',(-0.96931860959011,-3.81168078845833,
-35.3911779257277));
#16055=CARTESIAN_POINT('Ctrl Pts',(-0.856643069582972,-3.8403344202381,
-35.3853136183106));
#16056=CARTESIAN_POINT('Ctrl Pts',(-0.742678992132058,-3.86399201575787,
-35.3794493108935));
#16057=CARTESIAN_POINT('Ctrl Pts',(-0.627905965179305,-3.88255368268003,
-35.3735850034764));
#16058=CARTESIAN_POINT('Ctrl Pts',(-0.513120833305429,-3.90111730727047,
-35.3677200775605));
#16059=CARTESIAN_POINT('Ctrl Pts',(-0.397526988314185,-3.9145838691709,
-35.3618551516446));
#16060=CARTESIAN_POINT('Ctrl Pts',(-0.281611788061173,-3.92290502062247,
-35.3559902257287));
#16061=CARTESIAN_POINT('Ctrl Pts',(-0.162920589154323,-3.93142545141944,
-35.3499848434584));
#16062=CARTESIAN_POINT('Ctrl Pts',(-0.0438928990445518,-3.93455084456753,
-35.3439794611881));
#16063=CARTESIAN_POINT('Ctrl Pts',(0.0749465089043309,-3.93228585186823,
-35.3379740789177));
#16064=CARTESIAN_POINT('Ctrl Pts',(0.191176106553475,-3.93007060025548,
-35.3321005797389));
#16065=CARTESIAN_POINT('Ctrl Pts',(0.307225195050442,-3.92269936432258,
-35.32622708056));
#16066=CARTESIAN_POINT('Ctrl Pts',(0.422607673289962,-3.91022911790044,
-35.3203535813811));
#16067=CARTESIAN_POINT('Ctrl Pts',(0.541876335249591,-3.89733886257079,
-35.3142822575651));
#16068=CARTESIAN_POINT('Ctrl Pts',(0.660432211828677,-3.87900013685128,
-35.308210933749));
#16069=CARTESIAN_POINT('Ctrl Pts',(0.77775073672986,-3.85533303250396,-35.302139609933));
#16070=CARTESIAN_POINT('Ctrl Pts',(0.895069261631039,-3.83166592815663,
-35.296068286117));
#16071=CARTESIAN_POINT('Ctrl Pts',(1.01114998620073,-3.80267062373241,-35.289996962301));
#16072=CARTESIAN_POINT('Ctrl Pts',(1.12548770706434,-3.76852310875853,-35.283925638485));
#16073=CARTESIAN_POINT('Ctrl Pts',(1.23630940586834,-3.73542567082854,-35.2780410151586));
#16074=CARTESIAN_POINT('Ctrl Pts',(1.345846078771,-3.69738306041137,-35.2721563918322));
#16075=CARTESIAN_POINT('Ctrl Pts',(1.4536250113728,-3.65451273445742,-35.2662717685058));
#16076=CARTESIAN_POINT('Ctrl Pts',(1.56126889860917,-3.61169612437071,-35.2603945185231));
#16077=CARTESIAN_POINT('Ctrl Pts',(1.66715904704408,-3.56406398053053,-35.2545172685403));
#16078=CARTESIAN_POINT('Ctrl Pts',(1.77083703148471,-3.5117837644027,-35.2486400185576));
#16079=CARTESIAN_POINT('Ctrl Pts',(1.87441248724979,-3.45955524894543,-35.2427685806733));
#16080=CARTESIAN_POINT('Ctrl Pts',(1.9757797657369,-3.40268798941228,-35.236897142789));
#16081=CARTESIAN_POINT('Ctrl Pts',(2.07450019996574,-3.34139759985879,-35.2310257049048));
#16082=CARTESIAN_POINT('Ctrl Pts',(2.17445953447812,-3.27933804147426,-35.2250805829234));
#16083=CARTESIAN_POINT('Ctrl Pts',(2.27170473558523,-3.21274372887598,-35.2191354609421));
#16084=CARTESIAN_POINT('Ctrl Pts',(2.36580560185385,-3.14188683027205,-35.2131903389607));
#16085=CARTESIAN_POINT('Ctrl Pts',(2.45863972148375,-3.07198377770266,-35.2073252477335));
#16086=CARTESIAN_POINT('Ctrl Pts',(2.5484133093192,-2.99793245860549,-35.2014601565062));
#16087=CARTESIAN_POINT('Ctrl Pts',(2.63474288294348,-2.9200374896187,-35.1955950652789));
#16088=CARTESIAN_POINT('Ctrl Pts',(2.72106091840379,-2.84215293148982,-35.1897307579358));
#16089=CARTESIAN_POINT('Ctrl Pts',(2.8039355498467,-2.76042602060623,-35.1838664505927));
#16090=CARTESIAN_POINT('Ctrl Pts',(2.88301774185246,-2.67520049718968,-35.1780021432496));
#16091=CARTESIAN_POINT('Ctrl Pts',(2.96210827448838,-2.58996598521892,-35.1721372174105));
#16092=CARTESIAN_POINT('Ctrl Pts',(3.03740529281105,-2.50123242865741,-35.1662722915714));
#16093=CARTESIAN_POINT('Ctrl Pts',(3.108598350078,-2.40937861240037,-35.1604073657323));
#16094=CARTESIAN_POINT('Ctrl Pts',(3.18149637851831,-2.31532502955241,-35.1544019833673));
#16095=CARTESIAN_POINT('Ctrl Pts',(3.25009109191741,-2.21800018708156,-35.1483966010023));
#16096=CARTESIAN_POINT('Ctrl Pts',(3.31409540635905,-2.11784339306518,-35.1423912186373));
#16097=CARTESIAN_POINT('Ctrl Pts',(3.37669413199414,-2.01988612684309,-35.1365177195416));
#16098=CARTESIAN_POINT('Ctrl Pts',(3.43490184314894,-1.91922040189029,-35.1306442204458));
#16099=CARTESIAN_POINT('Ctrl Pts',(3.48849644101194,-1.81628235168628,-35.12477072135));
#16100=CARTESIAN_POINT('Ctrl Pts',(3.54389615469999,-1.70987725236104,-35.1186993973504));
#16101=CARTESIAN_POINT('Ctrl Pts',(3.59436632447562,-1.60104450114051,-35.1126280733509));
#16102=CARTESIAN_POINT('Ctrl Pts',(3.63971605311705,-1.49028723831416,-35.1065567493513));
#16103=CARTESIAN_POINT('Ctrl Pts',(3.68506578175848,-1.37952997548781,-35.1004854253517));
#16104=CARTESIAN_POINT('Ctrl Pts',(3.72529496910861,-1.26684867343169,-35.0944141013522));
#16105=CARTESIAN_POINT('Ctrl Pts',(3.76026997298341,-1.15276135009782,-35.0883427773526));
#16106=CARTESIAN_POINT('Ctrl Pts',(3.80113461351723,-1.01946222383631,-35.0812490691233));
#16107=CARTESIAN_POINT('Ctrl Pts',(3.83493313330237,-0.88390402157618,-35.074155360894));
#16108=CARTESIAN_POINT('Ctrl Pts',(3.86145381695015,-0.746768651967352,
-35.0670616526647));
#16109=CARTESIAN_POINT('Ctrl Pts',(3.8876819604404,-0.611145973477642,-35.0600461925888));
#16110=CARTESIAN_POINT('Ctrl Pts',(3.9067919115526,-0.473980755150574,-35.0530307325129));
#16111=CARTESIAN_POINT('Ctrl Pts',(3.91862537579101,-0.33595262196737,-35.046015272437));
#16112=CARTESIAN_POINT('Ctrl Pts',(3.92810036406333,-0.225434271904183,
-35.0403980330044));
#16113=CARTESIAN_POINT('Ctrl Pts',(3.93291115998635,-0.114363079279912,
-35.0347807935718));
#16114=CARTESIAN_POINT('Ctrl Pts',(3.93299878050155,-0.00309718796439099,
-35.0291635541393));
#16115=CARTESIAN_POINT('',(3.93264515487443,0.00306832688220754,-33.7791634933578));
#16116=CARTESIAN_POINT('Ctrl Pts',(3.93057853514731,-0.0030946465227831,
-35.029163522035));
#16117=CARTESIAN_POINT('Ctrl Pts',(3.92365169001617,0.896981560524963,-34.9836956534301));
#16118=CARTESIAN_POINT('Ctrl Pts',(3.17394638211024,3.09807182351393,-34.8730334977809));
#16119=CARTESIAN_POINT('Ctrl Pts',(-0.452408180865259,4.60400171736557,
-34.697177055088));
#16120=CARTESIAN_POINT('Ctrl Pts',(-4.08239314255048,2.17613677140805,-34.5015941939554));
#16121=CARTESIAN_POINT('Ctrl Pts',(-4.07447403678864,-2.19092822357172,
-34.3060113328231));
#16122=CARTESIAN_POINT('Ctrl Pts',(-0.435707702205553,-4.60561216169713,
-34.1104284716908));
#16123=CARTESIAN_POINT('Ctrl Pts',(3.18020937176261,-3.08861798879681,-33.9348125347613));
#16124=CARTESIAN_POINT('Ctrl Pts',(3.92364775283068,-0.892318847406521,
-33.8243908848761));
#16125=CARTESIAN_POINT('Ctrl Pts',(3.93045809296359,0.00306605271246902,
-33.779163522035));
#16126=CARTESIAN_POINT('',(3.93299959220032,-0.00179101985566553,-32.5291635219964));
#16127=CARTESIAN_POINT('Ctrl Pts',(3.9329988028365,0.00306869461550739,
-33.7791634887208));
#16128=CARTESIAN_POINT('Ctrl Pts',(3.93289100539829,0.141227504320743,-33.7721893226934));
#16129=CARTESIAN_POINT('Ctrl Pts',(3.92549945843856,0.279086805530256,-33.7652151566661));
#16130=CARTESIAN_POINT('Ctrl Pts',(3.91094177047953,0.415960897102635,-33.7582409906387));
#16131=CARTESIAN_POINT('Ctrl Pts',(3.89621992300834,0.554378446960705,-33.7511881805508));
#16132=CARTESIAN_POINT('Ctrl Pts',(3.87416947544637,0.691788396585036,-33.744135370463));
#16133=CARTESIAN_POINT('Ctrl Pts',(3.84496154579419,0.827502091455922,-33.7370825603751));
#16134=CARTESIAN_POINT('Ctrl Pts',(3.82036237760766,0.941801326119291,-33.7311426233921));
#16135=CARTESIAN_POINT('Ctrl Pts',(3.79068718235984,1.0548977358952,-33.725202686409));
#16136=CARTESIAN_POINT('Ctrl Pts',(3.75606447311104,1.16639130390838,-33.719262749426));
#16137=CARTESIAN_POINT('Ctrl Pts',(3.72176417441482,1.2768466313086,-33.7133781258025));
#16138=CARTESIAN_POINT('Ctrl Pts',(3.68253296561105,1.38596324660863,-33.707493502179));
#16139=CARTESIAN_POINT('Ctrl Pts',(3.63849343586062,1.49326974026771,-33.7016088785555));
#16140=CARTESIAN_POINT('Ctrl Pts',(3.59450908705311,1.60044178032259,-33.6957316282869));
#16141=CARTESIAN_POINT('Ctrl Pts',(3.54572855487768,1.70580783244215,-33.6898543780182));
#16142=CARTESIAN_POINT('Ctrl Pts',(3.49232427470953,1.80891131907415,-33.6839771277496));
#16143=CARTESIAN_POINT('Ctrl Pts',(3.43897280691607,1.91191284496533,-33.6781056895908));
#16144=CARTESIAN_POINT('Ctrl Pts',(3.38100687546608,2.01265589327127,-33.672234251432));
#16145=CARTESIAN_POINT('Ctrl Pts',(3.31864685067646,2.11070416697727,-33.6663628132732));
#16146=CARTESIAN_POINT('Ctrl Pts',(3.25550423767038,2.20998289920066,-33.6604176913991));
#16147=CARTESIAN_POINT('Ctrl Pts',(3.18785664584906,2.30649835847185,-33.6544725695249));
#16148=CARTESIAN_POINT('Ctrl Pts',(3.11598090425347,2.39982332773222,-33.6485274476508));
#16149=CARTESIAN_POINT('Ctrl Pts',(3.04507271968931,2.49189200066491,-33.6426623561783));
#16150=CARTESIAN_POINT('Ctrl Pts',(2.97004978649661,2.58085522413837,-33.6367972647059));
#16151=CARTESIAN_POINT('Ctrl Pts',(2.89122087237093,2.6663328500333,-33.6309321732334));
#16152=CARTESIAN_POINT('Ctrl Pts',(2.81240249407926,2.7517990514644,-33.6250678656565));
#16153=CARTESIAN_POINT('Ctrl Pts',(2.72977942529371,2.8337802795901,-33.6192035580795));
#16154=CARTESIAN_POINT('Ctrl Pts',(2.64369918049048,2.91193125658453,-33.6133392505025));
#16155=CARTESIAN_POINT('Ctrl Pts',(2.55760985715705,2.99009047584183,-33.6074743244411));
#16156=CARTESIAN_POINT('Ctrl Pts',(2.46806293747283,3.06441836447313,-33.6016093983797));
#16157=CARTESIAN_POINT('Ctrl Pts',(2.37544055899965,3.13460861203746,-33.5957444723183));
#16158=CARTESIAN_POINT('Ctrl Pts',(2.28060001730402,3.20647980785954,-33.5897390903162));
#16159=CARTESIAN_POINT('Ctrl Pts',(2.18253519374144,3.27401237963774,-33.5837337083142));
#16160=CARTESIAN_POINT('Ctrl Pts',(2.08168849136363,3.33692403643299,-33.5777283263121));
#16161=CARTESIAN_POINT('Ctrl Pts',(1.98305645856488,3.39845410583679,-33.5718548270243));
#16162=CARTESIAN_POINT('Ctrl Pts',(1.88176386432633,3.45556397466868,-33.5659813277365));
#16163=CARTESIAN_POINT('Ctrl Pts',(1.77824923092822,3.50803629865815,-33.5601078284487));
#16164=CARTESIAN_POINT('Ctrl Pts',(1.67124814333661,3.56227593175176,-33.5540365050895));
#16165=CARTESIAN_POINT('Ctrl Pts',(1.56187313987604,3.6115599207793,-33.5479651817303));
#16166=CARTESIAN_POINT('Ctrl Pts',(1.45062940626627,3.65570284975072,-33.5418938583712));
#16167=CARTESIAN_POINT('Ctrl Pts',(1.33938567265651,3.69984577872215,-33.535822535012));
#16168=CARTESIAN_POINT('Ctrl Pts',(1.22627368233417,3.73884755262167,-33.5297512116529));
#16169=CARTESIAN_POINT('Ctrl Pts',(1.11181287535345,3.77258016882323,-33.5236798882937));
#16170=CARTESIAN_POINT('Ctrl Pts',(1.00087175247158,3.80527550286691,-33.5177952588855));
#16171=CARTESIAN_POINT('Ctrl Pts',(0.888310844573323,3.83312496977567,-33.5119106294773));
#16172=CARTESIAN_POINT('Ctrl Pts',(0.774590439266641,3.85596922334667,-33.5060260000691));
#16173=CARTESIAN_POINT('Ctrl Pts',(0.661012523218186,3.87878485355199,-33.5001487439768));
#16174=CARTESIAN_POINT('Ctrl Pts',(0.546278399129095,3.89660766344188,-33.4942714878846));
#16175=CARTESIAN_POINT('Ctrl Pts',(0.4308636477164,3.90932801349241,-33.4883942317924));
#16176=CARTESIAN_POINT('Ctrl Pts',(0.315563031132705,3.92203578425857,-33.4825227877788));
#16177=CARTESIAN_POINT('Ctrl Pts',(0.199583532768558,3.92965108828396,-33.4766513437653));
#16178=CARTESIAN_POINT('Ctrl Pts',(0.0834104323618352,3.9321154229973,-33.4707798997518));
#16179=CARTESIAN_POINT('Ctrl Pts',(-0.0342204239031183,3.93461068051766,
-33.4648347800605));
#16180=CARTESIAN_POINT('Ctrl Pts',(-0.152049354966056,3.93182472315353,
-33.4588896603692));
#16181=CARTESIAN_POINT('Ctrl Pts',(-0.269567336800497,3.92375106893012,
-33.4529445406779));
#16182=CARTESIAN_POINT('Ctrl Pts',(-0.385503506534395,3.91578608747106,
-33.4470794433128));
#16183=CARTESIAN_POINT('Ctrl Pts',(-0.501136624927632,3.90267491989501,
-33.4412143459476));
#16184=CARTESIAN_POINT('Ctrl Pts',(-0.615979129770265,3.88446376114998,
-33.4353492485825));
#16185=CARTESIAN_POINT('Ctrl Pts',(-0.730806285486452,3.86625503639382,
-33.4294849351093));
#16186=CARTESIAN_POINT('Ctrl Pts',(-0.844842631716971,3.84294774051984,
-33.4236206216362));
#16187=CARTESIAN_POINT('Ctrl Pts',(-0.957608143411652,3.8146396479447,-33.417756308163));
#16188=CARTESIAN_POINT('Ctrl Pts',(-1.07038554794669,3.78632856985014,-33.4118913762087));
#16189=CARTESIAN_POINT('Ctrl Pts',(-1.18189145261582,3.75301574673305,-33.4060264442544));
#16190=CARTESIAN_POINT('Ctrl Pts',(-1.29165906555342,3.71484937223216,-33.4001615123001));
#16191=CARTESIAN_POINT('Ctrl Pts',(-1.40405517649577,3.67576906477291,-33.3941561385385));
#16192=CARTESIAN_POINT('Ctrl Pts',(-1.5146282547568,3.63159994266073,-33.388150764777));
#16193=CARTESIAN_POINT('Ctrl Pts',(-1.62289808782706,3.58255366973438,-33.3821453910154));
#16194=CARTESIAN_POINT('Ctrl Pts',(-1.72879048418896,3.53458437648332,-33.3762718858974));
#16195=CARTESIAN_POINT('Ctrl Pts',(-1.83247940080365,3.4819501569843,-33.3703983807794));
#16196=CARTESIAN_POINT('Ctrl Pts',(-1.93354082357389,3.4248954558604,-33.3645248756614));
#16197=CARTESIAN_POINT('Ctrl Pts',(-2.0380057079412,3.36591931449862,-33.3584535675781));
#16198=CARTESIAN_POINT('Ctrl Pts',(-2.13966259455587,3.30221996183034,-33.3523822594947));
#16199=CARTESIAN_POINT('Ctrl Pts',(-2.23807708431421,3.23411502032127,-33.3463109514113));
#16200=CARTESIAN_POINT('Ctrl Pts',(-2.33649157407254,3.16601007881219,-33.340239643328));
#16201=CARTESIAN_POINT('Ctrl Pts',(-2.43166332541418,3.09349988977969,-33.3341683352446));
#16202=CARTESIAN_POINT('Ctrl Pts',(-2.52319781621016,3.01694577019082,-33.3280970271613));
#16203=CARTESIAN_POINT('Ctrl Pts',(-2.61191753789585,2.94274575962916,-33.3222124173411));
#16204=CARTESIAN_POINT('Ctrl Pts',(-2.69750251298505,2.86451100509295,-33.3163278075209));
#16205=CARTESIAN_POINT('Ctrl Pts',(-2.77956492914437,2.78253621803395,-33.3104431977007));
#16206=CARTESIAN_POINT('Ctrl Pts',(-2.86152452215785,2.70066414432266,-33.3045659612205));
#16207=CARTESIAN_POINT('Ctrl Pts',(-2.93997004623968,2.61506164677989,-33.2986887247403));
#16208=CARTESIAN_POINT('Ctrl Pts',(-3.01454657687363,2.52606372363396,-33.2928114882601));
#16209=CARTESIAN_POINT('Ctrl Pts',(-3.08904935777308,2.43715381173162,-33.2869400638581));
#16210=CARTESIAN_POINT('Ctrl Pts',(-3.15969049388662,2.34485546747271,-33.2810686394561));
#16211=CARTESIAN_POINT('Ctrl Pts',(-3.22615224045201,2.24954011331794,-33.2751972150541));
#16212=CARTESIAN_POINT('Ctrl Pts',(-3.29344826604316,2.15302828743447,-33.2692520880114));
#16213=CARTESIAN_POINT('Ctrl Pts',(-3.35645894996537,2.05342348798032,-33.2633069609687));
#16214=CARTESIAN_POINT('Ctrl Pts',(-3.41489667157031,1.9511457460933,-33.257361833926));
#16215=CARTESIAN_POINT('Ctrl Pts',(-3.4725475486578,1.85024514003999,-33.2514967560448));
#16216=CARTESIAN_POINT('Ctrl Pts',(-3.525747651882,1.74674350200199,-33.2456316781637));
#16217=CARTESIAN_POINT('Ctrl Pts',(-3.57426510284596,1.64107220273135,-33.2397666002825));
#16218=CARTESIAN_POINT('Ctrl Pts',(-3.62277606993461,1.53541502538006,-33.2339023062108));
#16219=CARTESIAN_POINT('Ctrl Pts',(-3.6666054577924,1.42758913713199,-33.2280380121391));
#16220=CARTESIAN_POINT('Ctrl Pts',(-3.70556849258319,1.31804823385746,-33.2221737180673));
#16221=CARTESIAN_POINT('Ctrl Pts',(-3.74453563732704,1.20849577583688,-33.2163088054099));
#16222=CARTESIAN_POINT('Ctrl Pts',(-3.7786352707319,1.09722833064852,-33.2104438927526));
#16223=CARTESIAN_POINT('Ctrl Pts',(-3.80773191605457,0.984716535587463,
-33.2045789800952));
#16224=CARTESIAN_POINT('Ctrl Pts',(-3.83752554438897,0.869509625371121,
-33.198573578923));
#16225=CARTESIAN_POINT('Ctrl Pts',(-3.86207332821644,0.752998429117083,
-33.1925681777508));
#16226=CARTESIAN_POINT('Ctrl Pts',(-3.88128516945974,0.635699955428583,
-33.1865627765786));
#16227=CARTESIAN_POINT('Ctrl Pts',(-3.90007500252231,0.520978065361393,
-33.1806892903224));
#16228=CARTESIAN_POINT('Ctrl Pts',(-3.91376090692278,0.40550354843166,-33.1748158040662));
#16229=CARTESIAN_POINT('Ctrl Pts',(-3.92231122642181,0.289764806499083,
-33.1689423178099));
#16230=CARTESIAN_POINT('Ctrl Pts',(-3.93114959835571,0.17012693232627,-33.1628709591798));
#16231=CARTESIAN_POINT('Ctrl Pts',(-3.934500243471,0.0502072011357646,-33.1567996005496));
#16232=CARTESIAN_POINT('Ctrl Pts',(-3.93238664930414,-0.0694567518281636,
-33.1507282419194));
#16233=CARTESIAN_POINT('Ctrl Pts',(-3.93027305513729,-0.189120704792092,
-33.1446568832892));
#16234=CARTESIAN_POINT('Ctrl Pts',(-3.92269531637615,-0.308528406004927,
-33.1385855246591));
#16235=CARTESIAN_POINT('Ctrl Pts',(-3.9097353961647,-0.427151181640451,
-33.1325141660289));
#16236=CARTESIAN_POINT('Ctrl Pts',(-3.89717406651062,-0.542125638653213,
-33.1266295358801));
#16237=CARTESIAN_POINT('Ctrl Pts',(-3.87951686780026,-0.656728299452036,
-33.1207449057314));
#16238=CARTESIAN_POINT('Ctrl Pts',(-3.85679404856287,-0.770473015082302,
-33.1148602755826));
#16239=CARTESIAN_POINT('Ctrl Pts',(-3.83409970101184,-0.884075208614637,
-33.1089830188739));
#16240=CARTESIAN_POINT('Ctrl Pts',(-3.80635243691103,-0.996821195167531,
-33.1031057621651));
#16241=CARTESIAN_POINT('Ctrl Pts',(-3.77363426670775,-1.10822985933832,
-33.0972285054563));
#16242=CARTESIAN_POINT('Ctrl Pts',(-3.74094845251934,-1.21952834802034,
-33.0913570609493));
#16243=CARTESIAN_POINT('Ctrl Pts',(-3.70330162679568,-1.32949175279322,
-33.0854856164422));
#16244=CARTESIAN_POINT('Ctrl Pts',(-3.66082672701619,-1.43764970516601,
-33.0796141719352));
#16245=CARTESIAN_POINT('Ctrl Pts',(-3.61781885170795,-1.54716482476353,
-33.0736690524752));
#16246=CARTESIAN_POINT('Ctrl Pts',(-3.56986098538416,-1.6548284504036,-33.0677239330153));
#16247=CARTESIAN_POINT('Ctrl Pts',(-3.51714321807872,-1.76016833954109,
-33.0617788135554));
#16248=CARTESIAN_POINT('Ctrl Pts',(-3.46513503719965,-1.86409034322349,
-33.0559137159986));
#16249=CARTESIAN_POINT('Ctrl Pts',(-3.40849450365517,-1.9657504074155,-33.0500486184419));
#16250=CARTESIAN_POINT('Ctrl Pts',(-3.34745205280478,-2.06471638589252,
-33.0441835208851));
#16251=CARTESIAN_POINT('Ctrl Pts',(-3.28641776167668,-2.16366913529878,
-33.0383192073331));
#16252=CARTESIAN_POINT('Ctrl Pts',(-3.22098293935824,-2.25992816527032,
-33.032454893781));
#16253=CARTESIAN_POINT('Ctrl Pts',(-3.15142271737998,-2.35308815312588,
-33.0265905802289));
#16254=CARTESIAN_POINT('Ctrl Pts',(-3.0818551605482,-2.44625796433804,-33.0207256483079));
#16255=CARTESIAN_POINT('Ctrl Pts',(-3.00816158534893,-2.53632775427524,
-33.0148607163869));
#16256=CARTESIAN_POINT('Ctrl Pts',(-2.93065855470544,-2.62292383338362,
-33.0089957844659));
#16257=CARTESIAN_POINT('Ctrl Pts',(-2.85129964023448,-2.71159353801871,
-33.0029904111685));
#16258=CARTESIAN_POINT('Ctrl Pts',(-2.76794680303372,-2.79662070864973,
-32.996985037871));
#16259=CARTESIAN_POINT('Ctrl Pts',(-2.68098034811745,-2.87764371891449,
-32.9909796645736));
#16260=CARTESIAN_POINT('Ctrl Pts',(-2.59592353883439,-2.95688759217879,
-32.9851061597639));
#16261=CARTESIAN_POINT('Ctrl Pts',(-2.50741053123919,-3.03230111937766,
-32.9792326549541));
#16262=CARTESIAN_POINT('Ctrl Pts',(-2.41583023454058,-3.10358716292609,
-32.9733591501444));
#16263=CARTESIAN_POINT('Ctrl Pts',(-2.32116577711776,-3.17727391518177,
-32.9672878426031));
#16264=CARTESIAN_POINT('Ctrl Pts',(-2.22322418970466,-3.24654999930959,
-32.9612165350618));
#16265=CARTESIAN_POINT('Ctrl Pts',(-2.12246591290477,-3.3111368815797,-32.9551452275205));
#16266=CARTESIAN_POINT('Ctrl Pts',(-2.02170763610487,-3.37572376384981,
-32.9490739199792));
#16267=CARTESIAN_POINT('Ctrl Pts',(-1.91813311646427,-3.43562126052983,
-32.9430026124379));
#16268=CARTESIAN_POINT('Ctrl Pts',(-1.81222775722322,-3.49060446856267,
-32.9369313048966));
#16269=CARTESIAN_POINT('Ctrl Pts',(-1.70957815735091,-3.54389737408429,
-32.9310466424557));
#16270=CARTESIAN_POINT('Ctrl Pts',(-1.60441260888199,-3.59274317505789,
-32.9251619800147));
#16271=CARTESIAN_POINT('Ctrl Pts',(-1.49715247406656,-3.63689750603401,
-32.9192773175738));
#16272=CARTESIAN_POINT('Ctrl Pts',(-1.39002672970553,-3.68099651430692,
-32.9134000282586));
#16273=CARTESIAN_POINT('Ctrl Pts',(-1.28081199578994,-3.72041558845105,
-32.9075227389434));
#16274=CARTESIAN_POINT('Ctrl Pts',(-1.16995414392166,-3.7549562315852,-32.9016454496283));
#16275=CARTESIAN_POINT('Ctrl Pts',(-1.05920591713262,-3.78946271817855,
-32.8957739722452));
#16276=CARTESIAN_POINT('Ctrl Pts',(-0.946818195253127,-3.81910024897877,
-32.8899024948621));
#16277=CARTESIAN_POINT('Ctrl Pts',(-0.833256141587372,-3.84371866849109,
-32.884031017479));
#16278=CARTESIAN_POINT('Ctrl Pts',(-0.71826999020284,-3.86864580939349,
-32.8780859102409));
#16279=CARTESIAN_POINT('Ctrl Pts',(-0.602080246841668,-3.88842692692477,
-32.8721408030027));
#16280=CARTESIAN_POINT('Ctrl Pts',(-0.485185310360534,-3.9029583926312,
-32.8661956957646));
#16281=CARTESIAN_POINT('Ctrl Pts',(-0.369862899223941,-3.91729437426618,
-32.860330564889));
#16282=CARTESIAN_POINT('Ctrl Pts',(-0.253854572799971,-3.92652103580639,
-32.8544654340133));
#16283=CARTESIAN_POINT('Ctrl Pts',(-0.137647740870454,-3.9305905535216,
-32.8486003031376));
#16284=CARTESIAN_POINT('Ctrl Pts',(-0.021456440484935,-3.93465952732823,
-32.842735956162));
#16285=CARTESIAN_POINT('Ctrl Pts',(0.0949329017311209,-3.9335727137738,
-32.8368716091863));
#16286=CARTESIAN_POINT('Ctrl Pts',(0.211030418065854,-3.92733435839768,
-32.8310072622107));
#16287=CARTESIAN_POINT('Ctrl Pts',(0.327140177661687,-3.92109534514519,
-32.8251422968003));
#16288=CARTESIAN_POINT('Ctrl Pts',(0.442957639529098,-3.90970373216336,
-32.81927733139));
#16289=CARTESIAN_POINT('Ctrl Pts',(0.557996290726594,-3.89321578383929,
-32.8134123659797));
#16290=CARTESIAN_POINT('Ctrl Pts',(0.675788068279957,-3.87633324287516,
-32.8074070391284));
#16291=CARTESIAN_POINT('Ctrl Pts',(0.792762833562814,-3.85410738747903,
-32.8014017122771));
#16292=CARTESIAN_POINT('Ctrl Pts',(0.908408792051104,-3.8266542130854,-32.7953963854258));
#16293=CARTESIAN_POINT('Ctrl Pts',(1.02151686524768,-3.79980350684903,-32.7895228472759));
#16294=CARTESIAN_POINT('Ctrl Pts',(1.13335346959867,-3.76795272140445,-32.7836493091259));
#16295=CARTESIAN_POINT('Ctrl Pts',(1.24345568871581,-3.7312607722056,-32.777775770976));
#16296=CARTESIAN_POINT('Ctrl Pts',(1.35726356908134,-3.69333389844878,-32.771704549774));
#16297=CARTESIAN_POINT('Ctrl Pts',(1.46921780783199,-3.65023442009615,-32.7656333285721));
#16298=CARTESIAN_POINT('Ctrl Pts',(1.57883133942658,-3.60219108344414,-32.7595621073701));
#16299=CARTESIAN_POINT('Ctrl Pts',(1.68844487102117,-3.55414774679213,-32.7534908861681));
#16300=CARTESIAN_POINT('Ctrl Pts',(1.79571729501313,-3.50116082156502,-32.7474196649661));
#16301=CARTESIAN_POINT('Ctrl Pts',(1.90019233549209,-3.4435095597569,-32.7413484437642));
#16302=CARTESIAN_POINT('Ctrl Pts',(2.00145443157965,-3.38763126015519,-32.7354639321918));
#16303=CARTESIAN_POINT('Ctrl Pts',(2.10041065483412,-3.32719367701901,-32.7295794206194));
#16304=CARTESIAN_POINT('Ctrl Pts',(2.19662403138074,-3.26241197042321,-32.723694909047));
#16305=CARTESIAN_POINT('Ctrl Pts',(2.29271685043375,-3.19771143674181,-32.7178177708981));
#16306=CARTESIAN_POINT('Ctrl Pts',(2.38607332008407,-3.12867783359656,-32.7119406327492));
#16307=CARTESIAN_POINT('Ctrl Pts',(2.47628104895044,-3.05557215045054,-32.7060634946002));
#16308=CARTESIAN_POINT('Ctrl Pts',(2.56639956928246,-2.98253876322558,-32.7001921684908));
#16309=CARTESIAN_POINT('Ctrl Pts',(2.6533752255352,-2.90544156451583,-32.6943208423813));
#16310=CARTESIAN_POINT('Ctrl Pts',(2.73682515998634,-2.82458440193699,-32.6884495162718));
#16311=CARTESIAN_POINT('Ctrl Pts',(2.82132456074276,-2.74271037974974,-32.6825043523702));
#16312=CARTESIAN_POINT('Ctrl Pts',(2.90220859319854,-2.65698140870002,-32.6765591884685));
#16313=CARTESIAN_POINT('Ctrl Pts',(2.97911465530891,-2.56775483068841,-32.6706140245668));
#16314=CARTESIAN_POINT('Ctrl Pts',(3.05498347035287,-2.47973166894529,-32.6647490442508));
#16315=CARTESIAN_POINT('Ctrl Pts',(3.12698068875266,-2.38830499211795,-32.6588840639347));
#16316=CARTESIAN_POINT('Ctrl Pts',(3.1947962814962,-2.29385390113191,-32.6530190836187));
#16317=CARTESIAN_POINT('Ctrl Pts',(3.26260281637298,-2.19941542561322,-32.6471548866654));
#16318=CARTESIAN_POINT('Ctrl Pts',(3.3262285965868,-2.10195367335074,-32.6412906897121));
#16319=CARTESIAN_POINT('Ctrl Pts',(3.38540556353765,-2.00187866025099,-32.6354264927588));
#16320=CARTESIAN_POINT('Ctrl Pts',(3.4445887783888,-1.90179308123793,-32.629561676664));
#16321=CARTESIAN_POINT('Ctrl Pts',(3.49932203689145,-1.79909404692213,-32.6236968605692));
#16322=CARTESIAN_POINT('Ctrl Pts',(3.54938243186301,-1.69421762249783,-32.6178320444744));
#16323=CARTESIAN_POINT('Ctrl Pts',(3.60064399297771,-1.58682475747607,-32.6118265059875));
#16324=CARTESIAN_POINT('Ctrl Pts',(3.64700538402346,-1.47714908601084,-32.6058209675006));
#16325=CARTESIAN_POINT('Ctrl Pts',(3.68827935888879,-1.36568091836817,-32.5998154290138));
#16326=CARTESIAN_POINT('Ctrl Pts',(3.72864513663629,-1.25666550864162,-32.5939420370614));
#16327=CARTESIAN_POINT('Ctrl Pts',(3.76414500498145,-1.14593608744854,-32.588068645109));
#16328=CARTESIAN_POINT('Ctrl Pts',(3.79465457177639,-1.03396599600593,-32.5821952531567));
#16329=CARTESIAN_POINT('Ctrl Pts',(3.82619379917154,-0.918217050791476,
-32.5761236414025));
#16330=CARTESIAN_POINT('Ctrl Pts',(3.85239983575519,-0.801142687395448,
-32.5700520296484));
#16331=CARTESIAN_POINT('Ctrl Pts',(3.87319299810052,-0.683275200387892,
-32.5639804178942));
#16332=CARTESIAN_POINT('Ctrl Pts',(3.89398616044585,-0.565407713380327,
-32.5579088061401));
#16333=CARTESIAN_POINT('Ctrl Pts',(3.90936645103122,-0.446747585810446,
-32.5518371943859));
#16334=CARTESIAN_POINT('Ctrl Pts',(3.91931331057507,-0.327829488528789,
-32.5457655826318));
#16335=CARTESIAN_POINT('Ctrl Pts',(3.92837945707135,-0.219440616014741,
-32.5402315624328));
#16336=CARTESIAN_POINT('Ctrl Pts',(3.932950010281,-0.11067065348999,-32.5346975422339));
#16337=CARTESIAN_POINT('Ctrl Pts',(3.93299959219997,-0.00179102061575733,
-32.529163522035));
#16338=CARTESIAN_POINT('',(3.93299993544946,-0.00071256899522975,-31.2791635220851));
#16339=CARTESIAN_POINT('Ctrl Pts',(3.93299959220032,-0.00179101985566553,
-32.5291635219964));
#16340=CARTESIAN_POINT('Ctrl Pts',(3.93305171423223,0.112666633760392,-32.5233459879883));
#16341=CARTESIAN_POINT('Ctrl Pts',(3.92810321604783,0.227316899582816,-32.5175284539803));
#16342=CARTESIAN_POINT('Ctrl Pts',(3.9181299609264,0.341682029511204,-32.5117109199722));
#16343=CARTESIAN_POINT('Ctrl Pts',(3.90816838821679,0.455913195099014,-32.5059002004723));
#16344=CARTESIAN_POINT('Ctrl Pts',(3.89319379647479,0.56985947233263,-32.5000894809724));
#16345=CARTESIAN_POINT('Ctrl Pts',(3.87323406790185,0.683042352452951,-32.4942787614725));
#16346=CARTESIAN_POINT('Ctrl Pts',(3.85261041818044,0.799990038666822,-32.4882747598069));
#16347=CARTESIAN_POINT('Ctrl Pts',(3.82666418253833,0.916122200091492,-32.4822707581414));
#16348=CARTESIAN_POINT('Ctrl Pts',(3.79548448130774,1.03091539524448,-32.4762667564758));
#16349=CARTESIAN_POINT('Ctrl Pts',(3.76535245975493,1.14185138545445,-32.4704644972992));
#16350=CARTESIAN_POINT('Ctrl Pts',(3.73033314601399,1.25153650408435,-32.4646622381226));
#16351=CARTESIAN_POINT('Ctrl Pts',(3.69055888857356,1.35950876789032,-32.458859978946));
#16352=CARTESIAN_POINT('Ctrl Pts',(3.65079462690175,1.46745389691527,-32.4530591779497));
#16353=CARTESIAN_POINT('Ctrl Pts',(3.60627794228205,1.57368663149507,-32.4472583769534));
#16354=CARTESIAN_POINT('Ctrl Pts',(3.5571905223991,1.67776177908368,-32.4414575759572));
#16355=CARTESIAN_POINT('Ctrl Pts',(3.50810303093362,1.78183707844156,-32.4356567665018));
#16356=CARTESIAN_POINT('Ctrl Pts',(3.45444497145797,1.88375440369289,-32.4298559570464));
#16357=CARTESIAN_POINT('Ctrl Pts',(3.3964451407445,1.98309087182436,-32.424055147591));
#16358=CARTESIAN_POINT('Ctrl Pts',(3.33843056402285,2.08245259548421,-32.4182528633247));
#16359=CARTESIAN_POINT('Ctrl Pts',(3.2760722352333,2.1792317944758,-32.4124505790584));
#16360=CARTESIAN_POINT('Ctrl Pts',(3.20964319846377,2.27303311426721,-32.4066482947921));
#16361=CARTESIAN_POINT('Ctrl Pts',(3.14314496263893,2.36693214679135,-32.4008399662926));
#16362=CARTESIAN_POINT('Ctrl Pts',(3.07256780052672,2.45784676568021,-32.395031637793));
#16363=CARTESIAN_POINT('Ctrl Pts',(2.99822606403165,2.54541341808384,-32.3892233092935));
#16364=CARTESIAN_POINT('Ctrl Pts',(2.9238378888289,2.63303477034203,-32.3834113525324));
#16365=CARTESIAN_POINT('Ctrl Pts',(2.84568074474241,2.71730368548287,-32.3775993957713));
#16366=CARTESIAN_POINT('Ctrl Pts',(2.76410571389922,2.79789360097729,-32.3717874390101));
#16367=CARTESIAN_POINT('Ctrl Pts',(2.68241606262938,2.87859675272063,-32.3659673159148));
#16368=CARTESIAN_POINT('Ctrl Pts',(2.59729925430606,2.95561030985458,-32.3601471928195));
#16369=CARTESIAN_POINT('Ctrl Pts',(2.50913919232883,3.02864813299918,-32.3543270697242));
#16370=CARTESIAN_POINT('Ctrl Pts',(2.48821374737605,3.04598420234176,-32.3529456203159));
#16371=CARTESIAN_POINT('Ctrl Pts',(2.46711697543488,3.06309647867762,-32.3515641709077));
#16372=CARTESIAN_POINT('Ctrl Pts',(2.44585423534079,3.07998150310444,-32.3501827214994));
#16373=CARTESIAN_POINT('Ctrl Pts',(2.35527673756693,3.15191029759021,-32.3442978623446));
#16374=CARTESIAN_POINT('Ctrl Pts',(2.26137970117448,3.21995436481127,-32.3384130031897));
#16375=CARTESIAN_POINT('Ctrl Pts',(2.16453006659768,3.28379332339821,-32.3325281440348));
#16376=CARTESIAN_POINT('Ctrl Pts',(2.06780174887448,3.34755231532728,-32.3266506564369));
#16377=CARTESIAN_POINT('Ctrl Pts',(1.96812852948163,3.40711645073853,-32.320773168839));
#16378=CARTESIAN_POINT('Ctrl Pts',(1.86591016926874,3.46220569005071,-32.314895681241));
#16379=CARTESIAN_POINT('Ctrl Pts',(1.76379286466078,3.51724046677523,-32.3090240042731));
#16380=CARTESIAN_POINT('Ctrl Pts',(1.65913578480731,3.56780895416281,-32.3031523273051));
#16381=CARTESIAN_POINT('Ctrl Pts',(1.55236686215112,3.61367487819465,-32.2972806503371));
#16382=CARTESIAN_POINT('Ctrl Pts',(1.44426405557712,3.66011381370697,-32.2913356174217));
#16383=CARTESIAN_POINT('Ctrl Pts',(1.33399663377892,3.70173164382356,-32.2853905845063));
#16384=CARTESIAN_POINT('Ctrl Pts',(1.22203397624083,3.73833144075175,-32.2794455515908));
#16385=CARTESIAN_POINT('Ctrl Pts',(1.11157231774895,3.7744405717607,-32.2735802192554));
#16386=CARTESIAN_POINT('Ctrl Pts',(0.999461004124491,3.80566527020334,-32.2677148869199));
#16387=CARTESIAN_POINT('Ctrl Pts',(0.886169354619096,3.83186545626722,-32.2618495545844));
#16388=CARTESIAN_POINT('Ctrl Pts',(0.772892840062088,3.85806214217494,-32.255985005815));
#16389=CARTESIAN_POINT('Ctrl Pts',(0.658436703789539,3.8792355580563,-32.2501204570457));
#16390=CARTESIAN_POINT('Ctrl Pts',(0.543282626586267,3.89529626442579,-32.2442559082764));
#16391=CARTESIAN_POINT('Ctrl Pts',(0.428116404063426,3.91135866472064,-32.2383907409721));
#16392=CARTESIAN_POINT('Ctrl Pts',(0.312252501559839,3.92230722672671,-32.2325255736678));
#16393=CARTESIAN_POINT('Ctrl Pts',(0.196179246584895,3.92810421236624,-32.2266604063636));
#16394=CARTESIAN_POINT('Ctrl Pts',(0.0773377641063493,3.93403945013877,
-32.2206553608639));
#16395=CARTESIAN_POINT('Ctrl Pts',(-0.0417227306380141,3.93457424637719,
-32.2146503153641));
#16396=CARTESIAN_POINT('Ctrl Pts',(-0.160477806242441,3.92972465622003,
-32.2086452698644));
#16397=CARTESIAN_POINT('Ctrl Pts',(-0.276636168396961,3.92498110781244,
-32.2027715314465));
#16398=CARTESIAN_POINT('Ctrl Pts',(-0.392501921659066,3.91508632444816,
-32.1968977930285));
#16399=CARTESIAN_POINT('Ctrl Pts',(-0.507590284058821,3.90010783229504,
-32.1910240546105));
#16400=CARTESIAN_POINT('Ctrl Pts',(-0.626537836959727,3.8846270751567,-32.1849533555699));
#16401=CARTESIAN_POINT('Ctrl Pts',(-0.744654470882471,3.86371577033904,
-32.1788826565293));
#16402=CARTESIAN_POINT('Ctrl Pts',(-0.861418538167016,3.83750532274578,
-32.1728119574888));
#16403=CARTESIAN_POINT('Ctrl Pts',(-0.978182605451561,3.81129487515252,
-32.1667412584482));
#16404=CARTESIAN_POINT('Ctrl Pts',(-1.09359366177943,3.77978547286386,-32.1606705594076));
#16405=CARTESIAN_POINT('Ctrl Pts',(-1.20715061798569,3.74316395386266,-32.1545998603671));
#16406=CARTESIAN_POINT('Ctrl Pts',(-1.31721038200262,3.70767026088368,-32.1487161195013));
#16407=CARTESIAN_POINT('Ctrl Pts',(-1.42587865616431,3.66726183895507,-32.1428323786355));
#16408=CARTESIAN_POINT('Ctrl Pts',(-1.53268548963072,3.62206628733869,-32.1369486377698));
#16409=CARTESIAN_POINT('Ctrl Pts',(-1.63935845199653,3.57692738357938,-32.1310722715526));
#16410=CARTESIAN_POINT('Ctrl Pts',(-1.74417423832575,3.52701344283815,-32.1251959053355));
#16411=CARTESIAN_POINT('Ctrl Pts',(-1.84667826186071,3.47250174905227,-32.1193195391183));
#16412=CARTESIAN_POINT('Ctrl Pts',(-1.9490808989236,3.41804397264572,-32.1134489852002));
#16413=CARTESIAN_POINT('Ctrl Pts',(-2.04917596062447,3.35899768197562,-32.1075784312821));
#16414=CARTESIAN_POINT('Ctrl Pts',(-2.14652965376657,3.29558787555434,-32.101707877364));
#16415=CARTESIAN_POINT('Ctrl Pts',(-2.24512543193172,3.23136905646669,-32.0957624241086));
#16416=CARTESIAN_POINT('Ctrl Pts',(-2.34090900591231,3.16267476497765,-32.0898169708532));
#16417=CARTESIAN_POINT('Ctrl Pts',(-2.43345601439873,3.08978653404837,-32.0838715175978));
#16418=CARTESIAN_POINT('Ctrl Pts',(-2.52473842753528,3.01789427391708,-32.0780073051374));
#16419=CARTESIAN_POINT('Ctrl Pts',(-2.61287184749229,2.9419222435584,-32.0721430926769));
#16420=CARTESIAN_POINT('Ctrl Pts',(-2.69747958601758,2.8621832371493,-32.0662788802165));
#16421=CARTESIAN_POINT('Ctrl Pts',(-2.78207606554118,2.78245484184532,-32.0604154481241));
#16422=CARTESIAN_POINT('Ctrl Pts',(-2.86314749740785,2.69896074954711,-32.0545520160318));
#16423=CARTESIAN_POINT('Ctrl Pts',(-2.9403524823033,2.61205212042426,-32.0486885839394));
#16424=CARTESIAN_POINT('Ctrl Pts',(-3.01756567032978,2.52513425714542,-32.0428245288497));
#16425=CARTESIAN_POINT('Ctrl Pts',(-3.09091132148113,2.43480144339318,-32.03696047376));
#16426=CARTESIAN_POINT('Ctrl Pts',(-3.16008737867501,2.34143903596462,-32.0310964186702));
#16427=CARTESIAN_POINT('Ctrl Pts',(-3.23094520039683,2.2458068607663,-32.0250898003839));
#16428=CARTESIAN_POINT('Ctrl Pts',(-3.29742779643953,2.14699624324494,-32.0190831820976));
#16429=CARTESIAN_POINT('Ctrl Pts',(-3.35925750524257,2.04545300935305,-32.0130765638113));
#16430=CARTESIAN_POINT('Ctrl Pts',(-3.41970817227618,1.94617458251997,-32.0072039163567));
#16431=CARTESIAN_POINT('Ctrl Pts',(-3.47571118555646,1.84428455241217,-32.0013312689021));
#16432=CARTESIAN_POINT('Ctrl Pts',(-3.52705408247575,1.74022369231405,-31.9954586214474));
#16433=CARTESIAN_POINT('Ctrl Pts',(-3.58015388307097,1.63260197144264,-31.9893850177453));
#16434=CARTESIAN_POINT('Ctrl Pts',(-3.6282687334104,1.52265863931259,-31.9833114140432));
#16435=CARTESIAN_POINT('Ctrl Pts',(-3.6712185706291,1.41090155810674,-31.9772378103411));
#16436=CARTESIAN_POINT('Ctrl Pts',(-3.7141684078478,1.29914447690088,-31.9711642066389));
#16437=CARTESIAN_POINT('Ctrl Pts',(-3.75195314199437,1.18557412248454,-31.9650906029368));
#16438=CARTESIAN_POINT('Ctrl Pts',(-3.78445039868035,1.07071199672375,-31.9590169992347));
#16439=CARTESIAN_POINT('Ctrl Pts',(-3.81594193452872,0.959404608965796,
-31.9531313606233));
#16440=CARTESIAN_POINT('Ctrl Pts',(-3.84256869735034,0.846530012854143,
-31.9472457220119));
#16441=CARTESIAN_POINT('Ctrl Pts',(-3.86417636695459,0.732550343027453,
-31.9413600834006));
#16442=CARTESIAN_POINT('Ctrl Pts',(-3.88575695202142,0.61871354314872,-31.935481822253));
#16443=CARTESIAN_POINT('Ctrl Pts',(-3.90233088084884,0.503774825099512,
-31.9296035611053));
#16444=CARTESIAN_POINT('Ctrl Pts',(-3.91379370506384,0.388211069139834,
-31.9237252999577));
#16445=CARTESIAN_POINT('Ctrl Pts',(-3.9252451851199,0.27276168059867,-31.9178528562184));
#16446=CARTESIAN_POINT('Ctrl Pts',(-3.93159558268809,0.156688891572664,
-31.9119804124791));
#16447=CARTESIAN_POINT('Ctrl Pts',(-3.9327916895247,0.0404787204031693,
-31.9061079687398));
#16448=CARTESIAN_POINT('Ctrl Pts',(-3.93400252235544,-0.0771621844156868,
-31.9001632257965));
#16449=CARTESIAN_POINT('Ctrl Pts',(-3.9299312103716,-0.194943457129721,
-31.8942184828533));
#16450=CARTESIAN_POINT('Ctrl Pts',(-3.92057681599806,-0.312356254713251,
-31.8882737399101));
#16451=CARTESIAN_POINT('Ctrl Pts',(-3.91134620590901,-0.42821535907428,
-31.8824076622147));
#16452=CARTESIAN_POINT('Ctrl Pts',(-3.89697153222601,-0.54371526059975,
-31.8765415845193));
#16453=CARTESIAN_POINT('Ctrl Pts',(-3.87750429054874,-0.658368799971655,
-31.8706755068239));
#16454=CARTESIAN_POINT('Ctrl Pts',(-3.85803968014414,-0.773006842298287,
-31.8648102220117));
#16455=CARTESIAN_POINT('Ctrl Pts',(-3.8334839395444,-0.886798344779898,
-31.8589449371996));
#16456=CARTESIAN_POINT('Ctrl Pts',(-3.80394005912343,-0.999264242628561,
-31.8530796523875));
#16457=CARTESIAN_POINT('Ctrl Pts',(-3.77439311406386,-1.11174180676233,
-31.847213759159));
#16458=CARTESIAN_POINT('Ctrl Pts',(-3.73985710503007,-1.2228930952866,-31.8413478659306));
#16459=CARTESIAN_POINT('Ctrl Pts',(-3.70048529600371,-1.33225281912268,
-31.8354819727021));
#16460=CARTESIAN_POINT('Ctrl Pts',(-3.66018660840177,-1.44418705471125,
-31.8294779864855));
#16461=CARTESIAN_POINT('Ctrl Pts',(-3.61482172994897,-1.55424388785106,
-31.8234740002688));
#16462=CARTESIAN_POINT('Ctrl Pts',(-3.56460727454468,-1.66194584095365,
-31.8174700140522));
#16463=CARTESIAN_POINT('Ctrl Pts',(-3.51547634177199,-1.76732381179428,
-31.8115955812658));
#16464=CARTESIAN_POINT('Ctrl Pts',(-3.46170324796393,-1.87044716029178,
-31.8057211484794));
#16465=CARTESIAN_POINT('Ctrl Pts',(-3.40353702545444,-1.97089439503002,
-31.799846715693));
#16466=CARTESIAN_POINT('Ctrl Pts',(-3.34344662560106,-2.07466449113008,
-31.7937779527612));
#16467=CARTESIAN_POINT('Ctrl Pts',(-3.27866766660018,-2.17557794348095,
-31.7877091898294));
#16468=CARTESIAN_POINT('Ctrl Pts',(-3.20952190686546,-2.273204374743,-31.7816404268976));
#16469=CARTESIAN_POINT('Ctrl Pts',(-3.14037614713074,-2.37083080600505,
-31.7755716639658));
#16470=CARTESIAN_POINT('Ctrl Pts',(-3.06686393037735,-2.46516987925628,
-31.7695029010341));
#16471=CARTESIAN_POINT('Ctrl Pts',(-2.98935019207031,-2.55583145554812,
-31.7634341381023));
#16472=CARTESIAN_POINT('Ctrl Pts',(-2.91417255045495,-2.64376068770246,
-31.7575482745806));
#16473=CARTESIAN_POINT('Ctrl Pts',(-2.83499306814641,-2.72850939594701,
-31.7516624110588));
#16474=CARTESIAN_POINT('Ctrl Pts',(-2.75211092009533,-2.80969295181734,
-31.7457765475371));
#16475=CARTESIAN_POINT('Ctrl Pts',(-2.66933239946434,-2.89077500401473,
-31.7398980431014));
#16476=CARTESIAN_POINT('Ctrl Pts',(-2.58286071195722,-2.96830048431027,
-31.7340195386656));
#16477=CARTESIAN_POINT('Ctrl Pts',(-2.49303494529769,-3.04191810565711,
-31.7281410342298));
#16478=CARTESIAN_POINT('Ctrl Pts',(-2.40329779861645,-3.11546309759874,
-31.7222683293876));
#16479=CARTESIAN_POINT('Ctrl Pts',(-2.3102134718646,-3.18510764119335,-31.7163956245454));
#16480=CARTESIAN_POINT('Ctrl Pts',(-2.21415705663655,-3.25053803677892,
-31.7105229197031));
#16481=CARTESIAN_POINT('Ctrl Pts',(-2.11692384721111,-3.31677002494606,
-31.7045782679226));
#16482=CARTESIAN_POINT('Ctrl Pts',(-2.01664554141955,-3.37868361472674,
-31.698633616142));
#16483=CARTESIAN_POINT('Ctrl Pts',(-1.91374511930567,-3.43599601547116,
-31.6926889643615));
#16484=CARTESIAN_POINT('Ctrl Pts',(-1.81219955576724,-3.4925538012584,-31.6868225840037));
#16485=CARTESIAN_POINT('Ctrl Pts',(-1.70810088469865,-3.54463063851432,
-31.6809562036459));
#16486=CARTESIAN_POINT('Ctrl Pts',(-1.60188317654743,-3.59199934419458,
-31.6750898232882));
#16487=CARTESIAN_POINT('Ctrl Pts',(-1.49567955441164,-3.63936176809443,
-31.6692242208979));
#16488=CARTESIAN_POINT('Ctrl Pts',(-1.38735782941932,-3.68201713481731,
-31.6633586185076));
#16489=CARTESIAN_POINT('Ctrl Pts',(-1.27737387499542,-3.71978560988119,
-31.6574930161173));
#16490=CARTESIAN_POINT('Ctrl Pts',(-1.16737824096497,-3.75755809572038,
-31.6516267908368));
#16491=CARTESIAN_POINT('Ctrl Pts',(-1.0557204153621,-3.79044252472724,-31.6457605655564));
#16492=CARTESIAN_POINT('Ctrl Pts',(-0.942872669685536,-3.81830854289698,
-31.6398943402759));
#16493=CARTESIAN_POINT('Ctrl Pts',(-0.827382485098032,-3.84682707078469,
-31.633890751667));
#16494=CARTESIAN_POINT('Ctrl Pts',(-0.710646397335317,-3.87008912208951,
-31.6278871630582));
#16495=CARTESIAN_POINT('Ctrl Pts',(-0.593181743754018,-3.88801034192001,
-31.6218835744494));
#16496=CARTESIAN_POINT('Ctrl Pts',(-0.478236988361779,-3.90554710865743,
-31.616008777197));
#16497=CARTESIAN_POINT('Ctrl Pts',(-0.362595031718715,-3.91796990281258,
-31.6101339799445));
#16498=CARTESIAN_POINT('Ctrl Pts',(-0.246744773518751,-3.92525235070832,
-31.6042591826921));
#16499=CARTESIAN_POINT('Ctrl Pts',(-0.127084891449762,-3.93277427487074,
-31.5981911984051));
#16500=CARTESIAN_POINT('Ctrl Pts',(-0.00720325506352192,-3.93481194975495,
-31.5921232141181));
#16501=CARTESIAN_POINT('Ctrl Pts',(0.112363832481439,-3.9313945832427,-31.586055229831));
#16502=CARTESIAN_POINT('Ctrl Pts',(0.231930920026399,-3.92797721673046,
-31.579987245544));
#16503=CARTESIAN_POINT('Ctrl Pts',(0.351182988310738,-3.91910490808594,
-31.573919261257));
#16504=CARTESIAN_POINT('Ctrl Pts',(0.469593286093134,-3.90486506113287,
-31.56785127697));
#16505=CARTESIAN_POINT('Ctrl Pts',(0.584294806373449,-3.89107122626661,
-31.5619733505076));
#16506=CARTESIAN_POINT('Ctrl Pts',(0.698572919306183,-3.87219701765988,
-31.5560954240451));
#16507=CARTESIAN_POINT('Ctrl Pts',(0.811942726654698,-3.84827727803397,
-31.5502174975827));
#16508=CARTESIAN_POINT('Ctrl Pts',(0.925170039140109,-3.82438760320312,
-31.5443469591043));
#16509=CARTESIAN_POINT('Ctrl Pts',(1.03749091658504,-3.79546509425855,-31.5384764206259));
#16510=CARTESIAN_POINT('Ctrl Pts',(1.14842598251843,-3.76159630511789,-31.5326058821475));
#16511=CARTESIAN_POINT('Ctrl Pts',(1.25925109854133,-3.72776108399564,-31.5267411620745));
#16512=CARTESIAN_POINT('Ctrl Pts',(1.36869274309091,-3.68898945429681,-31.5208764420014));
#16513=CARTESIAN_POINT('Ctrl Pts',(1.47628278024491,-3.64541878976234,-31.5150117219284));
#16514=CARTESIAN_POINT('Ctrl Pts',(1.58539396695761,-3.60123210632054,-31.5090640841746));
#16515=CARTESIAN_POINT('Ctrl Pts',(1.69260036333872,-3.55210972764478,-31.5031164464208));
#16516=CARTESIAN_POINT('Ctrl Pts',(1.79743036528644,-3.49824714420612,-31.497168808667));
#16517=CARTESIAN_POINT('Ctrl Pts',(1.90068752249324,-3.4451927023254,-31.4913104078739));
#16518=CARTESIAN_POINT('Ctrl Pts',(2.00163872939307,-3.38753952073739,-31.4854520070808));
#16519=CARTESIAN_POINT('Ctrl Pts',(2.0998550913667,-3.32552215377696,-31.4795936062877));
#16520=CARTESIAN_POINT('Ctrl Pts',(2.19805868078675,-3.26351285186929,-31.4737359673507));
#16521=CARTESIAN_POINT('Ctrl Pts',(2.29352778400063,-3.19714071333686,-31.4678783284138));
#16522=CARTESIAN_POINT('Ctrl Pts',(2.38586080640622,-3.12668469987855,-31.4620206894768));
#16523=CARTESIAN_POINT('Ctrl Pts',(2.47820404212279,-3.05622089300943,-31.4561624026039));
#16524=CARTESIAN_POINT('Ctrl Pts',(2.5674101796388,-2.98167256333388,-31.4503041157309));
#16525=CARTESIAN_POINT('Ctrl Pts',(2.65310970997126,-2.90335975498321,-31.4444458288579));
#16526=CARTESIAN_POINT('Ctrl Pts',(2.74109860687635,-2.82295490803035,-31.4384310444396));
#16527=CARTESIAN_POINT('Ctrl Pts',(2.82539055430386,-2.73858191763267,-31.4324162600212));
#16528=CARTESIAN_POINT('Ctrl Pts',(2.90562603120515,-2.65062754207056,-31.4264014756028));
#16529=CARTESIAN_POINT('Ctrl Pts',(2.98389002092637,-2.56483431679443,-31.4205344820474));
#16530=CARTESIAN_POINT('Ctrl Pts',(3.05829435436076,-2.47563402424389,-31.414667488492));
#16531=CARTESIAN_POINT('Ctrl Pts',(3.12854700286134,-2.38341827023444,-31.4088004949366));
#16532=CARTESIAN_POINT('Ctrl Pts',(3.20145417095092,-2.28771811342087,-31.4027118150868));
#16533=CARTESIAN_POINT('Ctrl Pts',(3.2698894444237,-2.18877053340756,-31.3966231352369));
#16534=CARTESIAN_POINT('Ctrl Pts',(3.33357715425003,-2.08704392782285,-31.3905344553871));
#16535=CARTESIAN_POINT('Ctrl Pts',(3.39726486407637,-1.98531732223815,-31.3844457755372));
#16536=CARTESIAN_POINT('Ctrl Pts',(3.45620482858731,-1.88081215020138,-31.3783570956874));
#16537=CARTESIAN_POINT('Ctrl Pts',(3.51017619113269,-1.77402145060458,-31.3722684158376));
#16538=CARTESIAN_POINT('Ctrl Pts',(3.56572192470471,-1.66411561410128,-31.3660021262203));
#16539=CARTESIAN_POINT('Ctrl Pts',(3.61616462233887,-1.55147512007693,-31.3597358366031));
#16540=CARTESIAN_POINT('Ctrl Pts',(3.66124566739239,-1.43658245951997,-31.3534695469859));
#16541=CARTESIAN_POINT('Ctrl Pts',(3.70619995623913,-1.32201284732672,-31.3472208765499));
#16542=CARTESIAN_POINT('Ctrl Pts',(3.74582253378528,-1.20520400118841,-31.3409722061139));
#16543=CARTESIAN_POINT('Ctrl Pts',(3.77990204431146,-1.08665980665986,-31.3347235356779));
#16544=CARTESIAN_POINT('Ctrl Pts',(3.81392381785851,-0.968316447870441,
-31.3284854516427));
#16545=CARTESIAN_POINT('Ctrl Pts',(3.84242114239712,-0.848243912120649,
-31.3222473676074));
#16546=CARTESIAN_POINT('Ctrl Pts',(3.86523110494377,-0.726964583301815,
-31.3160092835721));
#16547=CARTESIAN_POINT('Ctrl Pts',(3.88798371869111,-0.605990174926128,
-31.3097868833254));
#16548=CARTESIAN_POINT('Ctrl Pts',(3.90507742094504,-0.483815345367452,
-31.3035644830787));
#16549=CARTESIAN_POINT('Ctrl Pts',(3.9163996318116,-0.360974963045875,-31.2973420828319));
#16550=CARTESIAN_POINT('Ctrl Pts',(3.9274254680305,-0.241350098917437,-31.291282562583));
#16551=CARTESIAN_POINT('Ctrl Pts',(3.93297812503326,-0.121094407183991,
-31.285223042334));
#16552=CARTESIAN_POINT('Ctrl Pts',(3.93299993544946,-0.000712568995229939,
-31.2791635220851));
#16553=CARTESIAN_POINT('',(0.654108433901418,3.87822525863301,-31.));
#16554=CARTESIAN_POINT('Ctrl Pts',(3.93299993544964,-0.000712567999896496,
-31.279163522035));
#16555=CARTESIAN_POINT('Ctrl Pts',(3.93302182838837,0.120124919265748,-31.2730810663097));
#16556=CARTESIAN_POINT('Ctrl Pts',(3.92747046918608,0.240887678128942,-31.2669986105844));
#16557=CARTESIAN_POINT('Ctrl Pts',(3.91639254011805,0.3610518961419,-31.260916154859));
#16558=CARTESIAN_POINT('Ctrl Pts',(3.90530392792135,0.481331995904546,-31.2548278334474));
#16559=CARTESIAN_POINT('Ctrl Pts',(3.88867815372494,0.601012040784996,-31.2487395120357));
#16560=CARTESIAN_POINT('Ctrl Pts',(3.86661343148888,0.719575966406443,-31.2426511906241));
#16561=CARTESIAN_POINT('Ctrl Pts',(3.84450626013787,0.838367990693939,-31.2365511562231));
#16562=CARTESIAN_POINT('Ctrl Pts',(3.81693929734249,0.956039245012285,-31.2304511218222));
#16563=CARTESIAN_POINT('Ctrl Pts',(3.78406158109265,1.07208532799334,-31.2243510874212));
#16564=CARTESIAN_POINT('Ctrl Pts',(3.75115008462019,1.18825064256846,-31.2182447855375));
#16565=CARTESIAN_POINT('Ctrl Pts',(3.71291706603387,1.30278710910749,-31.2121384836538));
#16566=CARTESIAN_POINT('Ctrl Pts',(3.66956041237949,1.41520859942883,-31.2060321817701));
#16567=CARTESIAN_POINT('Ctrl Pts',(3.62611689304407,1.52785532782776,-31.1999136458224));
#16568=CARTESIAN_POINT('Ctrl Pts',(3.57752936691509,1.63837827559699,-31.1937951098748));
#16569=CARTESIAN_POINT('Ctrl Pts',(3.52404300556402,1.74631322933068,-31.1876765739272));
#16570=CARTESIAN_POINT('Ctrl Pts',(3.49201630120468,1.81094280528141,-31.1840129008532));
#16571=CARTESIAN_POINT('Ctrl Pts',(3.45823403773063,1.87464498004681,-31.1803492277792));
#16572=CARTESIAN_POINT('Ctrl Pts',(3.42275629611291,1.93732504691894,-31.1766855547052));
#16573=CARTESIAN_POINT('Ctrl Pts',(3.36644302306109,2.03681615203801,-31.1708702628411));
#16574=CARTESIAN_POINT('Ctrl Pts',(3.3056891682797,2.13402452447637,-31.165054970977));
#16575=CARTESIAN_POINT('Ctrl Pts',(3.24070643811116,2.22852210713397,-31.1592396791128));
#16576=CARTESIAN_POINT('Ctrl Pts',(3.1758044980169,2.32290220524297,-31.1534316171367));
#16577=CARTESIAN_POINT('Ctrl Pts',(3.1066843713842,2.41457786870808,-31.1476235551606));
#16578=CARTESIAN_POINT('Ctrl Pts',(3.03360355966315,2.50314570946221,-31.1418154931845));
#16579=CARTESIAN_POINT('Ctrl Pts',(2.95925294581569,2.59325244435111,-31.1359065143018));
#16580=CARTESIAN_POINT('Ctrl Pts',(2.88080291760339,2.68014194914679,-31.1299975354191));
#16581=CARTESIAN_POINT('Ctrl Pts',(2.79857094634214,2.76341992073041,-31.1240885565364));
#16582=CARTESIAN_POINT('Ctrl Pts',(2.71787516654151,2.84514216031779,-31.1182899644383));
#16583=CARTESIAN_POINT('Ctrl Pts',(2.6335378263978,2.92338631305955,-31.1124913723403));
#16584=CARTESIAN_POINT('Ctrl Pts',(2.54589896308285,2.99781378170387,-31.1066927802422));
#16585=CARTESIAN_POINT('Ctrl Pts',(2.45828820621802,3.07221738089284,-31.1008960477967));
#16586=CARTESIAN_POINT('Ctrl Pts',(2.36737835217052,3.1428064560757,-31.0950993153513));
#16587=CARTESIAN_POINT('Ctrl Pts',(2.27354439861573,3.20928105150095,-31.0893025829058));
#16588=CARTESIAN_POINT('Ctrl Pts',(2.1797167497417,3.27575118051414,-31.0835062399414));
#16589=CARTESIAN_POINT('Ctrl Pts',(2.08296573690538,3.33810713625727,-31.077709896977));
#16590=CARTESIAN_POINT('Ctrl Pts',(1.98369668323778,3.39609135167349,-31.0719135540125));
#16591=CARTESIAN_POINT('Ctrl Pts',(1.88106314204737,3.45604080360682,-31.0659207578448));
#16592=CARTESIAN_POINT('Ctrl Pts',(1.77573824618556,3.51131664947634,-31.0599279616771));
#16593=CARTESIAN_POINT('Ctrl Pts',(1.66819802120471,3.56168560685088,-31.0539351655094));
#16594=CARTESIAN_POINT('Ctrl Pts',(1.56406648301076,3.61045802674836,-31.0481323221256));
#16595=CARTESIAN_POINT('Ctrl Pts',(1.45785835084361,3.65462980752974,-31.0423294787417));
#16596=CARTESIAN_POINT('Ctrl Pts',(1.35002535461948,3.69403851386048,-31.0365266353579));
#16597=CARTESIAN_POINT('Ctrl Pts',(1.23689758052407,3.73538225263511,-31.0304388627982));
#16598=CARTESIAN_POINT('Ctrl Pts',(1.12198182485564,3.7714831080146,-31.0243510902386));
#16599=CARTESIAN_POINT('Ctrl Pts',(1.0058150810249,3.80221317429505,-31.0182633176789));
#16600=CARTESIAN_POINT('Ctrl Pts',(0.88964833719417,3.83294324057551,-31.0121755451193));
#16601=CARTESIAN_POINT('Ctrl Pts',(0.772231136853311,3.85830247151174,-31.0060877725596));
#16602=CARTESIAN_POINT('Ctrl Pts',(0.654108433901418,3.87822525863301,-31.));
#16603=CARTESIAN_POINT('',(3.48540987471235,1.82219839898339,-31.));
#16604=CARTESIAN_POINT('Origin',(0.,0.,-31.));
#16605=CARTESIAN_POINT('',(3.92893057216212,-0.00338598511717015,-31.095833725221));
#16606=CARTESIAN_POINT('Ctrl Pts',(3.48540987471235,1.82219839898339,-31.));
#16607=CARTESIAN_POINT('Ctrl Pts',(3.77799362579873,1.26255884722778,-31.0319436609371));
#16608=CARTESIAN_POINT('Ctrl Pts',(3.92425990185113,0.629251789626864,-31.0638873218741));
#16609=CARTESIAN_POINT('Ctrl Pts',(3.92487792373439,-0.00332812842372134,
-31.0958309828112));
#16610=CARTESIAN_POINT('',(3.93299929380719,-0.00235688610855974,-32.3458364779251));
#16611=CARTESIAN_POINT('Ctrl Pts',(3.93299849204801,-0.00344405983004216,
-31.095836477965));
#16612=CARTESIAN_POINT('Ctrl Pts',(3.93288845114196,-0.129107009634538,
-31.1021690432223));
#16613=CARTESIAN_POINT('Ctrl Pts',(3.92675170311396,-0.25460888520464,-31.1085016084795));
#16614=CARTESIAN_POINT('Ctrl Pts',(3.91465899908993,-0.379386242296975,
-31.1148341737368));
#16615=CARTESIAN_POINT('Ctrl Pts',(3.90253790530163,-0.504456536332721,
-31.1211816058125));
#16616=CARTESIAN_POINT('Ctrl Pts',(3.88443295009405,-0.628798615777614,
-31.1275290378882));
#16617=CARTESIAN_POINT('Ctrl Pts',(3.86046608878056,-0.751858083267953,
-31.1338764699639));
#16618=CARTESIAN_POINT('Ctrl Pts',(3.8364193407474,-0.875327734513778,-31.1402450594002));
#16619=CARTESIAN_POINT('Ctrl Pts',(3.80647165118053,-0.997505924425334,
-31.1466136488364));
#16620=CARTESIAN_POINT('Ctrl Pts',(3.77079568576157,-1.11785012244127,-31.1529822382727));
#16621=CARTESIAN_POINT('Ctrl Pts',(3.73505755223346,-1.23840402946294,-31.1593619254651));
#16622=CARTESIAN_POINT('Ctrl Pts',(3.69357130388557,-1.35711727869021,-31.1657416126575));
#16623=CARTESIAN_POINT('Ctrl Pts',(3.64655818641543,-1.47346611535067,-31.1721212998499));
#16624=CARTESIAN_POINT('Ctrl Pts',(3.59943219296957,-1.59009429933308,-31.1785163043293));
#16625=CARTESIAN_POINT('Ctrl Pts',(3.54675291703733,-1.70434644496144,-31.1849113088088));
#16626=CARTESIAN_POINT('Ctrl Pts',(3.48878881390637,-1.81572068665909,-31.1913063132883));
#16627=CARTESIAN_POINT('Ctrl Pts',(3.47586798582981,-1.84054721465491,-31.1927318292363));
#16628=CARTESIAN_POINT('Ctrl Pts',(3.46268473224403,-1.86523085121481,-31.1941573451844));
#16629=CARTESIAN_POINT('Ctrl Pts',(3.44924232171538,-1.8897662305395,-31.1955828611324));
#16630=CARTESIAN_POINT('Ctrl Pts',(3.39423695124737,-1.99016322603759,-31.201415969165));
#16631=CARTESIAN_POINT('Ctrl Pts',(3.33474002976474,-2.08834716632629,-31.2072490771975));
#16632=CARTESIAN_POINT('Ctrl Pts',(3.27095393633534,-2.1838840047888,-31.21308218523));
#16633=CARTESIAN_POINT('Ctrl Pts',(3.20725631784468,-2.27928832822371,-31.2189072024099));
#16634=CARTESIAN_POINT('Ctrl Pts',(3.13928158462642,-2.372052503483,-31.2247322195899));
#16635=CARTESIAN_POINT('Ctrl Pts',(3.06727850060632,-2.46176595144994,-31.2305572367698));
#16636=CARTESIAN_POINT('Ctrl Pts',(2.99535532717324,-2.55137983348317,-31.2363757892192));
#16637=CARTESIAN_POINT('Ctrl Pts',(2.91941295315617,-2.6379493951853,-31.2421943416685));
#16638=CARTESIAN_POINT('Ctrl Pts',(2.83974361914423,-2.72109264405489,-31.2480128941179));
#16639=CARTESIAN_POINT('Ctrl Pts',(2.75807317376219,-2.80632426108675,-31.2539775952906));
#16640=CARTESIAN_POINT('Ctrl Pts',(2.67248628543714,-2.88795476940036,-31.2599422964634));
#16641=CARTESIAN_POINT('Ctrl Pts',(2.58334229389153,-2.96560813200114,-31.2659069976362));
#16642=CARTESIAN_POINT('Ctrl Pts',(2.49649679742058,-3.04125927472848,-31.271717904526));
#16643=CARTESIAN_POINT('Ctrl Pts',(2.4062757346846,-3.11313557650278,-31.2775288114157));
#16644=CARTESIAN_POINT('Ctrl Pts',(2.3130483080209,-3.18092699142273,-31.2833397183054));
#16645=CARTESIAN_POINT('Ctrl Pts',(2.21983983305758,-3.24870462539184,-31.2891494439273));
#16646=CARTESIAN_POINT('Ctrl Pts',(2.12362654842139,-3.31239877639275,-31.2949591695491));
#16647=CARTESIAN_POINT('Ctrl Pts',(2.02480914457453,-3.37174093430195,-31.300768895171));
#16648=CARTESIAN_POINT('Ctrl Pts',(1.92598704856082,-3.43108590996687,-31.3065788966572));
#16649=CARTESIAN_POINT('Ctrl Pts',(1.82456094781493,-3.48607826618171,-31.3123888981434));
#16650=CARTESIAN_POINT('Ctrl Pts',(1.72095810138853,-3.53649433949288,-31.3181988996296));
#16651=CARTESIAN_POINT('Ctrl Pts',(1.61253055425839,-3.58925824853226,-31.3242794681825));
#16652=CARTESIAN_POINT('Ctrl Pts',(1.50171907493652,-3.63700911638447,-31.3303600367355));
#16653=CARTESIAN_POINT('Ctrl Pts',(1.38903784788383,-3.67954655591504,-31.3364406052884));
#16654=CARTESIAN_POINT('Ctrl Pts',(1.2812187115245,-3.720248544286,-31.3422588029341));
#16655=CARTESIAN_POINT('Ctrl Pts',(1.1716882509613,-3.75617757405178,-31.3480770005797));
#16656=CARTESIAN_POINT('Ctrl Pts',(1.06091210127569,-3.78720933054496,-31.3538951982254));
#16657=CARTESIAN_POINT('Ctrl Pts',(0.950061720735049,-3.81826188135013,
-31.3597172946326));
#16658=CARTESIAN_POINT('Ctrl Pts',(0.83796439726712,-3.84441053232061,-31.3655393910397));
#16659=CARTESIAN_POINT('Ctrl Pts',(0.725095303676809,-3.86558220719542,
-31.3713614874469));
#16660=CARTESIAN_POINT('Ctrl Pts',(0.612067657769103,-3.88678362287888,
-31.377191762416));
#16661=CARTESIAN_POINT('Ctrl Pts',(0.498266492570521,-3.90299405740786,
-31.3830220373852));
#16662=CARTESIAN_POINT('Ctrl Pts',(0.384171317235336,-3.91419230480743,
-31.3888523123543));
#16663=CARTESIAN_POINT('Ctrl Pts',(0.36908061049378,-3.91567343200697,-31.3896234489911));
#16664=CARTESIAN_POINT('Ctrl Pts',(0.353984758379108,-3.91706695155966,
-31.3903945856279));
#16665=CARTESIAN_POINT('Ctrl Pts',(0.338884867325807,-3.91837288254928,
-31.3911657222647));
#16666=CARTESIAN_POINT('Ctrl Pts',(0.223539665693932,-3.92834864149907,
-31.397056288663));
#16667=CARTESIAN_POINT('Ctrl Pts',(0.107572026652748,-3.93324268448918,
-31.4029468550613));
#16668=CARTESIAN_POINT('Ctrl Pts',(-0.00853435788344206,-3.93299074048433,
-31.4088374214595));
#16669=CARTESIAN_POINT('Ctrl Pts',(-0.124495126349702,-3.93273911245777,
-31.4147206001407));
#16670=CARTESIAN_POINT('Ctrl Pts',(-0.240593887336033,-3.92735433517721,
-31.4206037788218));
#16671=CARTESIAN_POINT('Ctrl Pts',(-0.356341900523714,-3.91682389825368,
-31.4264869575029));
#16672=CARTESIAN_POINT('Ctrl Pts',(-0.47197512477886,-3.90630390451254,
-31.432364301753));
#16673=CARTESIAN_POINT('Ctrl Pts',(-0.587257886849221,-3.89064844015712,
-31.4382416460031));
#16674=CARTESIAN_POINT('Ctrl Pts',(-0.701702152312787,-3.86989703860963,
-31.4441189902532));
#16675=CARTESIAN_POINT('Ctrl Pts',(-0.817422920671509,-3.84891417745998,
-31.4500618899676));
#16676=CARTESIAN_POINT('Ctrl Pts',(-0.932285946629697,-3.82272100001071,
-31.4560047896819));
#16677=CARTESIAN_POINT('Ctrl Pts',(-1.04579232132231,-3.79141232532987,
-31.4619476893962));
#16678=CARTESIAN_POINT('Ctrl Pts',(-1.15792355827808,-3.7604829574515,-31.4678185904613));
#16679=CARTESIAN_POINT('Ctrl Pts',(-1.26873043180122,-3.72456148096188,
-31.4736894915263));
#16680=CARTESIAN_POINT('Ctrl Pts',(-1.37774352204889,-3.68379041035892,
-31.4795603925913));
#16681=CARTESIAN_POINT('Ctrl Pts',(-1.48674117497777,-3.64302511333794,
-31.4854304622794));
#16682=CARTESIAN_POINT('Ctrl Pts',(-1.59394516568978,-3.59741173182533,
-31.4913005319675));
#16683=CARTESIAN_POINT('Ctrl Pts',(-1.69890371294145,-3.54714183169404,
-31.4971706016556));
#16684=CARTESIAN_POINT('Ctrl Pts',(-1.80387234132728,-3.49686710320316,
-31.5030412351564));
#16685=CARTESIAN_POINT('Ctrl Pts',(-1.90659472750348,-3.4419351442463,-31.5089118686571));
#16686=CARTESIAN_POINT('Ctrl Pts',(-2.0066420688035,-3.38258430903178,-31.5147825021579));
#16687=CARTESIAN_POINT('Ctrl Pts',(-2.10884590380171,-3.32195418242921,
-31.5207796755945));
#16688=CARTESIAN_POINT('Ctrl Pts',(-2.208257657063,-3.25671271250808,-31.5267768490311));
#16689=CARTESIAN_POINT('Ctrl Pts',(-2.30445085540019,-3.18716100237269,
-31.5327740224677));
#16690=CARTESIAN_POINT('Ctrl Pts',(-2.3987488390712,-3.11897961179613,-31.5386530385788));
#16691=CARTESIAN_POINT('Ctrl Pts',(-2.48995363833394,-3.04665656586699,
-31.5445320546898));
#16692=CARTESIAN_POINT('Ctrl Pts',(-2.5776973771932,-2.97051598743573,-31.5504110708008));
#16693=CARTESIAN_POINT('Ctrl Pts',(-2.66808634579564,-2.89207998228404,
-31.5564673229002));
#16694=CARTESIAN_POINT('Ctrl Pts',(-2.75480192024057,-2.80959294879769,
-31.5625235749996));
#16695=CARTESIAN_POINT('Ctrl Pts',(-2.837484066154,-2.72344876476906,-31.568579827099));
#16696=CARTESIAN_POINT('Ctrl Pts',(-2.92016621206744,-2.63730458074044,
-31.5746360791984));
#16697=CARTESIAN_POINT('Ctrl Pts',(-2.99881466652138,-2.54750364007306,
-31.5806923312978));
#16698=CARTESIAN_POINT('Ctrl Pts',(-3.07311643582633,-2.45447435754666,
-31.5867485833971));
#16699=CARTESIAN_POINT('Ctrl Pts',(-3.14542210974768,-2.36394427959004,
-31.5926421360484));
#16700=CARTESIAN_POINT('Ctrl Pts',(-3.21383489080398,-2.2700777034157,-31.5985356886997));
#16701=CARTESIAN_POINT('Ctrl Pts',(-3.27803367643307,-2.17324278813268,
-31.604429241351));
#16702=CARTESIAN_POINT('Ctrl Pts',(-3.34215395399215,-2.07652629132492,
-31.6103155868342));
#16703=CARTESIAN_POINT('Ctrl Pts',(-3.40207026179529,-1.97684901452301,
-31.6162019323173));
#16704=CARTESIAN_POINT('Ctrl Pts',(-3.45750187819924,-1.87461189643316,
-31.6220882778004));
#16705=CARTESIAN_POINT('Ctrl Pts',(-3.51288020561038,-1.77247306364337,
-31.6279689644657));
#16706=CARTESIAN_POINT('Ctrl Pts',(-3.56378222474554,-1.66777964389323,
-31.6338496511309));
#16707=CARTESIAN_POINT('Ctrl Pts',(-3.60997100205417,-1.56096071838083,
-31.6397303377962));
#16708=CARTESIAN_POINT('Ctrl Pts',(-3.65663909781835,-1.45303329237582,
-31.6456720505767));
#16709=CARTESIAN_POINT('Ctrl Pts',(-3.6984953340556,-1.34293634713679,-31.6516137633573));
#16710=CARTESIAN_POINT('Ctrl Pts',(-3.73534330456992,-1.23113744033909,
-31.6575554761379));
#16711=CARTESIAN_POINT('Ctrl Pts',(-3.77177541596714,-1.12060027452805,
-31.6634301318893));
#16712=CARTESIAN_POINT('Ctrl Pts',(-3.80331160853401,-1.0083997689392,-31.6693047876408));
#16713=CARTESIAN_POINT('Ctrl Pts',(-3.8298110422003,-0.895006358100695,
-31.6751794433922));
#16714=CARTESIAN_POINT('Ctrl Pts',(-3.85630739569812,-0.781626127574343,
-31.6810534163016));
#16715=CARTESIAN_POINT('Ctrl Pts',(-3.87776806151683,-0.667053666515133,
-31.6869273892109));
#16716=CARTESIAN_POINT('Ctrl Pts',(-3.89410283350252,-0.551771802566638,
-31.6928013621203));
#16717=CARTESIAN_POINT('Ctrl Pts',(-3.91043957582767,-0.436476033042626,
-31.6986760435623));
#16718=CARTESIAN_POINT('Ctrl Pts',(-3.9216491374739,-0.320471096193623,
-31.7045507250044));
#16719=CARTESIAN_POINT('Ctrl Pts',(-3.92769300733848,-0.204246517973773,
-31.7104254064465));
#16720=CARTESIAN_POINT('Ctrl Pts',(-3.93385774921905,-0.0856975516728088,
-31.7164175762867));
#16721=CARTESIAN_POINT('Ctrl Pts',(-3.93464793608923,0.0330794915937387,
-31.722409746127));
#16722=CARTESIAN_POINT('Ctrl Pts',(-3.9300785144255,0.151564740131223,-31.7284019159672));
#16723=CARTESIAN_POINT('Ctrl Pts',(-3.92559204599207,0.267899008778536,
-31.7342853040225));
#16724=CARTESIAN_POINT('Ctrl Pts',(-3.91593901857735,0.383951580272443,
-31.7401686920779));
#16725=CARTESIAN_POINT('Ctrl Pts',(-3.90118599137473,0.49923627742943,-31.7460520801332));
#16726=CARTESIAN_POINT('Ctrl Pts',(-3.88602379671181,0.61771833510769,-31.7520986408659));
#16727=CARTESIAN_POINT('Ctrl Pts',(-3.86547465590248,0.735388840375355,
-31.7581452015986));
#16728=CARTESIAN_POINT('Ctrl Pts',(-3.83966659809232,0.851733183276386,
-31.7641917623313));
#16729=CARTESIAN_POINT('Ctrl Pts',(-3.81385854028217,0.968077526177417,
-31.7702383230641));
#16730=CARTESIAN_POINT('Ctrl Pts',(-3.78279174634404,1.08309527567172,-31.7762848837968));
#16731=CARTESIAN_POINT('Ctrl Pts',(-3.74664851272451,1.19629173787134,-31.7823314445295));
#16732=CARTESIAN_POINT('Ctrl Pts',(-3.71151110362466,1.30633807303971,-31.7882097364485));
#16733=CARTESIAN_POINT('Ctrl Pts',(-3.67146411556804,1.41501373852729,-31.7940880283675));
#16734=CARTESIAN_POINT('Ctrl Pts',(-3.6266326806316,1.5218490068909,-31.7999663202865));
#16735=CARTESIAN_POINT('Ctrl Pts',(-3.58185810939464,1.62854876657401,-31.8058371562447));
#16736=CARTESIAN_POINT('Ctrl Pts',(-3.53231131853186,1.73341239476686,-31.8117079922028));
#16737=CARTESIAN_POINT('Ctrl Pts',(-3.47816719981031,1.83598527503999,-31.8175788281609));
#16738=CARTESIAN_POINT('Ctrl Pts',(-3.42407736618943,1.93845531535078,-31.8234437779965));
#16739=CARTESIAN_POINT('Ctrl Pts',(-3.36539956498137,2.03863881380937,-31.829308727832));
#16740=CARTESIAN_POINT('Ctrl Pts',(-3.30235650108527,2.13610171568206,-31.8351736776675));
#16741=CARTESIAN_POINT('Ctrl Pts',(-3.23842581409762,2.23493685927217,-31.841121203834));
#16742=CARTESIAN_POINT('Ctrl Pts',(-3.17000616205701,2.33097380993132,-31.8470687300004));
#16743=CARTESIAN_POINT('Ctrl Pts',(-3.09737794932883,2.423786054711,-31.8530162561668));
#16744=CARTESIAN_POINT('Ctrl Pts',(-3.02583733452349,2.51520844834546,-31.858874718912));
#16745=CARTESIAN_POINT('Ctrl Pts',(-2.95021360718964,2.60350172132222,-31.8647331816572));
#16746=CARTESIAN_POINT('Ctrl Pts',(-2.87081757249818,2.68828857555056,-31.8705916444024));
#16747=CARTESIAN_POINT('Ctrl Pts',(-2.79143271514784,2.77306349352042,-31.8764492823956));
#16748=CARTESIAN_POINT('Ctrl Pts',(-2.70827688832753,2.8543326735494,-31.8823069203888));
#16749=CARTESIAN_POINT('Ctrl Pts',(-2.62169940402785,2.93175395197483,-31.888164558382));
#16750=CARTESIAN_POINT('Ctrl Pts',(-2.53511327273959,3.00918296290618,-31.894022781411));
#16751=CARTESIAN_POINT('Ctrl Pts',(-2.44510511203493,3.08276303347397,-31.89988100444));
#16752=CARTESIAN_POINT('Ctrl Pts',(-2.35205857871393,3.15219121283881,-31.905739227469));
#16753=CARTESIAN_POINT('Ctrl Pts',(-2.25652846112328,3.22347255887184,-31.9117538173184));
#16754=CARTESIAN_POINT('Ctrl Pts',(-2.15779584488271,3.29037695920454,-31.9177684071678));
#16755=CARTESIAN_POINT('Ctrl Pts',(-2.05630804007415,3.3526237850863,-31.9237829970172));
#16756=CARTESIAN_POINT('Ctrl Pts',(-1.95731441833698,3.41334082145636,-31.9296497711935));
#16757=CARTESIAN_POINT('Ctrl Pts',(-1.85569985651786,3.46962641060938,-31.9355165453697));
#16758=CARTESIAN_POINT('Ctrl Pts',(-1.75190378738148,3.52126711848994,-31.941383319546));
#16759=CARTESIAN_POINT('Ctrl Pts',(-1.64418494432331,3.57485948816136,-31.947471817232));
#16760=CARTESIAN_POINT('Ctrl Pts',(-1.53411690652952,3.62344876785874,-31.9535603149179));
#16761=CARTESIAN_POINT('Ctrl Pts',(-1.422211510523,3.66685197674189,-31.9596488126039));
#16762=CARTESIAN_POINT('Ctrl Pts',(-1.31030611451649,3.71025518562503,-31.9657373102899));
#16763=CARTESIAN_POINT('Ctrl Pts',(-1.19656384528513,3.74847223088484,-31.9718258079759));
#16764=CARTESIAN_POINT('Ctrl Pts',(-1.08151049659051,3.78137859064185,-31.9779143056618));
#16765=CARTESIAN_POINT('Ctrl Pts',(-0.970285561707589,3.81318998737853,
-31.9838002078658));
#16766=CARTESIAN_POINT('Ctrl Pts',(-0.857479633024243,3.84014032372034,
-31.9896861100698));
#16767=CARTESIAN_POINT('Ctrl Pts',(-0.743554482563883,3.86207401941744,
-31.9955720122738));
#16768=CARTESIAN_POINT('Ctrl Pts',(-0.62977194254846,3.88398025871803,-32.0014505465601));
#16769=CARTESIAN_POINT('Ctrl Pts',(-0.514873367582792,3.90088227040903,
-32.0073290808463));
#16770=CARTESIAN_POINT('Ctrl Pts',(-0.399335407964658,3.91267430690898,
-32.0132076151326));
#16771=CARTESIAN_POINT('Ctrl Pts',(-0.283911607503072,3.92445469209585,
-32.0190803410377));
#16772=CARTESIAN_POINT('Ctrl Pts',(-0.167850085885753,3.93113510480027,
-32.0249530669427));
#16773=CARTESIAN_POINT('Ctrl Pts',(-0.0516367685391186,3.93266101312265,
-32.0308257928478));
#16774=CARTESIAN_POINT('Ctrl Pts',(0.0659996431599903,3.9342056070102,-32.0367704334289));
#16775=CARTESIAN_POINT('Ctrl Pts',(0.183791173653705,3.93046852614243,-32.04271507401));
#16776=CARTESIAN_POINT('Ctrl Pts',(0.301229032194601,3.92144744579895,-32.0486597145911));
#16777=CARTESIAN_POINT('Ctrl Pts',(0.417120827942007,3.91254512747012,-32.0545260943138));
#16778=CARTESIAN_POINT('Ctrl Pts',(0.532667787277854,3.89849714383648,-32.0603924740364));
#16779=CARTESIAN_POINT('Ctrl Pts',(0.647382560249071,3.87935366017142,-32.0662588537591));
#16780=CARTESIAN_POINT('Ctrl Pts',(0.762081961465147,3.86021274172908,-32.0721244473881));
#16781=CARTESIAN_POINT('Ctrl Pts',(0.875948992750114,3.83597774888851,-32.0779900410171));
#16782=CARTESIAN_POINT('Ctrl Pts',(0.988504258375365,3.8067503636532,-32.0838556346462));
#16783=CARTESIAN_POINT('Ctrl Pts',(1.10107132092402,3.77751991509409,-32.0897218430484));
#16784=CARTESIAN_POINT('Ctrl Pts',(1.21232594663721,3.74329613725687,-32.0955880514506));
#16785=CARTESIAN_POINT('Ctrl Pts',(1.32180237773559,3.70423102333164,-32.1014542598528));
#16786=CARTESIAN_POINT('Ctrl Pts',(1.43384238434553,3.66425113379296,-32.1074578354312));
#16787=CARTESIAN_POINT('Ctrl Pts',(1.54401945122707,3.61920049195865,-32.1134614110097));
#16788=CARTESIAN_POINT('Ctrl Pts',(1.65185562922367,3.56929432524163,-32.1194649865881));
#16789=CARTESIAN_POINT('Ctrl Pts',(1.75737803034139,3.52045896552841,-32.1253397470081));
#16790=CARTESIAN_POINT('Ctrl Pts',(1.860658644922,3.46697459450396,-32.131214507428));
#16791=CARTESIAN_POINT('Ctrl Pts',(1.96127524441245,3.40908908884102,-32.1370892678479));
#16792=CARTESIAN_POINT('Ctrl Pts',(2.06520115584614,3.34929971049503,-32.1431572510056));
#16793=CARTESIAN_POINT('Ctrl Pts',(2.16628438487693,3.28481495921471,-32.1492252341633));
#16794=CARTESIAN_POINT('Ctrl Pts',(2.26409384522701,3.21595523289818,-32.1552932173211));
#16795=CARTESIAN_POINT('Ctrl Pts',(2.3619033055771,3.14709550658164,-32.1613612004788));
#16796=CARTESIAN_POINT('Ctrl Pts',(2.45643865972793,3.07386114764121,-32.1674291836365));
#16797=CARTESIAN_POINT('Ctrl Pts',(2.54730890847625,2.99661581201154,-32.1734971667942));
#16798=CARTESIAN_POINT('Ctrl Pts',(2.63427423100519,2.92268990535426,-32.1793043932482));
#16799=CARTESIAN_POINT('Ctrl Pts',(2.7181748340813,2.84484219312201,-32.1851116197022));
#16800=CARTESIAN_POINT('Ctrl Pts',(2.79863052019651,2.76335958778886,-32.1909188461562));
#16801=CARTESIAN_POINT('Ctrl Pts',(2.87898489175215,2.6819795901727,-32.1967187598071));
#16802=CARTESIAN_POINT('Ctrl Pts',(2.95590267489068,2.59697409683223,-32.202518673458));
#16803=CARTESIAN_POINT('Ctrl Pts',(3.02903642612008,2.50867043057427,-32.2083185871088));
#16804=CARTESIAN_POINT('Ctrl Pts',(3.10209185833723,2.42046132880675,-32.214112289626));
#16805=CARTESIAN_POINT('Ctrl Pts',(3.17137105156308,2.32896140468738,-32.2199059921432));
#16806=CARTESIAN_POINT('Ctrl Pts',(3.23656382083118,2.23453432143852,-32.2256996946603));
#16807=CARTESIAN_POINT('Ctrl Pts',(3.30171799691789,2.14016313766427,-32.231489967389));
#16808=CARTESIAN_POINT('Ctrl Pts',(3.36279031607265,2.04286858521363,-32.2372802401176));
#16809=CARTESIAN_POINT('Ctrl Pts',(3.41951159785563,1.94304643077071,-32.2430705128463));
#16810=CARTESIAN_POINT('Ctrl Pts',(3.47621377014188,1.84325790658216,-32.2488588348221));
#16811=CARTESIAN_POINT('Ctrl Pts',(3.52856760988196,1.74094384073624,-32.254647156798));
#16812=CARTESIAN_POINT('Ctrl Pts',(3.57634837369138,1.63652721028251,-32.2604354787739));
#16813=CARTESIAN_POINT('Ctrl Pts',(3.62412522745937,1.53211912455092,-32.2662233270742));
#16814=CARTESIAN_POINT('Ctrl Pts',(3.66732957434697,1.42560920173296,-32.2720111753745));
#16815=CARTESIAN_POINT('Ctrl Pts',(3.70578394079474,1.31744236463982,-32.2777990236749));
#16816=CARTESIAN_POINT('Ctrl Pts',(3.74426510439598,1.20920015084436,-32.2835909052716));
#16817=CARTESIAN_POINT('Ctrl Pts',(3.77798953120207,1.09929911511907,-32.2893827868684));
#16818=CARTESIAN_POINT('Ctrl Pts',(3.80682902228904,0.98820129278295,-32.2951746684652));
#16819=CARTESIAN_POINT('Ctrl Pts',(3.83567813033554,0.877066423216763,-32.3009684814515));
#16820=CARTESIAN_POINT('Ctrl Pts',(3.85963896757854,0.764734386023264,-32.3067622944377));
#16821=CARTESIAN_POINT('Ctrl Pts',(3.87863444631211,0.651677705527191,-32.312556107424));
#16822=CARTESIAN_POINT('Ctrl Pts',(3.8976559144384,0.538466342197817,-32.3183578474378));
#16823=CARTESIAN_POINT('Ctrl Pts',(3.91169839772483,0.424528775291612,-32.3241595874515));
#16824=CARTESIAN_POINT('Ctrl Pts',(3.92073667789608,0.310343201311663,-32.3299613274652));
#16825=CARTESIAN_POINT('Ctrl Pts',(3.92898041496336,0.206195528200064,-32.3352530442852));
#16826=CARTESIAN_POINT('Ctrl Pts',(3.9330617358394,0.101841813893803,-32.3405447611052));
#16827=CARTESIAN_POINT('Ctrl Pts',(3.93299929380719,-0.00235688610856188,
-32.3458364779251));
#16828=CARTESIAN_POINT('',(3.93299863980535,0.00327097680709692,-33.5958364779274));
#16829=CARTESIAN_POINT('Ctrl Pts',(3.93299929380672,-0.00235688689347031,
-32.345836477965));
#16830=CARTESIAN_POINT('Ctrl Pts',(3.93290786947772,-0.154919074919968,
-32.3535843279522));
#16831=CARTESIAN_POINT('Ctrl Pts',(3.92393949909681,-0.307206649636701,
-32.3613321779394));
#16832=CARTESIAN_POINT('Ctrl Pts',(3.9061895909518,-0.458445067090745,-32.3690800279266));
#16833=CARTESIAN_POINT('Ctrl Pts',(3.89271012912065,-0.573297068510666,
-32.3749638244692));
#16834=CARTESIAN_POINT('Ctrl Pts',(3.87413948421733,-0.687737169573374,
-32.3808476210119));
#16835=CARTESIAN_POINT('Ctrl Pts',(3.85051165487551,-0.801279598934025,
-32.3867314175545));
#16836=CARTESIAN_POINT('Ctrl Pts',(3.82691348143223,-0.914679518260579,
-32.3926078291923));
#16837=CARTESIAN_POINT('Ctrl Pts',(3.79827083100888,-1.02718360738723,-32.39848424083));
#16838=CARTESIAN_POINT('Ctrl Pts',(3.7646694235675,-1.1383115264531,-32.4043606524677));
#16839=CARTESIAN_POINT('Ctrl Pts',(3.73110130936551,-1.24932933678556,-32.410231241588));
#16840=CARTESIAN_POINT('Ctrl Pts',(3.69258433062127,-1.35897329793973,-32.4161018307083));
#16841=CARTESIAN_POINT('Ctrl Pts',(3.64925504953696,-1.46677421010494,-32.4219724198286));
#16842=CARTESIAN_POINT('Ctrl Pts',(3.60537334162382,-1.575949530397,-32.4279178560465));
#16843=CARTESIAN_POINT('Ctrl Pts',(3.55655585067352,-1.68323405766395,-32.4338632922645));
#16844=CARTESIAN_POINT('Ctrl Pts',(3.50299642499465,-1.78815688530808,-32.4398087284824));
#16845=CARTESIAN_POINT('Ctrl Pts',(3.45016861389524,-1.89164648118303,-32.4456729508381));
#16846=CARTESIAN_POINT('Ctrl Pts',(3.39272780919716,-1.99283812295064,-32.4515371731938));
#16847=CARTESIAN_POINT('Ctrl Pts',(3.33090777942233,-2.09130159589281,-32.4574013955495));
#16848=CARTESIAN_POINT('Ctrl Pts',(3.26909607629266,-2.18975180662201,-32.4632648280431));
#16849=CARTESIAN_POINT('Ctrl Pts',(3.2029065398853,-2.2854742310021,-32.4691282605367));
#16850=CARTESIAN_POINT('Ctrl Pts',(3.1326174228084,-2.37806582800335,-32.4749916930303));
#16851=CARTESIAN_POINT('Ctrl Pts',(3.0623209512491,-2.47066711303738,-32.4808557390258));
#16852=CARTESIAN_POINT('Ctrl Pts',(2.9879242950677,-2.5601365918027,-32.4867197850214));
#16853=CARTESIAN_POINT('Ctrl Pts',(2.90974688741391,-2.64610318226351,-32.492583831017));
#16854=CARTESIAN_POINT('Ctrl Pts',(2.82966915740579,-2.73415943313237,-32.4985904191871));
#16855=CARTESIAN_POINT('Ctrl Pts',(2.74562479919922,-2.81853996037597,-32.5045970073573));
#16856=CARTESIAN_POINT('Ctrl Pts',(2.65799729820821,-2.89888588301055,-32.5106035955274));
#16857=CARTESIAN_POINT('Ctrl Pts',(2.57232427483763,-2.97743973916022,-32.5164762104355));
#16858=CARTESIAN_POINT('Ctrl Pts',(2.48322663197954,-3.0521368632481,-32.5223488253436));
#16859=CARTESIAN_POINT('Ctrl Pts',(2.39109555004112,-3.12268331256526,-32.5282214402517));
#16860=CARTESIAN_POINT('Ctrl Pts',(2.29581175799552,-3.1956438494966,-32.5342950150529));
#16861=CARTESIAN_POINT('Ctrl Pts',(2.19728360198152,-3.26416427734106,-32.5403685898541));
#16862=CARTESIAN_POINT('Ctrl Pts',(2.09597436760318,-3.32796941848186,-32.5464421646553));
#16863=CARTESIAN_POINT('Ctrl Pts',(1.99466513322484,-3.39177455962266,-32.5525157394565));
#16864=CARTESIAN_POINT('Ctrl Pts',(1.89057526983297,-3.45086423343124,-32.5585893142577));
#16865=CARTESIAN_POINT('Ctrl Pts',(1.78419264010639,-3.50501720723168,-32.5646628890589));
#16866=CARTESIAN_POINT('Ctrl Pts',(1.68111551557648,-3.55748754791079,-32.5705477466501));
#16867=CARTESIAN_POINT('Ctrl Pts',(1.57555808635996,-3.60549039330302,-32.5764326042414));
#16868=CARTESIAN_POINT('Ctrl Pts',(1.46794369784586,-3.64878477029745,-32.5823174618327));
#16869=CARTESIAN_POINT('Ctrl Pts',(1.36046410956057,-3.69202491577131,-32.5881949479176));
#16870=CARTESIAN_POINT('Ctrl Pts',(1.25093306492191,-3.73056817116982,-32.5940724340025));
#16871=CARTESIAN_POINT('Ctrl Pts',(1.13979804754758,-3.76421962839667,-32.5999499200874));
#16872=CARTESIAN_POINT('Ctrl Pts',(1.02877290005148,-3.79783781724784,-32.6058215955943));
#16873=CARTESIAN_POINT('Ctrl Pts',(0.916147325773982,-3.82657371003728,
-32.6116932711013));
#16874=CARTESIAN_POINT('Ctrl Pts',(0.802387709503257,-3.85028089412164,
-32.6175649466082));
#16875=CARTESIAN_POINT('Ctrl Pts',(0.687206833635811,-3.87428426470869,
-32.6235099800909));
#16876=CARTESIAN_POINT('Ctrl Pts',(0.570863781666884,-3.89313225162008,
-32.6294550135735));
#16877=CARTESIAN_POINT('Ctrl Pts',(0.453857729347805,-3.9067252477633,-32.6354000470561));
#16878=CARTESIAN_POINT('Ctrl Pts',(0.338420326141269,-3.92013600853567,
-32.6412653780677));
#16879=CARTESIAN_POINT('Ctrl Pts',(0.222338012342579,-3.92843178006083,
-32.6471307090793));
#16880=CARTESIAN_POINT('Ctrl Pts',(0.106098594155559,-3.93156865491603,
-32.6529960400909));
#16881=CARTESIAN_POINT('Ctrl Pts',(-0.010125296343861,-3.93470511073598,
-32.65886058759));
#16882=CARTESIAN_POINT('Ctrl Pts',(-0.126505838513776,-3.932684029393,-32.6647251350892));
#16883=CARTESIAN_POINT('Ctrl Pts',(-0.242553186744214,-3.9255135908057,
-32.6705896825884));
#16884=CARTESIAN_POINT('Ctrl Pts',(-0.358612775602586,-3.91834239588339,
-32.6764548486777));
#16885=CARTESIAN_POINT('Ctrl Pts',(-0.47433869020946,-3.90602078932509,
-32.682320014767));
#16886=CARTESIAN_POINT('Ctrl Pts',(-0.589244857220856,-3.88860894128463,
-32.6881851808563));
#16887=CARTESIAN_POINT('Ctrl Pts',(-0.70689148036391,-3.8707818291468,-32.6941902283009));
#16888=CARTESIAN_POINT('Ctrl Pts',(-0.823678309532684,-3.84761865795514,
-32.7001952757455));
#16889=CARTESIAN_POINT('Ctrl Pts',(-0.939094590741654,-3.81923949885835,
-32.7062003231901));
#16890=CARTESIAN_POINT('Ctrl Pts',(-1.05198710792769,-3.79148089606418,
-32.712074060541));
#16891=CARTESIAN_POINT('Ctrl Pts',(-1.16356801858427,-3.75873225249553,
-32.7179477978919));
#16892=CARTESIAN_POINT('Ctrl Pts',(-1.27337566660935,-3.72115619286361,
-32.7238215352428));
#16893=CARTESIAN_POINT('Ctrl Pts',(-1.38686551517042,-3.68232008814917,
-32.7298922377342));
#16894=CARTESIAN_POINT('Ctrl Pts',(-1.49846063602563,-3.63832730397798,
-32.7359629402257));
#16895=CARTESIAN_POINT('Ctrl Pts',(-1.60767595214863,-3.58941040184638,
-32.7420336427171));
#16896=CARTESIAN_POINT('Ctrl Pts',(-1.71689126827162,-3.54049349971479,
-32.7481043452085));
#16897=CARTESIAN_POINT('Ctrl Pts',(-1.82372638164384,-3.48665275234288,
-32.7541750476999));
#16898=CARTESIAN_POINT('Ctrl Pts',(-1.92772739141904,-3.42817095611825,
-32.7602457501914));
#16899=CARTESIAN_POINT('Ctrl Pts',(-2.02854192543948,-3.37148097735932,
-32.766130453082));
#16900=CARTESIAN_POINT('Ctrl Pts',(-2.12701386129577,-3.31025008180474,
-32.7720151559726));
#16901=CARTESIAN_POINT('Ctrl Pts',(-2.22270794992252,-3.24469696109686,
-32.7778998588632));
#16902=CARTESIAN_POINT('Ctrl Pts',(-2.31828216821603,-3.1792259549118,-32.783777190334));
#16903=CARTESIAN_POINT('Ctrl Pts',(-2.41108512357713,-3.10944372242548,
-32.7896545218048));
#16904=CARTESIAN_POINT('Ctrl Pts',(-2.50070651882283,-3.03561458467919,
-32.7955318532757));
#16905=CARTESIAN_POINT('Ctrl Pts',(-2.59023931497713,-2.96185843390778,
-32.8014033744573));
#16906=CARTESIAN_POINT('Ctrl Pts',(-2.67659649230363,-2.88406359674231,
-32.8072748956388));
#16907=CARTESIAN_POINT('Ctrl Pts',(-2.75939763216431,-2.80253701270937,
-32.8131464168204));
#16908=CARTESIAN_POINT('Ctrl Pts',(-2.84323627165616,-2.71998889925055,
-32.8190915082581));
#16909=CARTESIAN_POINT('Ctrl Pts',(-2.92342879285128,-2.63361511917308,
-32.8250365996957));
#16910=CARTESIAN_POINT('Ctrl Pts',(-2.9996155108833,-2.54377589163596,-32.8309816911333));
#16911=CARTESIAN_POINT('Ctrl Pts',(-3.07477813895752,-2.45514426895587,
-32.8368468695809));
#16912=CARTESIAN_POINT('Ctrl Pts',(-3.14604172766473,-2.36314012029348,
-32.8427120480285));
#16913=CARTESIAN_POINT('Ctrl Pts',(-3.21309928916625,-2.26814504782197,
-32.8485772264761));
#16914=CARTESIAN_POINT('Ctrl Pts',(-3.2801479034551,-2.1731626501495,-32.8544416223573));
#16915=CARTESIAN_POINT('Ctrl Pts',(-3.34299136954786,-2.07519045824185,
-32.8603060182384));
#16916=CARTESIAN_POINT('Ctrl Pts',(-3.40136491724334,-1.97464065078844,
-32.8661704141195));
#16917=CARTESIAN_POINT('Ctrl Pts',(-3.45974463353904,-1.87408021777623,
-32.8720354297182));
#16918=CARTESIAN_POINT('Ctrl Pts',(-3.51365328594307,-1.77094198339011,
-32.8779004453169));
#16919=CARTESIAN_POINT('Ctrl Pts',(-3.56287146345836,-1.66566381208037,
-32.8837654609156));
#16920=CARTESIAN_POINT('Ctrl Pts',(-3.6132665685438,-1.55786818099041,-32.8897707234496));
#16921=CARTESIAN_POINT('Ctrl Pts',(-3.65874382689069,-1.44782937750596,
-32.8957759859836));
#16922=CARTESIAN_POINT('Ctrl Pts',(-3.6991199637996,-1.33603910624624,-32.9017812485177));
#16923=CARTESIAN_POINT('Ctrl Pts',(-3.73861081307489,-1.22669994973603,
-32.9076548395975));
#16924=CARTESIAN_POINT('Ctrl Pts',(-3.77322186797733,-1.1156857559224,-32.9135284306774));
#16925=CARTESIAN_POINT('Ctrl Pts',(-3.80283252423422,-1.00347087283408,
-32.9194020217573));
#16926=CARTESIAN_POINT('Ctrl Pts',(-3.83343887753063,-0.88748261755462,
-32.9254731200184));
#16927=CARTESIAN_POINT('Ctrl Pts',(-3.85870252048206,-0.77021197615689,
-32.9315442182795));
#16928=CARTESIAN_POINT('Ctrl Pts',(-3.87854805071123,-0.652191703660906,
-32.9376153165405));
#16929=CARTESIAN_POINT('Ctrl Pts',(-3.8983935809404,-0.534171431164921,
-32.9436864148016));
#16930=CARTESIAN_POINT('Ctrl Pts',(-3.91282100477258,-0.415402010263376,
-32.9497575130626));
#16931=CARTESIAN_POINT('Ctrl Pts',(-3.92181403309018,-0.296418099745836,
-32.9558286113237));
#16932=CARTESIAN_POINT('Ctrl Pts',(-3.93053068511083,-0.181090836513672,
-32.9617131308711));
#16933=CARTESIAN_POINT('Ctrl Pts',(-3.93416982632619,-0.0651953659832383,
-32.9675976504184));
#16934=CARTESIAN_POINT('Ctrl Pts',(-3.93267210647658,0.0507848692139364,
-32.9734821699658));
#16935=CARTESIAN_POINT('Ctrl Pts',(-3.93117626367143,0.166619750085193,
-32.9793593146326));
#16936=CARTESIAN_POINT('Ctrl Pts',(-3.92455636942314,0.282538776546033,
-32.9852364592995));
#16937=CARTESIAN_POINT('Ctrl Pts',(-3.91280488118397,0.398053968430045,
-32.9911136039664));
#16938=CARTESIAN_POINT('Ctrl Pts',(-3.90106501715643,0.513454896230318,
-32.9969849351421));
#16939=CARTESIAN_POINT('Ctrl Pts',(-3.88420369839419,0.628452377167216,
-33.0028562663178));
#16940=CARTESIAN_POINT('Ctrl Pts',(-3.86226541634821,0.74255966338108,-33.0087275974935));
#16941=CARTESIAN_POINT('Ctrl Pts',(-3.84005126678914,0.858101815515895,
-33.0146727589502));
#16942=CARTESIAN_POINT('Ctrl Pts',(-3.81263159476208,0.972730802578463,
-33.020617920407));
#16943=CARTESIAN_POINT('Ctrl Pts',(-3.78010674175324,1.08594752219051,-33.0265630818638));
#16944=CARTESIAN_POINT('Ctrl Pts',(-3.74802053654203,1.19763733975325,-33.0324280636506));
#16945=CARTESIAN_POINT('Ctrl Pts',(-3.71096613123705,1.30795234443374,-33.0382930454374));
#16946=CARTESIAN_POINT('Ctrl Pts',(-3.66909086963857,1.41642549762947,-33.0441580272242));
#16947=CARTESIAN_POINT('Ctrl Pts',(-3.6272212107881,1.52488413753693,-33.0500222242992));
#16948=CARTESIAN_POINT('Ctrl Pts',(-3.58053212654854,1.63150103247949,-33.0558864213741));
#16949=CARTESIAN_POINT('Ctrl Pts',(-3.5292198152104,1.73582732318807,-33.0617506184491));
#16950=CARTESIAN_POINT('Ctrl Pts',(-3.47790209812912,1.84016460465336,-33.0676154333162));
#16951=CARTESIAN_POINT('Ctrl Pts',(-3.4219603672357,1.9422104331075,-33.0734802481833));
#16952=CARTESIAN_POINT('Ctrl Pts',(-3.36163734700523,2.04153945521992,-33.0793450630504));
#16953=CARTESIAN_POINT('Ctrl Pts',(-3.29986694772536,2.14325175895605,-33.0853505971675));
#16954=CARTESIAN_POINT('Ctrl Pts',(-3.23350255939668,2.24211482894883,-33.0913561312846));
#16955=CARTESIAN_POINT('Ctrl Pts',(-3.1628518234218,2.33770343351704,-33.0973616654018));
#16956=CARTESIAN_POINT('Ctrl Pts',(-3.09375569744753,2.43118869126863,-33.1032350527936));
#16957=CARTESIAN_POINT('Ctrl Pts',(-3.02056021980915,2.52154181398208,-33.1091084401855));
#16958=CARTESIAN_POINT('Ctrl Pts',(-2.94359326470448,2.60839945023504,-33.1149818275774));
#16959=CARTESIAN_POINT('Ctrl Pts',(-2.8640287631433,2.698188432089,-33.1210534350571));
#16960=CARTESIAN_POINT('Ctrl Pts',(-2.78043405929133,2.78424147427113,-33.1271250425369));
#16961=CARTESIAN_POINT('Ctrl Pts',(-2.69321084009126,2.86620033682486,-33.1331966500167));
#16962=CARTESIAN_POINT('Ctrl Pts',(-2.60598762089118,2.94815919937859,-33.1392682574965));
#16963=CARTESIAN_POINT('Ctrl Pts',(-2.51513629182969,3.02602361977077,-33.1453398649762));
#16964=CARTESIAN_POINT('Ctrl Pts',(-2.42109291475038,3.09948352119277,-33.151411472456));
#16965=CARTESIAN_POINT('Ctrl Pts',(-2.32994515332462,3.17068157657018,-33.1572961338455));
#16966=CARTESIAN_POINT('Ctrl Pts',(-2.23550924406806,3.23796877116968,-33.163180795235));
#16967=CARTESIAN_POINT('Ctrl Pts',(-2.13815464494391,3.30102767548301,-33.1690654566246));
#16968=CARTESIAN_POINT('Ctrl Pts',(-2.04092202264943,3.36400757248391,-33.1749427450461));
#16969=CARTESIAN_POINT('Ctrl Pts',(-1.9407783259589,3.42276949413999,-33.1808200334676));
#16970=CARTESIAN_POINT('Ctrl Pts',(-1.83812551117062,3.47703661257453,-33.1866973218892));
#16971=CARTESIAN_POINT('Ctrl Pts',(-1.73557420493279,3.53125006880272,-33.1925687985361));
#16972=CARTESIAN_POINT('Ctrl Pts',(-1.63051907802622,3.58097737262402,-33.198440275183));
#16973=CARTESIAN_POINT('Ctrl Pts',(-1.52338990881487,3.62598568470989,-33.2043117518299));
#16974=CARTESIAN_POINT('Ctrl Pts',(-1.4149172922143,3.67155842103063,-33.2102568594031));
#16975=CARTESIAN_POINT('Ctrl Pts',(-1.30431861513318,3.71229276106702,-33.2162019669764));
#16976=CARTESIAN_POINT('Ctrl Pts',(-1.19206485361884,3.74799551557452,-33.2221470745497));
#16977=CARTESIAN_POINT('Ctrl Pts',(-1.0813211949525,3.78321797587596,-33.2280122050803));
#16978=CARTESIAN_POINT('Ctrl Pts',(-0.968967114970975,3.81354327603183,
-33.2338773356108));
#16979=CARTESIAN_POINT('Ctrl Pts',(-0.855473010787105,3.83883510036767,
-33.2397424661414));
#16980=CARTESIAN_POINT('Ctrl Pts',(-0.741994072734053,3.86412354497626,
-33.245606812919));
#16981=CARTESIAN_POINT('Ctrl Pts',(-0.627375814775837,3.88437976206234,
-33.2514711596967));
#16982=CARTESIAN_POINT('Ctrl Pts',(-0.512100590272377,3.89951817349819,
-33.2573355064743));
#16983=CARTESIAN_POINT('Ctrl Pts',(-0.396813206327458,3.91465818176136,
-33.263200471834));
#16984=CARTESIAN_POINT('Ctrl Pts',(-0.280869125837155,3.92467925766785,
-33.2690654371936));
#16985=CARTESIAN_POINT('Ctrl Pts',(-0.164756934862439,3.92954757604673,
-33.2749304025533));
#16986=CARTESIAN_POINT('Ctrl Pts',(-0.045865909800695,3.93453240457794,
-33.2809357301396));
#16987=CARTESIAN_POINT('Ctrl Pts',(0.0732009217401429,3.93411467667804,
-33.2869410577258));
#16988=CARTESIAN_POINT('Ctrl Pts',(0.19191917622264,3.92831465514131,-33.2929463853121));
#16989=CARTESIAN_POINT('Ctrl Pts',(0.308032114969537,3.9226419172093,-33.2988199237769));
#16990=CARTESIAN_POINT('Ctrl Pts',(0.423811209757561,3.91182078482897,-33.3046934622417));
#16991=CARTESIAN_POINT('Ctrl Pts',(0.538772264323822,3.8959226695605,-33.3105670007065));
#16992=CARTESIAN_POINT('Ctrl Pts',(0.657602523920222,3.87948947684516,-33.3166382228535));
#16993=CARTESIAN_POINT('Ctrl Pts',(0.775558231229076,3.85763162002537,-33.3227094450005));
#16994=CARTESIAN_POINT('Ctrl Pts',(0.892118655377857,3.83048473495546,-33.3287806671475));
#16995=CARTESIAN_POINT('Ctrl Pts',(1.00867907952663,3.80333784988555,-33.3348518892945));
#16996=CARTESIAN_POINT('Ctrl Pts',(1.12384377742956,3.77090212835676,-33.3409231114414));
#16997=CARTESIAN_POINT('Ctrl Pts',(1.2371130332575,3.7333684981454,-33.3469943335884));
#16998=CARTESIAN_POINT('Ctrl Pts',(1.3469010622397,3.69698842968524,-33.3528789622828));
#16999=CARTESIAN_POINT('Ctrl Pts',(1.45525749307561,3.6557036013568,-33.3587635909771));
#17000=CARTESIAN_POINT('Ctrl Pts',(1.56171331480212,3.60964548430587,-33.3646482196714));
#17001=CARTESIAN_POINT('Ctrl Pts',(1.66803575248797,3.56364507586739,-33.3705254752081));
#17002=CARTESIAN_POINT('Ctrl Pts',(1.77246194313386,3.51288343575072,-33.3764027307448));
#17003=CARTESIAN_POINT('Ctrl Pts',(1.8745386466048,3.45754159228563,-33.3822799862815));
#17004=CARTESIAN_POINT('Ctrl Pts',(1.97651440811705,3.40225447545147,-33.3881514298978));
#17005=CARTESIAN_POINT('Ctrl Pts',(2.07614494481964,3.34239636046427,-33.394022873514));
#17006=CARTESIAN_POINT('Ctrl Pts',(2.17299819887174,3.27819581899864,-33.3998943171302));
#17007=CARTESIAN_POINT('Ctrl Pts',(2.27106679079648,3.21318967373321,-33.4058394370298));
#17008=CARTESIAN_POINT('Ctrl Pts',(2.36628752689966,3.14373154093288,-33.4117845569294));
#17009=CARTESIAN_POINT('Ctrl Pts',(2.45823849561404,3.07010626830428,-33.417729676829));
#17010=CARTESIAN_POINT('Ctrl Pts',(2.54895178535895,2.99747200700299,-33.4235947741908));
#17011=CARTESIAN_POINT('Ctrl Pts',(2.63648246611203,2.92078236986249,-33.4294598715526));
#17012=CARTESIAN_POINT('Ctrl Pts',(2.72045628843409,2.84035324963628,-33.4353249689144));
#17013=CARTESIAN_POINT('Ctrl Pts',(2.80441888946648,2.75993487702679,-33.4411892825325));
#17014=CARTESIAN_POINT('Ctrl Pts',(2.8848252804178,2.67577829955866,-33.4470535961506));
#17015=CARTESIAN_POINT('Ctrl Pts',(2.96133680772466,2.58823749126991,-33.4529179097686));
#17016=CARTESIAN_POINT('Ctrl Pts',(3.03785640627714,2.50068744825025,-33.4587828420166));
#17017=CARTESIAN_POINT('Ctrl Pts',(3.1104800537526,2.4097527743698,-33.4646477742645));
#17018=CARTESIAN_POINT('Ctrl Pts',(3.17890871093214,2.31582132461892,-33.4705127065124));
#17019=CARTESIAN_POINT('Ctrl Pts',(3.2489759619245,2.21964059074156,-33.4765180805298));
#17020=CARTESIAN_POINT('Ctrl Pts',(3.31464448561763,2.12031809477642,-33.4825234545472));
#17021=CARTESIAN_POINT('Ctrl Pts',(3.37564039807835,2.0183014895851,-33.4885288285645));
#17022=CARTESIAN_POINT('Ctrl Pts',(3.43529693959773,1.91852500296919,-33.4944023343447));
#17023=CARTESIAN_POINT('Ctrl Pts',(3.49048381712388,1.81617189948764,-33.5002758401249));
#17024=CARTESIAN_POINT('Ctrl Pts',(3.5409920065088,1.71168472851772,-33.5061493459051));
#17025=CARTESIAN_POINT('Ctrl Pts',(3.59320116278114,1.60367873772582,-33.5122206540411));
#17026=CARTESIAN_POINT('Ctrl Pts',(3.64041075589718,1.49339285329059,-33.518291962177));
#17027=CARTESIAN_POINT('Ctrl Pts',(3.68244494504431,1.38133566764838,-33.524363270313));
#17028=CARTESIAN_POINT('Ctrl Pts',(3.72447913419144,1.26927848200616,-33.5304345784489));
#17029=CARTESIAN_POINT('Ctrl Pts',(3.761337833314,1.15545047029401,-33.5365058865849));
#17030=CARTESIAN_POINT('Ctrl Pts',(3.79290287308455,1.04037339227171,-33.5425771947208));
#17031=CARTESIAN_POINT('Ctrl Pts',(3.83119867671295,0.900757880486982,-33.5499431168243));
#17032=CARTESIAN_POINT('Ctrl Pts',(3.86180261359598,0.758949987624212,-33.5573090389277));
#17033=CARTESIAN_POINT('Ctrl Pts',(3.88450769868466,0.615701988675996,-33.5646749610311));
#17034=CARTESIAN_POINT('Ctrl Pts',(3.90687601725961,0.474578673648444,-33.5719316302559));
#17035=CARTESIAN_POINT('Ctrl Pts',(3.92157806086247,0.332057550685683,-33.5791882994806));
#17036=CARTESIAN_POINT('Ctrl Pts',(3.92846204140117,0.188878239271026,-33.5864449687053));
#17037=CARTESIAN_POINT('Ctrl Pts',(3.93143176781017,0.127111158446251,-33.5895754717793));
#17038=CARTESIAN_POINT('Ctrl Pts',(3.93294711680607,0.0652218550975597,
-33.5927059748534));
#17039=CARTESIAN_POINT('Ctrl Pts',(3.93299863980535,0.00327097680709954,
-33.5958364779274));
#17040=CARTESIAN_POINT('',(3.93299901959195,-0.00277702875856491,-34.8458364780034));
#17041=CARTESIAN_POINT('Ctrl Pts',(3.93299863980597,0.00327097606317273,
-33.595836477965));
#17042=CARTESIAN_POINT('Ctrl Pts',(3.93309624041199,-0.114083306980526,
-33.6017666270437));
#17043=CARTESIAN_POINT('Ctrl Pts',(3.9279367460832,-0.231548868260059,-33.6076967761224));
#17044=CARTESIAN_POINT('Ctrl Pts',(3.91751920417218,-0.348614808839455,
-33.613626925201));
#17045=CARTESIAN_POINT('Ctrl Pts',(3.90730826068607,-0.463359123152169,
-33.6194394688532));
#17046=CARTESIAN_POINT('Ctrl Pts',(3.89204593702237,-0.577719083384085,
-33.6252520125054));
#17047=CARTESIAN_POINT('Ctrl Pts',(3.87178389998692,-0.691215184875232,
-33.6310645561577));
#17048=CARTESIAN_POINT('Ctrl Pts',(3.85152588368495,-0.804688764564849,
-33.6368759463874));
#17049=CARTESIAN_POINT('Ctrl Pts',(3.82627019998669,-0.917298413337728,
-33.6426873366171));
#17050=CARTESIAN_POINT('Ctrl Pts',(3.79611999416202,-1.02857279271978,-33.6484987268469));
#17051=CARTESIAN_POINT('Ctrl Pts',(3.76596821706489,-1.1398529711457,-33.6543104199361));
#17052=CARTESIAN_POINT('Ctrl Pts',(3.73092152122106,-1.24979733697056,-33.6601221130254));
#17053=CARTESIAN_POINT('Ctrl Pts',(3.69113327348597,-1.35794851057202,-33.6659338061147));
#17054=CARTESIAN_POINT('Ctrl Pts',(3.64992675137281,-1.46995479333782,-33.6719526602595));
#17055=CARTESIAN_POINT('Ctrl Pts',(3.60363449834118,-1.58003720159471,-33.6779715144044));
#17056=CARTESIAN_POINT('Ctrl Pts',(3.55248123063851,-1.68771031458633,-33.6839903685493));
#17057=CARTESIAN_POINT('Ctrl Pts',(3.50301921804101,-1.79182348487604,-33.6898102243064));
#17058=CARTESIAN_POINT('Ctrl Pts',(3.44901280294868,-1.89368381053235,-33.6956300800636));
#17059=CARTESIAN_POINT('Ctrl Pts',(3.39071134500875,-1.99287871553413,-33.7014499358207));
#17060=CARTESIAN_POINT('Ctrl Pts',(3.32941963354287,-2.09716127914546,-33.7075682891595));
#17061=CARTESIAN_POINT('Ctrl Pts',(3.26338090755395,-2.19849730185159,-33.7136866424982));
#17062=CARTESIAN_POINT('Ctrl Pts',(3.19293463525649,-2.29644451598106,-33.719804995837));
#17063=CARTESIAN_POINT('Ctrl Pts',(3.12248836295904,-2.39439173011053,-33.7259233491757));
#17064=CARTESIAN_POINT('Ctrl Pts',(3.04763493272809,-2.48894976633921,-33.7320417025144));
#17065=CARTESIAN_POINT('Ctrl Pts',(2.96875942677061,-2.57972023017238,-33.7381600558532));
#17066=CARTESIAN_POINT('Ctrl Pts',(2.89289700477522,-2.66702321667546,-33.74404468502));
#17067=CARTESIAN_POINT('Ctrl Pts',(2.81305973462294,-2.75111579554493,-33.7499293141867));
#17068=CARTESIAN_POINT('Ctrl Pts',(2.72954960188932,-2.83161578799558,-33.7558139433535));
#17069=CARTESIAN_POINT('Ctrl Pts',(2.64614410503506,-2.91201491618913,-33.7616911992431));
#17070=CARTESIAN_POINT('Ctrl Pts',(2.55907519218587,-2.98883012786828,-33.7675684551328));
#17071=CARTESIAN_POINT('Ctrl Pts',(2.46868450730728,-3.06171288715663,-33.7734457110225));
#17072=CARTESIAN_POINT('Ctrl Pts',(2.37838321010869,-3.13452357241685,-33.7793171548723));
#17073=CARTESIAN_POINT('Ctrl Pts',(2.28476699406984,-3.20340928468332,-33.785188598722));
#17074=CARTESIAN_POINT('Ctrl Pts',(2.1882132186511,-3.26805934917354,-33.7910600425718));
#17075=CARTESIAN_POINT('Ctrl Pts',(2.09044786935521,-3.33352065412488,-33.797005162339));
#17076=CARTESIAN_POINT('Ctrl Pts',(1.98967103841307,-3.39463898224683,-33.8029502821063));
#17077=CARTESIAN_POINT('Ctrl Pts',(1.88630811055672,-3.45113469920372,-33.8088954018735));
#17078=CARTESIAN_POINT('Ctrl Pts',(1.78433646783499,-3.50686997281016,-33.8147604991711));
#17079=CARTESIAN_POINT('Ctrl Pts',(1.67984829521716,-3.55810611873482,-33.8206255964687));
#17080=CARTESIAN_POINT('Ctrl Pts',(1.57327926792445,-3.6046194452562,-33.8264906937663));
#17081=CARTESIAN_POINT('Ctrl Pts',(1.4667244833205,-3.65112655538572,-33.8323550072081));
#17082=CARTESIAN_POINT('Ctrl Pts',(1.35808977397541,-3.69291193697634,-33.8382193206498));
#17083=CARTESIAN_POINT('Ctrl Pts',(1.24783224668237,-3.72979941607315,-33.8440836340916));
#17084=CARTESIAN_POINT('Ctrl Pts',(1.13756309037341,-3.76669078574409,-33.8499485660507));
#17085=CARTESIAN_POINT('Ctrl Pts',(1.0256711658779,-3.79868309549359,-33.8558134980098));
#17086=CARTESIAN_POINT('Ctrl Pts',(0.912629587461413,-3.8256497795917,-33.8616784299689));
#17087=CARTESIAN_POINT('Ctrl Pts',(0.79688110965979,-3.85326220927852,-33.867683803887));
#17088=CARTESIAN_POINT('Ctrl Pts',(0.679927657319526,-3.87560514942635,
-33.873689177805));
#17089=CARTESIAN_POINT('Ctrl Pts',(0.562287838856864,-3.89259828215983,
-33.8796945517231));
#17090=CARTESIAN_POINT('Ctrl Pts',(0.447231208518604,-3.90921827203024,
-33.8855680569355));
#17091=CARTESIAN_POINT('Ctrl Pts',(0.331518464586647,-3.92072099962597,
-33.891441562148));
#17092=CARTESIAN_POINT('Ctrl Pts',(0.215638522254376,-3.92708403624368,
-33.8973150673604));
#17093=CARTESIAN_POINT('Ctrl Pts',(0.0958560709140378,-3.93366136195422,
-33.9033863756313));
#17094=CARTESIAN_POINT('Ctrl Pts',(-0.0241045538234508,-3.93474670906188,
-33.9094576839021));
#17095=CARTESIAN_POINT('Ctrl Pts',(-0.143706271518569,-3.93037371092448,
-33.915528992173));
#17096=CARTESIAN_POINT('Ctrl Pts',(-0.263307989213692,-3.92600071278707,
-33.9216003004438));
#17097=CARTESIAN_POINT('Ctrl Pts',(-0.382550328244256,-3.91616947300749,
-33.9276716087147));
#17098=CARTESIAN_POINT('Ctrl Pts',(-0.500906271424316,-3.90097191828495,
-33.9337429169855));
#17099=CARTESIAN_POINT('Ctrl Pts',(-0.615622924103891,-3.88624166849908,
-33.9396275404654));
#17100=CARTESIAN_POINT('Ctrl Pts',(-0.729871617218782,-3.8664234877586,
-33.9455121639452));
#17101=CARTESIAN_POINT('Ctrl Pts',(-0.843166860449312,-3.84155679971545,
-33.9513967874251));
#17102=CARTESIAN_POINT('Ctrl Pts',(-0.956320146799781,-3.81672126918036,
-33.9572740375787));
#17103=CARTESIAN_POINT('Ctrl Pts',(-1.06852196100831,-3.78684990002925,
-33.9631512877323));
#17104=CARTESIAN_POINT('Ctrl Pts',(-1.17929282290527,-3.7520337735479,-33.9690285378859));
#17105=CARTESIAN_POINT('Ctrl Pts',(-1.2899541422015,-3.71725207714119,-33.9748999759581));
#17106=CARTESIAN_POINT('Ctrl Pts',(-1.3991869340485,-3.67753547372865,-33.9807714140303));
#17107=CARTESIAN_POINT('Ctrl Pts',(-1.50652342501249,-3.63302575959607,
-33.9866428521026));
#17108=CARTESIAN_POINT('Ctrl Pts',(-1.61520693952953,-3.58795746903961,
-33.9925879740199));
#17109=CARTESIAN_POINT('Ctrl Pts',(-1.72194581173416,-3.53797502735493,
-33.9985330959372));
#17110=CARTESIAN_POINT('Ctrl Pts',(-1.82627147174328,-3.48327740949478,
-34.0044782178545));
#17111=CARTESIAN_POINT('Ctrl Pts',(-1.92919274833091,-3.42931610547832,
-34.0103433093108));
#17112=CARTESIAN_POINT('Ctrl Pts',(-2.02976501427928,-3.37076599738194,
-34.0162084007672));
#17113=CARTESIAN_POINT('Ctrl Pts',(-2.12756055287515,-3.30786564023534,
-34.0220734922235));
#17114=CARTESIAN_POINT('Ctrl Pts',(-2.22534302110393,-3.24497368971721,
-34.0279377998108));
#17115=CARTESIAN_POINT('Ctrl Pts',(-2.32034915424173,-3.17773286889969,
-34.0338021073981));
#17116=CARTESIAN_POINT('Ctrl Pts',(-2.41217889844789,-3.10642591443651,
-34.0396664149854));
#17117=CARTESIAN_POINT('Ctrl Pts',(-2.50401832797392,-3.03511143920031,
-34.0455313410836));
#17118=CARTESIAN_POINT('Ctrl Pts',(-2.59268037774681,-2.95973023001703,
-34.0513962671817));
#17119=CARTESIAN_POINT('Ctrl Pts',(-2.67779740387659,-2.88060585012803,
-34.0572611932799));
#17120=CARTESIAN_POINT('Ctrl Pts',(-2.76495285204481,-2.7995865628735,-34.0632665753497));
#17121=CARTESIAN_POINT('Ctrl Pts',(-2.8483909820269,-2.71464283968997,-34.0692719574195));
#17122=CARTESIAN_POINT('Ctrl Pts',(-2.92775741230827,-2.6261617495261,-34.0752773394894));
#17123=CARTESIAN_POINT('Ctrl Pts',(-3.0053808964421,-2.53962377025539,-34.081150838879));
#17124=CARTESIAN_POINT('Ctrl Pts',(-3.07910945607348,-2.44970254953049,
-34.0870243382687));
#17125=CARTESIAN_POINT('Ctrl Pts',(-3.14865335206111,-2.35679253829317,
-34.0928978376583));
#17126=CARTESIAN_POINT('Ctrl Pts',(-3.22053954046738,-2.26075324573149,
-34.0989691610682));
#17127=CARTESIAN_POINT('Ctrl Pts',(-3.28795393741286,-2.16152068481002,
-34.1050404844782));
#17128=CARTESIAN_POINT('Ctrl Pts',(-3.35062675256515,-2.05956047859604,
-34.1111118078881));
#17129=CARTESIAN_POINT('Ctrl Pts',(-3.41329956771743,-1.95760027238206,
-34.1171831312981));
#17130=CARTESIAN_POINT('Ctrl Pts',(-3.47123062580845,-1.85291287082147,
-34.123254454708));
#17131=CARTESIAN_POINT('Ctrl Pts',(-3.52420422986645,-1.74598784250962,
-34.1293257781179));
#17132=CARTESIAN_POINT('Ctrl Pts',(-3.57554882409555,-1.64235090314647,
-34.1352104001379));
#17133=CARTESIAN_POINT('Ctrl Pts',(-3.62239966877812,-1.53628245983126,
-34.1410950221579));
#17134=CARTESIAN_POINT('Ctrl Pts',(-3.66452039789657,-1.42820840685104,
-34.1469796441779));
#17135=CARTESIAN_POINT('Ctrl Pts',(-3.70658835021612,-1.32026976944123,
-34.1528568928328));
#17136=CARTESIAN_POINT('Ctrl Pts',(-3.74393782675065,-1.2103309004938,-34.1587341414877));
#17137=CARTESIAN_POINT('Ctrl Pts',(-3.77637878444347,-1.09884133358973,
-34.1646113901426));
#17138=CARTESIAN_POINT('Ctrl Pts',(-3.80878766068298,-0.987462020746884,
-34.1704828266793));
#17139=CARTESIAN_POINT('Ctrl Pts',(-3.83629756025312,-0.874535453351869,
-34.1763542632161));
#17140=CARTESIAN_POINT('Ctrl Pts',(-3.8587671369953,-0.760529540810288,
-34.1822256997529));
#17141=CARTESIAN_POINT('Ctrl Pts',(-3.88151870468208,-0.645092865449426,
-34.1881708222319));
#17142=CARTESIAN_POINT('Ctrl Pts',(-3.89910241080427,-0.528549965408921,
-34.194115944711));
#17143=CARTESIAN_POINT('Ctrl Pts',(-3.91142405295958,-0.411401115615005,
-34.20006106719));
#17144=CARTESIAN_POINT('Ctrl Pts',(-3.92357982241177,-0.295829311813609,
-34.2059261570303));
#17145=CARTESIAN_POINT('Ctrl Pts',(-3.93061429748689,-0.179668194380369,
-34.2117912468706));
#17146=CARTESIAN_POINT('Ctrl Pts',(-3.932488866005,-0.0634059835242513,
-34.2176563367108));
#17147=CARTESIAN_POINT('Ctrl Pts',(-3.93436318397833,0.0528406883477371,
-34.2235206426546));
#17148=CARTESIAN_POINT('Ctrl Pts',(-3.93107896035696,0.169188015656239,
-34.2293849485984));
#17149=CARTESIAN_POINT('Ctrl Pts',(-3.92264968935785,0.285146303817477,
-34.2352492545422));
#17150=CARTESIAN_POINT('Ctrl Pts',(-3.91421952935678,0.401116821641947,
-34.2411141789712));
#17151=CARTESIAN_POINT('Ctrl Pts',(-3.90064327308692,0.516697808568232,
-34.2469791034002));
#17152=CARTESIAN_POINT('Ctrl Pts',(-3.88198636099284,0.631403906438346,
-34.2528440278292));
#17153=CARTESIAN_POINT('Ctrl Pts',(-3.86288263202675,0.748857115919984,
-34.2588494121143));
#17154=CARTESIAN_POINT('Ctrl Pts',(-3.83845186018606,0.865392548235749,
-34.2648547963994));
#17155=CARTESIAN_POINT('Ctrl Pts',(-3.80881969032344,0.980500671394169,
-34.2708601806845));
#17156=CARTESIAN_POINT('Ctrl Pts',(-3.77983828423253,1.09308085965185,-34.2767336783563));
#17157=CARTESIAN_POINT('Ctrl Pts',(-3.74588176504571,1.20429540379539,-34.2826071760281));
#17158=CARTESIAN_POINT('Ctrl Pts',(-3.70711776117573,1.31368447687236,-34.2884806736999));
#17159=CARTESIAN_POINT('Ctrl Pts',(-3.66704811623616,1.42675796982645,-34.2945520012916));
#17160=CARTESIAN_POINT('Ctrl Pts',(-3.62184161023935,1.53788040401586,-34.3006233288834));
#17161=CARTESIAN_POINT('Ctrl Pts',(-3.57173616386766,1.64656909230069,-34.3066946564751));
#17162=CARTESIAN_POINT('Ctrl Pts',(-3.52163071749597,1.75525778058552,-34.3127659840668));
#17163=CARTESIAN_POINT('Ctrl Pts',(-3.46662660803095,1.86151232763336,-34.3188373116586));
#17164=CARTESIAN_POINT('Ctrl Pts',(-3.40701167590485,1.96488178785596,-34.3249086392503));
#17165=CARTESIAN_POINT('Ctrl Pts',(-3.34923000101901,2.0650724671152,-34.3307932635302));
#17166=CARTESIAN_POINT('Ctrl Pts',(-3.28693325400658,2.16287145976681,-34.3366778878101));
#17167=CARTESIAN_POINT('Ctrl Pts',(-3.22034482403828,2.25784592350538,-34.3425625120899));
#17168=CARTESIAN_POINT('Ctrl Pts',(-3.15383982820297,2.35270138590931,-34.3484397630389));
#17169=CARTESIAN_POINT('Ctrl Pts',(-3.08305407872684,2.44473902442852,-34.354317013988));
#17170=CARTESIAN_POINT('Ctrl Pts',(-3.00825632123417,2.53355144130817,-34.360194264937));
#17171=CARTESIAN_POINT('Ctrl Pts',(-2.93353253218,2.62227603047723,-34.366065703799));
#17172=CARTESIAN_POINT('Ctrl Pts',(-2.8548048913113,2.70778143004122,-34.3719371426609));
#17173=CARTESIAN_POINT('Ctrl Pts',(-2.77238443652447,2.78969058071265,-34.3778085815229));
#17174=CARTESIAN_POINT('Ctrl Pts',(-2.68892965838043,2.87262763820562,-34.3837537031421));
#17175=CARTESIAN_POINT('Ctrl Pts',(-2.60168898803608,2.95187721300267,-34.3896988247613));
#17176=CARTESIAN_POINT('Ctrl Pts',(-2.51102653650519,3.02708353584217,-34.3956439463804));
#17177=CARTESIAN_POINT('Ctrl Pts',(-2.42158452441485,3.10127747967556,-34.4015090386073));
#17178=CARTESIAN_POINT('Ctrl Pts',(-2.32881262063838,3.17153609527604,-34.4073741308341));
#17179=CARTESIAN_POINT('Ctrl Pts',(-2.23309572594469,3.23755655993337,-34.4132392230609));
#17180=CARTESIAN_POINT('Ctrl Pts',(-2.13739162394793,3.3035682008632,-34.41910353141));
#17181=CARTESIAN_POINT('Ctrl Pts',(-2.0387436523071,3.36534258394099,-34.424967839759));
#17182=CARTESIAN_POINT('Ctrl Pts',(-1.93756682863945,3.42261943320552,-34.430832148108));
#17183=CARTESIAN_POINT('Ctrl Pts',(-1.83637933397904,3.47990232338753,-34.4366970749583));
#17184=CARTESIAN_POINT('Ctrl Pts',(-1.73266281497774,3.5326865341732,-34.4425620018086));
#17185=CARTESIAN_POINT('Ctrl Pts',(-1.62685748141285,3.58075742478753,-34.4484269286589));
#17186=CARTESIAN_POINT('Ctrl Pts',(-1.51851830623253,3.62997952412666,-34.4544323096359));
#17187=CARTESIAN_POINT('Ctrl Pts',(-1.40798940641783,3.67425948458499,-34.4604376906129));
#17188=CARTESIAN_POINT('Ctrl Pts',(-1.29576448807703,3.71341936649208,-34.4664430715899));
#17189=CARTESIAN_POINT('Ctrl Pts',(-1.18600407939974,3.75171927978607,-34.4723165717006));
#17190=CARTESIAN_POINT('Ctrl Pts',(-1.07462179118489,3.785121614066,-34.4781900718112));
#17191=CARTESIAN_POINT('Ctrl Pts',(-0.962093242570019,3.81351092729536,
-34.4840635719219));
#17192=CARTESIAN_POINT('Ctrl Pts',(-0.84577469765106,3.84285640137047,-34.4901348933321));
#17193=CARTESIAN_POINT('Ctrl Pts',(-0.728231793541606,3.86684512381164,
-34.4962062147422));
#17194=CARTESIAN_POINT('Ctrl Pts',(-0.609998144737329,3.88540747714021,
-34.5022775361523));
#17195=CARTESIAN_POINT('Ctrl Pts',(-0.491764495933051,3.90396983046877,
-34.5083488575625));
#17196=CARTESIAN_POINT('Ctrl Pts',(-0.372840585171041,3.91710582625685,
-34.5144201789726));
#17197=CARTESIAN_POINT('Ctrl Pts',(-0.253761288374039,3.92480498987182,
-34.5204915003827));
#17198=CARTESIAN_POINT('Ctrl Pts',(-0.138343775920815,3.93226739800079,
-34.5263761237665));
#17199=CARTESIAN_POINT('Ctrl Pts',(-0.0224133461781239,3.93464621096049,
-34.5322607471504));
#17200=CARTESIAN_POINT('Ctrl Pts',(0.0935459234724902,3.93188735344766,
-34.5381453705342));
#17201=CARTESIAN_POINT('Ctrl Pts',(0.209359897989908,3.92913195273972,-34.5440226205779));
#17202=CARTESIAN_POINT('Ctrl Pts',(0.325202232851273,3.92125169474425,-34.5498998706215));
#17203=CARTESIAN_POINT('Ctrl Pts',(0.440584878799683,3.9082443583498,-34.5557771206652));
#17204=CARTESIAN_POINT('Ctrl Pts',(0.555853421229502,3.89524988509294,-34.5616485586138));
#17205=CARTESIAN_POINT('Ctrl Pts',(0.670662772626538,3.87713846563527,-34.5675199965624));
#17206=CARTESIAN_POINT('Ctrl Pts',(0.7845266835988,3.85395989635614,-34.573391434511));
#17207=CARTESIAN_POINT('Ctrl Pts',(0.899819537466818,3.83049044604525,-34.5793365564695));
#17208=CARTESIAN_POINT('Ctrl Pts',(1.01414262987097,3.80182579812155,-34.585281678428));
#17209=CARTESIAN_POINT('Ctrl Pts',(1.12699800331394,3.76807172178641,-34.5912268003865));
#17210=CARTESIAN_POINT('Ctrl Pts',(1.23833416655996,3.73477202821916,-34.597091891686));
#17211=CARTESIAN_POINT('Ctrl Pts',(1.34824148095915,3.69651921823463,-34.6029569829856));
#17212=CARTESIAN_POINT('Ctrl Pts',(1.45625452603846,3.653465718382,-34.6088220742852));
#17213=CARTESIAN_POINT('Ctrl Pts',(1.56425313495665,3.61041797271638,-34.6146863817035));
#17214=CARTESIAN_POINT('Ctrl Pts',(1.67035759613018,3.56257096550373,-34.6205506891218));
#17215=CARTESIAN_POINT('Ctrl Pts',(1.77412119952072,3.51012577686486,-34.62641499654));
#17216=CARTESIAN_POINT('Ctrl Pts',(1.87789574668625,3.45767505691902,-34.6322799224571));
#17217=CARTESIAN_POINT('Ctrl Pts',(1.97932857822698,3.40062537699027,-34.6381448483742));
#17218=CARTESIAN_POINT('Ctrl Pts',(2.0779969952556,3.33922408468026,-34.6440097742912));
#17219=CARTESIAN_POINT('Ctrl Pts',(2.17902837578433,3.27635232170741,-34.6500151565599));
#17220=CARTESIAN_POINT('Ctrl Pts',(2.27716085985052,3.2089180970275,-34.6560205388285));
#17221=CARTESIAN_POINT('Ctrl Pts',(2.37197263114538,3.13723362807064,-34.6620259210972));
#17222=CARTESIAN_POINT('Ctrl Pts',(2.46470225867718,3.06712340847026,-34.6678994202772));
#17223=CARTESIAN_POINT('Ctrl Pts',(2.55425523969155,2.99294801054815,-34.6737729194572));
#17224=CARTESIAN_POINT('Ctrl Pts',(2.64027179851076,2.91503925016264,-34.6796464186373));
#17225=CARTESIAN_POINT('Ctrl Pts',(2.72918547089927,2.8345064540103,-34.6857177424502));
#17226=CARTESIAN_POINT('Ctrl Pts',(2.81431995726265,2.74998471745796,-34.6917890662632));
#17227=CARTESIAN_POINT('Ctrl Pts',(2.89532146271884,2.66187952911465,-34.6978603900762));
#17228=CARTESIAN_POINT('Ctrl Pts',(2.97632296817504,2.57377434077133,-34.7039317138891));
#17229=CARTESIAN_POINT('Ctrl Pts',(3.05319123470526,2.48208610879974,-34.7100030377021));
#17230=CARTESIAN_POINT('Ctrl Pts',(3.12562098824291,2.38725416281037,-34.716074361515));
#17231=CARTESIAN_POINT('Ctrl Pts',(3.19582130929989,2.29534120260056,-34.7219588062369));
#17232=CARTESIAN_POINT('Ctrl Pts',(3.26207947609405,2.20017791712166,-34.7278432509588));
#17233=CARTESIAN_POINT('Ctrl Pts',(3.32408079320321,2.10213602800997,-34.7337276956806));
#17234=CARTESIAN_POINT('Ctrl Pts',(3.38600596947555,2.00421453942891,-34.7396049139988));
#17235=CARTESIAN_POINT('Ctrl Pts',(3.44368447223116,1.9034218193157,-34.745482132317));
#17236=CARTESIAN_POINT('Ctrl Pts',(3.49684230894722,1.8001619000403,-34.7513593506352));
#17237=CARTESIAN_POINT('Ctrl Pts',(3.54994754095069,1.69700416623199,-34.7572307528894));
#17238=CARTESIAN_POINT('Ctrl Pts',(3.59854081669175,1.59138445150422,-34.7631021551436));
#17239=CARTESIAN_POINT('Ctrl Pts',(3.64239224160431,1.48373439614398,-34.7689735573978));
#17240=CARTESIAN_POINT('Ctrl Pts',(3.68621072592521,1.3761652060355,-34.7748405491348));
#17241=CARTESIAN_POINT('Ctrl Pts',(3.72529429092247,1.26656908823968,-34.7807075408718));
#17242=CARTESIAN_POINT('Ctrl Pts',(3.75945997591371,1.15540022914264,-34.7865745326088));
#17243=CARTESIAN_POINT('Ctrl Pts',(3.79361010033921,1.04428200126641,-34.792438852258));
#17244=CARTESIAN_POINT('Ctrl Pts',(3.82284667914449,0.931592848625983,-34.7983031719072));
#17245=CARTESIAN_POINT('Ctrl Pts',(3.84703590292379,0.81780423183997,-34.8041674915563));
#17246=CARTESIAN_POINT('Ctrl Pts',(3.87121878030779,0.70404546915547,-34.8100302726158));
#17247=CARTESIAN_POINT('Ctrl Pts',(3.89035685524024,0.589188218375522,-34.8158930536753));
#17248=CARTESIAN_POINT('Ctrl Pts',(3.90436711264923,0.473715578868916,-34.8217558347347));
#17249=CARTESIAN_POINT('Ctrl Pts',(3.91837958235046,0.358224705634153,-34.8276195415577));
#17250=CARTESIAN_POINT('Ctrl Pts',(3.92726256756757,0.242118657273612,-34.8334832483807));
#17251=CARTESIAN_POINT('Ctrl Pts',(3.93098480463834,0.125886717736397,-34.8393469552036));
#17252=CARTESIAN_POINT('Ctrl Pts',(3.93235797141511,0.0830077084910385,
-34.8415101294574));
#17253=CARTESIAN_POINT('Ctrl Pts',(3.93302930256552,0.0401115937067086,
-34.8436733037112));
#17254=CARTESIAN_POINT('Ctrl Pts',(3.93299901959249,-0.00277702799701734,
-34.845836477965));
#17255=CARTESIAN_POINT('',(3.93299981803602,0.00119638148616161,-36.0958364779956));
#17256=CARTESIAN_POINT('Ctrl Pts',(3.93299901959195,-0.00277702875855888,
-34.8458364780034));
#17257=CARTESIAN_POINT('Ctrl Pts',(3.93290411654262,-0.137184567338229,
-34.8526155936621));
#17258=CARTESIAN_POINT('Ctrl Pts',(3.92591531627658,-0.271321633643327,
-34.8593947093209));
#17259=CARTESIAN_POINT('Ctrl Pts',(3.91213938866519,-0.404542214922395,
-34.8661738249796));
#17260=CARTESIAN_POINT('Ctrl Pts',(3.89828763983609,-0.538496027892523,
-34.8729902521588));
#17261=CARTESIAN_POINT('Ctrl Pts',(3.87757395605432,-0.671523115649326,
-34.8798066793379));
#17262=CARTESIAN_POINT('Ctrl Pts',(3.85015627438072,-0.802985468639864,
-34.886623106517));
#17263=CARTESIAN_POINT('Ctrl Pts',(3.82257135468943,-0.935249694800271,
-34.8934811114555));
#17264=CARTESIAN_POINT('Ctrl Pts',(3.78820048763923,-1.06592991939294,-34.9003391163939));
#17265=CARTESIAN_POINT('Ctrl Pts',(3.74725292585918,-1.19439713229722,-34.9071971213324));
#17266=CARTESIAN_POINT('Ctrl Pts',(3.73837618129646,-1.22224666921866,-34.9086838217707));
#17267=CARTESIAN_POINT('Ctrl Pts',(3.72919054225404,-1.2499922865566,-34.9101705222091));
#17268=CARTESIAN_POINT('Ctrl Pts',(3.71969843258908,-1.27762771204853,-34.9116572226475));
#17269=CARTESIAN_POINT('Ctrl Pts',(3.68212698190591,-1.38701361914676,-34.9175418462109));
#17270=CARTESIAN_POINT('Ctrl Pts',(3.63966663410879,-1.49491469887107,-34.9234264697742));
#17271=CARTESIAN_POINT('Ctrl Pts',(3.59245394985051,-1.6008633977337,-34.9293110933376));
#17272=CARTESIAN_POINT('Ctrl Pts',(3.54530042233089,-1.70667934457029,-34.9351883435618));
#17273=CARTESIAN_POINT('Ctrl Pts',(3.49340656754212,-1.81054740353643,-34.9410655937859));
#17274=CARTESIAN_POINT('Ctrl Pts',(3.43695832899016,-1.9120163296335,-34.94694284401));
#17275=CARTESIAN_POINT('Ctrl Pts',(3.3805659128858,-2.01338491169939,-34.9528142821397));
#17276=CARTESIAN_POINT('Ctrl Pts',(3.31962827159465,-2.11235872321046,-34.9586857202694));
#17277=CARTESIAN_POINT('Ctrl Pts',(3.25437865893949,-2.20850821692815,-34.9645571583991));
#17278=CARTESIAN_POINT('Ctrl Pts',(3.18831019462166,-2.30586434114666,-34.97050228029));
#17279=CARTESIAN_POINT('Ctrl Pts',(3.11782096049279,-2.40032438035578,-34.9764474021809));
#17280=CARTESIAN_POINT('Ctrl Pts',(3.04320037395452,-2.49146954305347,-34.9823925240717));
#17281=CARTESIAN_POINT('Ctrl Pts',(2.9695842943429,-2.58138775282158,-34.9882576155528));
#17282=CARTESIAN_POINT('Ctrl Pts',(2.89194768309327,-2.66807946298302,-34.9941227070339));
#17283=CARTESIAN_POINT('Ctrl Pts',(2.81061048168482,-2.75117388040876,-34.9999877985149));
#17284=CARTESIAN_POINT('Ctrl Pts',(2.72928415115963,-2.83425719209574,-35.0058521061146));
#17285=CARTESIAN_POINT('Ctrl Pts',(2.64425850175204,-2.91374387342072,-35.0117164137142));
#17286=CARTESIAN_POINT('Ctrl Pts',(2.55589116707806,-2.98929913893748,-35.0175807213138));
#17287=CARTESIAN_POINT('Ctrl Pts',(2.46751451245395,-3.06486237313758,-35.0234456474118));
#17288=CARTESIAN_POINT('Ctrl Pts',(2.37579578451845,-3.13649309998798,-35.0293105735098));
#17289=CARTESIAN_POINT('Ctrl Pts',(2.28112606525489,-3.20389651431109,-35.0351754996078));
#17290=CARTESIAN_POINT('Ctrl Pts',(2.18418915251842,-3.27291413624138,-35.0411808816221));
#17291=CARTESIAN_POINT('Ctrl Pts',(2.08415847107028,-3.33749912379196,-35.0471862636364));
#17292=CARTESIAN_POINT('Ctrl Pts',(1.98148462704563,-3.39738247372618,-35.0531916456508));
#17293=CARTESIAN_POINT('Ctrl Pts',(1.88106557700872,-3.45595074075219,-35.059065145009));
#17294=CARTESIAN_POINT('Ctrl Pts',(1.77811865621738,-3.51002160514262,-35.0649386443673));
#17295=CARTESIAN_POINT('Ctrl Pts',(1.67308865941643,-3.55939086610787,-35.0708121437255));
#17296=CARTESIAN_POINT('Ctrl Pts',(1.56452117139397,-3.61042292182316,-35.0768834670679));
#17297=CARTESIAN_POINT('Ctrl Pts',(1.45372826226303,-3.65643089712131,-35.0829547904103));
#17298=CARTESIAN_POINT('Ctrl Pts',(1.34122041071177,-3.69724448879029,-35.0890261137527));
#17299=CARTESIAN_POINT('Ctrl Pts',(1.22871255916052,-3.73805808045926,-35.095097437095));
#17300=CARTESIAN_POINT('Ctrl Pts',(1.11449024124293,-3.77367720761152,-35.1011687604374));
#17301=CARTESIAN_POINT('Ctrl Pts',(0.999076475456495,-3.80398937908473,
-35.1072400837798));
#17302=CARTESIAN_POINT('Ctrl Pts',(0.887211810708316,-3.83336941773553,
-35.1131247072096));
#17303=CARTESIAN_POINT('Ctrl Pts',(0.773872255728606,-3.85785755251595,
-35.1190093306395));
#17304=CARTESIAN_POINT('Ctrl Pts',(0.659522634313266,-3.87730820219756,
-35.1248939540693));
#17305=CARTESIAN_POINT('Ctrl Pts',(0.54531629118452,-3.89673448051943,-35.130771204158));
#17306=CARTESIAN_POINT('Ctrl Pts',(0.430102800820088,-3.91113575917428,
-35.1366484542468));
#17307=CARTESIAN_POINT('Ctrl Pts',(0.314360794522347,-3.92041659659624,
-35.1425257043355));
#17308=CARTESIAN_POINT('Ctrl Pts',(0.198733247138435,-3.92968825606627,
-35.1483971423282));
#17309=CARTESIAN_POINT('Ctrl Pts',(0.0825786312786711,-3.93384951493226,
-35.1542685803209));
#17310=CARTESIAN_POINT('Ctrl Pts',(-0.033616248424685,-3.93285633450319,
-35.1601400183135));
#17311=CARTESIAN_POINT('Ctrl Pts',(-0.151269322456923,-3.93185069009917,
-35.1660851402551));
#17312=CARTESIAN_POINT('Ctrl Pts',(-0.268963256133996,-3.92556027080728,
-35.1720302621967));
#17313=CARTESIAN_POINT('Ctrl Pts',(-0.386189056632202,-3.91399374201563,
-35.1779753841383));
#17314=CARTESIAN_POINT('Ctrl Pts',(-0.501836815279357,-3.90258291671611,
-35.1838404754792));
#17315=CARTESIAN_POINT('Ctrl Pts',(-0.617028546701187,-3.88603720961323,
-35.1897055668201));
#17316=CARTESIAN_POINT('Ctrl Pts',(-0.731278279749321,-3.86441730116804,
-35.195570658161));
#17317=CARTESIAN_POINT('Ctrl Pts',(-0.845512743068666,-3.84280028227129,
-35.2014349656195));
#17318=CARTESIAN_POINT('Ctrl Pts',(-0.958805054411566,-3.81611048726668,
-35.207299273078));
#17319=CARTESIAN_POINT('Ctrl Pts',(-1.07067831106139,-3.78445992900212,
-35.2131635805365));
#17320=CARTESIAN_POINT('Ctrl Pts',(-1.18256336677593,-3.75280603261193,
-35.2190285064926));
#17321=CARTESIAN_POINT('Ctrl Pts',(-1.29302867453848,-3.71619044482881,
-35.2248934324488));
#17322=CARTESIAN_POINT('Ctrl Pts',(-1.40161205905972,-3.67477518168096,
-35.2307583584049));
#17323=CARTESIAN_POINT('Ctrl Pts',(-1.51279585412699,-3.6323680845842,-35.2367637406138));
#17324=CARTESIAN_POINT('Ctrl Pts',(-1.62200601345193,-3.58492865021709,
-35.2427691228228));
#17325=CARTESIAN_POINT('Ctrl Pts',(-1.72876883209973,-3.53268273768825,
-35.2487745050317));
#17326=CARTESIAN_POINT('Ctrl Pts',(-1.83318705391937,-3.48158418715631,
-35.2546480042475));
#17327=CARTESIAN_POINT('Ctrl Pts',(-1.93526398218542,-3.42588834359902,
-35.2605215034633));
#17328=CARTESIAN_POINT('Ctrl Pts',(-2.03458306425122,-3.36585215876487,
-35.2663950026791));
#17329=CARTESIAN_POINT('Ctrl Pts',(-2.13724729816016,-3.30379390374867,
-35.2724663263846));
#17330=CARTESIAN_POINT('Ctrl Pts',(-2.23696423412104,-3.23709804963224,
-35.2785376500901));
#17331=CARTESIAN_POINT('Ctrl Pts',(-2.33330911196602,-3.16609500615764,
-35.2846089737956));
#17332=CARTESIAN_POINT('Ctrl Pts',(-2.429653989811,-3.09509196268304,-35.2906802975011));
#17333=CARTESIAN_POINT('Ctrl Pts',(-2.52262647828011,-3.01978208118662,
-35.2967516212066));
#17334=CARTESIAN_POINT('Ctrl Pts',(-2.61184297721808,-2.94053826065171,
-35.3028229449121));
#17335=CARTESIAN_POINT('Ctrl Pts',(-2.6983159669777,-2.86373127805096,-35.3087075684836));
#17336=CARTESIAN_POINT('Ctrl Pts',(-2.78153553523632,-2.78298459042336,
-35.3145921920551));
#17337=CARTESIAN_POINT('Ctrl Pts',(-2.8611228090182,-2.69860431922054,-35.3204768156265));
#17338=CARTESIAN_POINT('Ctrl Pts',(-2.94061036119725,-2.61432977517098,
-35.3263540658572));
#17339=CARTESIAN_POINT('Ctrl Pts',(-3.0164743910532,-2.5264309993937,-35.3322313160878));
#17340=CARTESIAN_POINT('Ctrl Pts',(-3.08837009760411,-2.43525340369842,
-35.3381085663184));
#17341=CARTESIAN_POINT('Ctrl Pts',(-3.16019470547257,-2.34416597481887,
-35.3439800044531));
#17342=CARTESIAN_POINT('Ctrl Pts',(-3.228058543559,-2.2498064975538,-35.3498514425877));
#17343=CARTESIAN_POINT('Ctrl Pts',(-3.29165505796186,-2.15255568555011,
-35.3557228807224));
#17344=CARTESIAN_POINT('Ctrl Pts',(-3.35604967834843,-2.05408442214732,
-35.3616680026108));
#17345=CARTESIAN_POINT('Ctrl Pts',(-3.41606883728247,-1.95264906512456,
-35.3676131244992));
#17346=CARTESIAN_POINT('Ctrl Pts',(-3.47143754046562,-1.84867801486522,
-35.3735582463876));
#17347=CARTESIAN_POINT('Ctrl Pts',(-3.52606089647284,-1.7461065734866,-35.3794233378698));
#17348=CARTESIAN_POINT('Ctrl Pts',(-3.5761580415076,-1.64106766609363,-35.385288429352));
#17349=CARTESIAN_POINT('Ctrl Pts',(-3.62151003356077,-1.53399937314806,
-35.3911535208341));
#17350=CARTESIAN_POINT('Ctrl Pts',(-3.66685596421629,-1.42694539012519,
-35.3970178284334));
#17351=CARTESIAN_POINT('Ctrl Pts',(-3.70745784284173,-1.31786293958858,
-35.4028821360326));
#17352=CARTESIAN_POINT('Ctrl Pts',(-3.74314447536411,-1.20721101575124,
-35.4087464436319));
#17353=CARTESIAN_POINT('Ctrl Pts',(-3.77883487168513,-1.09654742167408,
-35.414611369728));
#17354=CARTESIAN_POINT('Ctrl Pts',(-3.80960886511949,-0.984314416649301,
-35.4204762958242));
#17355=CARTESIAN_POINT('Ctrl Pts',(-3.83534504090498,-0.870986462125324,
-35.4263412219204));
#17356=CARTESIAN_POINT('Ctrl Pts',(-3.86169755831827,-0.754944478269699,
-35.4323466039307));
#17357=CARTESIAN_POINT('Ctrl Pts',(-3.88276778282798,-0.637754873362918,
-35.4383519859411));
#17358=CARTESIAN_POINT('Ctrl Pts',(-3.89848103892302,-0.519937101155188,
-35.4443573679514));
#17359=CARTESIAN_POINT('Ctrl Pts',(-3.91384922022218,-0.404706694891866,
-35.4502308673043));
#17360=CARTESIAN_POINT('Ctrl Pts',(-3.92409331811529,-0.288875846870358,
-35.4561043666572));
#17361=CARTESIAN_POINT('Ctrl Pts',(-3.92919622061545,-0.172933686427134,
-35.46197786601));
#17362=CARTESIAN_POINT('Ctrl Pts',(-3.93447099280575,-0.0530865046378151,
-35.4680491893491));
#17363=CARTESIAN_POINT('Ctrl Pts',(-3.93425214587245,0.0668791348487649,
-35.4741205126882));
#17364=CARTESIAN_POINT('Ctrl Pts',(-3.92857915073386,0.186426544298882,
-35.4801918360273));
#17365=CARTESIAN_POINT('Ctrl Pts',(-3.92290615559527,0.305973953748994,
-35.4862631593664));
#17366=CARTESIAN_POINT('Ctrl Pts',(-3.91177912097813,0.425102662685562,
-35.4923344827054));
#17367=CARTESIAN_POINT('Ctrl Pts',(-3.89529569908986,0.543286679987709,
-35.4984058060445));
#17368=CARTESIAN_POINT('Ctrl Pts',(-3.87931916098607,0.657836405674736,
-35.5042904293542));
#17369=CARTESIAN_POINT('Ctrl Pts',(-3.85826008052821,0.771862885642022,
-35.5101750526639));
#17370=CARTESIAN_POINT('Ctrl Pts',(-3.83216315702605,0.884881086888037,
-35.5160596759736));
#17371=CARTESIAN_POINT('Ctrl Pts',(-3.8060989325574,0.997757678110552,-35.5219369259431));
#17372=CARTESIAN_POINT('Ctrl Pts',(-3.77500951150435,1.10962810597062,-35.5278141759126));
#17373=CARTESIAN_POINT('Ctrl Pts',(-3.73899118241851,1.22001390885376,-35.5336914258821));
#17374=CARTESIAN_POINT('Ctrl Pts',(-3.70300847236422,1.33029054966591,-35.5395628637566));
#17375=CARTESIAN_POINT('Ctrl Pts',(-3.66210667767968,1.43908509731551,-35.545434301631));
#17376=CARTESIAN_POINT('Ctrl Pts',(-3.61643267165019,1.54593134757695,-35.5513057395055));
#17377=CARTESIAN_POINT('Ctrl Pts',(-3.57018547577501,1.65411847399581,-35.5572508614918));
#17378=CARTESIAN_POINT('Ctrl Pts',(-3.51904556041223,1.7603076483752,-35.5631959834781));
#17379=CARTESIAN_POINT('Ctrl Pts',(-3.46321698282404,1.86403249163719,-35.5691411054644));
#17380=CARTESIAN_POINT('Ctrl Pts',(-3.40813994633525,1.96636103418532,-35.5750061966904));
#17381=CARTESIAN_POINT('Ctrl Pts',(-3.34849991474435,2.06629081748993,-35.5808712879163));
#17382=CARTESIAN_POINT('Ctrl Pts',(-3.28454007888917,2.16339674358883,-35.5867363791423));
#17383=CARTESIAN_POINT('Ctrl Pts',(-3.22058879139169,2.26048969128994,-35.5926006864873));
#17384=CARTESIAN_POINT('Ctrl Pts',(-3.15231907405219,2.35475918902425,-35.5984649938323));
#17385=CARTESIAN_POINT('Ctrl Pts',(-3.08001799598553,2.44580828038612,-35.6043293011773));
#17386=CARTESIAN_POINT('Ctrl Pts',(-3.00770929243914,2.53686697455085,-35.6101942270214));
#17387=CARTESIAN_POINT('Ctrl Pts',(-2.93136863868749,2.62470426506676,-35.6160591528656));
#17388=CARTESIAN_POINT('Ctrl Pts',(-2.85132357567657,2.70895604740848,-35.6219240787098));
#17389=CARTESIAN_POINT('Ctrl Pts',(-2.76936154867657,2.79522553860931,-35.627929461082));
#17390=CARTESIAN_POINT('Ctrl Pts',(-2.68351573030301,2.87773526593777,-35.6339348434543));
#17391=CARTESIAN_POINT('Ctrl Pts',(-2.59417701938815,2.95613507676466,-35.6399402258266));
#17392=CARTESIAN_POINT('Ctrl Pts',(-2.50680026193911,3.0328131616007,-35.6458137249352));
#17393=CARTESIAN_POINT('Ctrl Pts',(-2.41608280721572,3.10555977107576,-35.6516872240439));
#17394=CARTESIAN_POINT('Ctrl Pts',(-2.32242223273743,3.17408947146846,-35.6575607231526));
#17395=CARTESIAN_POINT('Ctrl Pts',(-2.22560708327707,3.24492731570493,-35.6636320471567));
#17396=CARTESIAN_POINT('Ctrl Pts',(-2.12564746892987,3.311258915708,-35.6697033711607));
#17397=CARTESIAN_POINT('Ctrl Pts',(-2.02301191846946,3.37281955902336,-35.6757746951648));
#17398=CARTESIAN_POINT('Ctrl Pts',(-1.92037636800905,3.43438020233871,-35.6818460191688));
#17399=CARTESIAN_POINT('Ctrl Pts',(-1.81506533326051,3.49116971860004,-35.6879173431729));
#17400=CARTESIAN_POINT('Ctrl Pts',(-1.70757069904962,3.54297774587241,-35.6939886671769));
#17401=CARTESIAN_POINT('Ctrl Pts',(-1.60338165575405,3.59319261321128,-35.6998732905738));
#17402=CARTESIAN_POINT('Ctrl Pts',(-1.49681010637261,3.63888755925846,-35.7057579139707));
#17403=CARTESIAN_POINT('Ctrl Pts',(-1.38828449001756,3.67983086225124,-35.7116425373676));
#17404=CARTESIAN_POINT('Ctrl Pts',(-1.27989485459223,3.72072286391448,-35.7175197874218));
#17405=CARTESIAN_POINT('Ctrl Pts',(-1.1695564034432,3.75687492005202,-35.723397037476));
#17406=CARTESIAN_POINT('Ctrl Pts',(-1.05772070994583,3.7881018861366,-35.7292742875302));
#17407=CARTESIAN_POINT('Ctrl Pts',(-0.945995612383948,3.81929797142259,
-35.7351457254868));
#17408=CARTESIAN_POINT('Ctrl Pts',(-0.832776611923762,3.84557854566843,
-35.7410171634434));
#17409=CARTESIAN_POINT('Ctrl Pts',(-0.718533127238244,3.86680735815236,
-35.7468886014));
#17410=CARTESIAN_POINT('Ctrl Pts',(-0.602855936405293,3.88830258301897,
-35.7528337233546));
#17411=CARTESIAN_POINT('Ctrl Pts',(-0.486128770665354,3.90461822605745,
-35.7587788453091));
#17412=CARTESIAN_POINT('Ctrl Pts',(-0.368852899251572,3.91566552947436,
-35.7647239672637));
#17413=CARTESIAN_POINT('Ctrl Pts',(-0.253155744754137,3.92656411888408,
-35.770589058565));
#17414=CARTESIAN_POINT('Ctrl Pts',(-0.136924988936943,3.93233530731509,
-35.7764541498663));
#17415=CARTESIAN_POINT('Ctrl Pts',(-0.020649243143645,3.93294579275606,
-35.7823192411676));
#17416=CARTESIAN_POINT('Ctrl Pts',(0.0956109621152175,3.93355619660417,
-35.7881835485852));
#17417=CARTESIAN_POINT('Ctrl Pts',(0.211915734229722,3.92900726708336,-35.7940478560029));
#17418=CARTESIAN_POINT('Ctrl Pts',(0.327775554067432,3.91931782152912,-35.7999121634206));
#17419=CARTESIAN_POINT('Ctrl Pts',(0.44364759340196,3.909627354049,-35.8057770893347));
#17420=CARTESIAN_POINT('Ctrl Pts',(0.559074177333016,3.89479532703279,-35.8116420152488));
#17421=CARTESIAN_POINT('Ctrl Pts',(0.673570687652138,3.87489245382834,-35.8175069411629));
#17422=CARTESIAN_POINT('Ctrl Pts',(0.79080922096394,3.85451293608866,-35.8235123234251));
#17423=CARTESIAN_POINT('Ctrl Pts',(0.907072117552487,3.82881667211364,-35.8295177056873));
#17424=CARTESIAN_POINT('Ctrl Pts',(1.02185124222059,3.79793483866854,-35.8355230879495));
#17425=CARTESIAN_POINT('Ctrl Pts',(1.1341097237269,3.76773119546511,-35.8413965871208));
#17426=CARTESIAN_POINT('Ctrl Pts',(1.24494855309132,3.73256757789242,-35.8472700862921));
#17427=CARTESIAN_POINT('Ctrl Pts',(1.3539097527593,3.6926166036272,-35.8531435854633));
#17428=CARTESIAN_POINT('Ctrl Pts',(1.4665408618073,3.65132004528578,-35.859214909271));
#17429=CARTESIAN_POINT('Ctrl Pts',(1.5771651834653,3.60490814754724,-35.8652862330786));
#17430=CARTESIAN_POINT('Ctrl Pts',(1.68530264677118,3.55362406407685,-35.8713575568863));
#17431=CARTESIAN_POINT('Ctrl Pts',(1.79344011007705,3.50233998060646,-35.8774288806939));
#17432=CARTESIAN_POINT('Ctrl Pts',(1.89909032273816,3.44618399296587,-35.8835002045016));
#17433=CARTESIAN_POINT('Ctrl Pts',(2.00180549605808,3.38544882636729,-35.8895715283092));
#17434=CARTESIAN_POINT('Ctrl Pts',(2.1013620714965,3.32658132899761,-35.8954561526265));
#17435=CARTESIAN_POINT('Ctrl Pts',(2.19847801556756,3.26322502789782,-35.9013407769437));
#17436=CARTESIAN_POINT('Ctrl Pts',(2.29272294013962,3.19560800470858,-35.9072254012609));
#17437=CARTESIAN_POINT('Ctrl Pts',(2.38684977736114,3.12807570454455,-35.91310265224));
#17438=CARTESIAN_POINT('Ctrl Pts',(2.47811241854201,3.05629353807602,-35.9189799032191));
#17439=CARTESIAN_POINT('Ctrl Pts',(2.56610641169226,2.980534664095,-35.9248571541983));
#17440=CARTESIAN_POINT('Ctrl Pts',(2.65401338637372,2.90485070910531,-35.9307285930831));
#17441=CARTESIAN_POINT('Ctrl Pts',(2.73865783338161,2.82519813675476,-35.936600031968));
#17442=CARTESIAN_POINT('Ctrl Pts',(2.81966609718282,2.74189206578191,-35.9424714708529));
#17443=CARTESIAN_POINT('Ctrl Pts',(2.90169096178298,2.65754055803096,-35.9484165924608));
#17444=CARTESIAN_POINT('Ctrl Pts',(2.979987402897,2.56944347077906,-35.9543617140686));
#17445=CARTESIAN_POINT('Ctrl Pts',(3.05420363075142,2.4779687612851,-35.9603068356765));
#17446=CARTESIAN_POINT('Ctrl Pts',(3.12742080782104,2.38772542507636,-35.9661719279083));
#17447=CARTESIAN_POINT('Ctrl Pts',(3.196666687942,2.29419517737096,-35.9720370201401));
#17448=CARTESIAN_POINT('Ctrl Pts',(3.26164265077544,2.19776618834729,-35.9779021123719));
#17449=CARTESIAN_POINT('Ctrl Pts',(3.32660992940628,2.10135008730311,-35.9837664207193));
#17450=CARTESIAN_POINT('Ctrl Pts',(3.3873081959877,2.0020363564448,-35.9896307290666));
#17451=CARTESIAN_POINT('Ctrl Pts',(3.44348170183205,1.90024281847026,-35.9954950374139));
#17452=CARTESIAN_POINT('Ctrl Pts',(3.49966113216127,1.79843854457555,-36.0013599642558));
#17453=CARTESIAN_POINT('Ctrl Pts',(3.55131465437506,1.6941543037207,-36.0072248910976));
#17454=CARTESIAN_POINT('Ctrl Pts',(3.59823242615284,1.58783261314983,-36.0130898179395));
#17455=CARTESIAN_POINT('Ctrl Pts',(3.6462737915181,1.47896471534855,-36.019095198898));
#17456=CARTESIAN_POINT('Ctrl Pts',(3.68934950422021,1.36796095135993,-36.0251005798565));
#17457=CARTESIAN_POINT('Ctrl Pts',(3.72728700246295,1.2553169325994,-36.031105960815));
#17458=CARTESIAN_POINT('Ctrl Pts',(3.76439137614381,1.14514662726556,-36.0369794609007));
#17459=CARTESIAN_POINT('Ctrl Pts',(3.79658082777674,1.03340778284127,-36.0428529609865));
#17460=CARTESIAN_POINT('Ctrl Pts',(3.82374509287204,0.920577245393874,-36.0487264610722));
#17461=CARTESIAN_POINT('Ctrl Pts',(3.85182425886221,0.803946540361708,-36.0547977824671));
#17462=CARTESIAN_POINT('Ctrl Pts',(3.8745336789633,0.686149785033932,-36.060869103862));
#17463=CARTESIAN_POINT('Ctrl Pts',(3.8918095410351,0.567721319229954,-36.0669404252569));
#17464=CARTESIAN_POINT('Ctrl Pts',(3.90908540310689,0.449292853425975,-36.0730117466518));
#17465=CARTESIAN_POINT('Ctrl Pts',(3.92092772396887,0.330233159728559,-36.0790830680467));
#17466=CARTESIAN_POINT('Ctrl Pts',(3.92733184454616,0.21107719633736,-36.0851543894417));
#17467=CARTESIAN_POINT('Ctrl Pts',(3.93108772010556,0.141194850235918,-36.0887150856161));
#17468=CARTESIAN_POINT('Ctrl Pts',(3.9329785201217,0.0712113825834814,-36.0922757817906));
#17469=CARTESIAN_POINT('Ctrl Pts',(3.93299981803583,0.0011963820870183,
-36.095836477965));
#17470=CARTESIAN_POINT('',(3.93299985616677,0.0010636691862063,-37.3458364779175));
#17471=CARTESIAN_POINT('Ctrl Pts',(3.93299981803602,0.00119638148616424,
-36.0958364779956));
#17472=CARTESIAN_POINT('Ctrl Pts',(3.93303472923432,-0.113571138876911,
-36.1016731168274));
#17473=CARTESIAN_POINT('Ctrl Pts',(3.92804190460838,-0.228532354691529,
-36.1075097556592));
#17474=CARTESIAN_POINT('Ctrl Pts',(3.91799665328228,-0.343207262261184,
-36.113346394491));
#17475=CARTESIAN_POINT('Ctrl Pts',(3.90796365309392,-0.457742312893272,
-36.1191759149876));
#17476=CARTESIAN_POINT('Ctrl Pts',(3.89289051400948,-0.571991335969501,
-36.1250054354842));
#17477=CARTESIAN_POINT('Ctrl Pts',(3.87280455357822,-0.685473478541502,
-36.1308349559808));
#17478=CARTESIAN_POINT('Ctrl Pts',(3.85273755558346,-0.798848486683462,
-36.1366589730357));
#17479=CARTESIAN_POINT('Ctrl Pts',(3.82766722039873,-0.91145764399696,-36.1424829900906));
#17480=CARTESIAN_POINT('Ctrl Pts',(3.7976726789898,-1.02282511860751,-36.1483070071455));
#17481=CARTESIAN_POINT('Ctrl Pts',(3.76769688722855,-1.13412297718745,-36.1541273835957));
#17482=CARTESIAN_POINT('Ctrl Pts',(3.73280311890834,-1.24418029337354,-36.159947760046));
#17483=CARTESIAN_POINT('Ctrl Pts',(3.69312146758863,-1.35253200540173,-36.1657681364962));
#17484=CARTESIAN_POINT('Ctrl Pts',(3.65345227475206,-1.46084969923931,-36.1715866855763));
#17485=CARTESIAN_POINT('Ctrl Pts',(3.60899833068204,-1.56746246052562,-36.1774052346565));
#17486=CARTESIAN_POINT('Ctrl Pts',(3.55993919554999,-1.67192162614964,-36.1832237837367));
#17487=CARTESIAN_POINT('Ctrl Pts',(3.5108832290179,-1.77637404503209,-36.1890419570121));
#17488=CARTESIAN_POINT('Ctrl Pts',(3.45722284116619,-1.87867276600166,-36.1948601302875));
#17489=CARTESIAN_POINT('Ctrl Pts',(3.39918489340035,-1.97839102820419,-36.200678303563));
#17490=CARTESIAN_POINT('Ctrl Pts',(3.34113622069995,-2.07812771751998,-36.2064975519889));
#17491=CARTESIAN_POINT('Ctrl Pts',(3.27870859125413,-2.17528263869596,-36.2123168004148));
#17492=CARTESIAN_POINT('Ctrl Pts',(3.2121733758323,-2.26945614709651,-36.2181360488407));
#17493=CARTESIAN_POINT('Ctrl Pts',(3.14557087454878,-2.36372489146527,-36.2239611821675));
#17494=CARTESIAN_POINT('Ctrl Pts',(3.07485273583628,-2.45500586105009,-36.2297863154942));
#17495=CARTESIAN_POINT('Ctrl Pts',(3.00033201241088,-2.54293075314734,-36.235611448821));
#17496=CARTESIAN_POINT('Ctrl Pts',(2.92576983950635,-2.63090455031169,-36.2414398221692));
#17497=CARTESIAN_POINT('Ctrl Pts',(2.84740115471939,-2.71551824625154,-36.2472681955174));
#17498=CARTESIAN_POINT('Ctrl Pts',(2.76557616733952,-2.79644014108003,-36.2530965688656));
#17499=CARTESIAN_POINT('Ctrl Pts',(2.68362851809338,-2.8774833439705,-36.2589336793878));
#17500=CARTESIAN_POINT('Ctrl Pts',(2.59821453075075,-2.95482341483499,-36.26477078991));
#17501=CARTESIAN_POINT('Ctrl Pts',(2.50971793012842,-3.02816857377391,-36.2706079004322));
#17502=CARTESIAN_POINT('Ctrl Pts',(2.45852747378525,-3.07059474755056,-36.2739843504795));
#17503=CARTESIAN_POINT('Ctrl Pts',(2.40630614479675,-3.11168501738728,-36.2773608005268));
#17504=CARTESIAN_POINT('Ctrl Pts',(2.3531323840611,-3.15138969076865,-36.280737250574));
#17505=CARTESIAN_POINT('Ctrl Pts',(2.26045884695663,-3.22058871808819,-36.2866218742006));
#17506=CARTESIAN_POINT('Ctrl Pts',(2.16458299500471,-3.28580638831883,-36.2925064978272));
#17507=CARTESIAN_POINT('Ctrl Pts',(2.06588109249667,-3.34673337923187,-36.2983911214538));
#17508=CARTESIAN_POINT('Ctrl Pts',(1.96730286215315,-3.40758402943968,-36.3042683717257));
#17509=CARTESIAN_POINT('Ctrl Pts',(1.86590597102965,-3.46415447885765,-36.3101456219975));
#17510=CARTESIAN_POINT('Ctrl Pts',(1.76209829182777,-3.51617670345756,-36.3160228722693));
#17511=CARTESIAN_POINT('Ctrl Pts',(1.65839326975319,-3.56814748242093,-36.3218943104314));
#17512=CARTESIAN_POINT('Ctrl Pts',(1.55228256797723,-3.61557880094452,-36.3277657485934));
#17513=CARTESIAN_POINT('Ctrl Pts',(1.44420091878299,-3.65824721775147,-36.3336371867555));
#17514=CARTESIAN_POINT('Ctrl Pts',(1.33476289713381,-3.70145110256511,-36.3395823086284));
#17515=CARTESIAN_POINT('Ctrl Pts',(1.22330448215648,-3.73977149249103,-36.3455274305014));
#17516=CARTESIAN_POINT('Ctrl Pts',(1.1103007451359,-3.773025477697,-36.3514725523743));
#17517=CARTESIAN_POINT('Ctrl Pts',(0.998818210562108,-3.80583181360398,
-36.3573376438502));
#17518=CARTESIAN_POINT('Ctrl Pts',(0.885832111814612,-3.83370719955568,
-36.3632027353262));
#17519=CARTESIAN_POINT('Ctrl Pts',(0.771815692665296,-3.85652557836138,
-36.3690678268021));
#17520=CARTESIAN_POINT('Ctrl Pts',(0.657814512314632,-3.87934090738985,
-36.3749321343826));
#17521=CARTESIAN_POINT('Ctrl Pts',(0.542783688610737,-3.89710049282084,
-36.3807964419631));
#17522=CARTESIAN_POINT('Ctrl Pts',(0.427207315885236,-3.90972926290992,
-36.3866607495436));
#17523=CARTESIAN_POINT('Ctrl Pts',(0.311618753792879,-3.92235936490367,
-36.3925256756086));
#17524=CARTESIAN_POINT('Ctrl Pts',(0.195484937133343,-3.92985753116021,
-36.3983906016736));
#17525=CARTESIAN_POINT('Ctrl Pts',(0.0792950664487206,-3.93220056615083,
-36.4042555277387));
#17526=CARTESIAN_POINT('Ctrl Pts',(-0.0396773724094786,-3.93459971321521,
-36.410260909736));
#17527=CARTESIAN_POINT('Ctrl Pts',(-0.158708130861955,-3.93159365437423,
-36.4162662917333));
#17528=CARTESIAN_POINT('Ctrl Pts',(-0.277273370872376,-3.92321404945041,
-36.4222716737306));
#17529=CARTESIAN_POINT('Ctrl Pts',(-0.393234829030164,-3.91501846695366,
-36.4281451730221));
#17530=CARTESIAN_POINT('Ctrl Pts',(-0.508750597896959,-3.9016830282927,
-36.4340186723136));
#17531=CARTESIAN_POINT('Ctrl Pts',(-0.623338153738285,-3.88328965518852,
-36.4398921716052));
#17532=CARTESIAN_POINT('Ctrl Pts',(-0.741785108251943,-3.86427677886501,
-36.4459634949554));
#17533=CARTESIAN_POINT('Ctrl Pts',(-0.859239746550688,-3.83985934955294,
-36.4520348183055));
#17534=CARTESIAN_POINT('Ctrl Pts',(-0.975184380020213,-3.81018430328043,
-36.4581061416557));
#17535=CARTESIAN_POINT('Ctrl Pts',(-1.09112901348974,-3.78050925700792,
-36.4641774650059));
#17536=CARTESIAN_POINT('Ctrl Pts',(-1.20556320326289,-3.74557679518464,
-36.4702487883561));
#17537=CARTESIAN_POINT('Ctrl Pts',(-1.31799147545504,-3.70558868071294,
-36.4763201117063));
#17538=CARTESIAN_POINT('Ctrl Pts',(-1.42696256365722,-3.66683020596125,
-36.482204741074));
#17539=CARTESIAN_POINT('Ctrl Pts',(-1.53439575626693,-3.62319925666182,
-36.4880893704416));
#17540=CARTESIAN_POINT('Ctrl Pts',(-1.63982501144332,-3.57483746929073,
-36.4939739998093));
#17541=CARTESIAN_POINT('Ctrl Pts',(-1.74512216599344,-3.52653627821605,
-36.4998512558609));
#17542=CARTESIAN_POINT('Ctrl Pts',(-1.84842000639157,-3.47351620867746,
-36.5057285119124));
#17543=CARTESIAN_POINT('Ctrl Pts',(-1.94926933526407,-3.41596809976311,
-36.511605767964));
#17544=CARTESIAN_POINT('Ctrl Pts',(-2.05001893320035,-3.35847690076421,
-36.5174772119367));
#17545=CARTESIAN_POINT('Ctrl Pts',(-2.14832448123292,-3.2964667729808,-36.5233486559095));
#17546=CARTESIAN_POINT('Ctrl Pts',(-2.24375899286168,-3.23017562710642,
-36.5292200998822));
#17547=CARTESIAN_POINT('Ctrl Pts',(-2.34039103063641,-3.16305265028245,
-36.5351652195887));
#17548=CARTESIAN_POINT('Ctrl Pts',(-2.43407909406102,-3.09154065538387,
-36.5411103392953));
#17549=CARTESIAN_POINT('Ctrl Pts',(-2.52440756402997,-3.01593359520204,
-36.5470554590018));
#17550=CARTESIAN_POINT('Ctrl Pts',(-2.6135201965227,-2.94134421966899,-36.5529205563262));
#17551=CARTESIAN_POINT('Ctrl Pts',(-2.6993628030752,-2.86276962126291,-36.5587856536506));
#17552=CARTESIAN_POINT('Ctrl Pts',(-2.78156809028633,-2.7805337543538,-36.564650750975));
#17553=CARTESIAN_POINT('Ctrl Pts',(-2.86376239045725,-2.698308878572,-36.5705150644075));
#17554=CARTESIAN_POINT('Ctrl Pts',(-2.94232004745701,-2.61242399830032,
-36.57637937784));
#17555=CARTESIAN_POINT('Ctrl Pts',(-3.01691018322573,-2.52324036634421,
-36.5822436912725));
#17556=CARTESIAN_POINT('Ctrl Pts',(-3.09150818566194,-2.43404732861386,
-36.5881086231863));
#17557=CARTESIAN_POINT('Ctrl Pts',(-3.16213757119426,-2.34155516306203,
-36.5939735551));
#17558=CARTESIAN_POINT('Ctrl Pts',(-3.22850780330919,-2.2461581342309,-36.5998384870138));
#17559=CARTESIAN_POINT('Ctrl Pts',(-3.29646733977885,-2.14847672415659,
-36.6058438608326));
#17560=CARTESIAN_POINT('Ctrl Pts',(-3.35996088153859,-2.04774992820193,
-36.6118492346513));
#17561=CARTESIAN_POINT('Ctrl Pts',(-3.41872434138119,-1.94443124785829,
-36.6178546084701));
#17562=CARTESIAN_POINT('Ctrl Pts',(-3.47619744633893,-1.84338128627688,
-36.6237281135482));
#17563=CARTESIAN_POINT('Ctrl Pts',(-3.52914592394074,-1.7398524930139,-36.6296016186264));
#17564=CARTESIAN_POINT('Ctrl Pts',(-3.57737042052471,-1.63429185715246,
-36.6354751237045));
#17565=CARTESIAN_POINT('Ctrl Pts',(-3.62721898235056,-1.52517623634027,
-36.6415464318935));
#17566=CARTESIAN_POINT('Ctrl Pts',(-3.67201959214682,-1.41388995690449,
-36.6476177400826));
#17567=CARTESIAN_POINT('Ctrl Pts',(-3.7116075074509,-1.30094531423658,-36.6536890482716));
#17568=CARTESIAN_POINT('Ctrl Pts',(-3.75119542275497,-1.18800067156868,
-36.6597603564607));
#17569=CARTESIAN_POINT('Ctrl Pts',(-3.78557056786004,-1.07339814256441,
-36.6658316646497));
#17570=CARTESIAN_POINT('Ctrl Pts',(-3.81462614444298,-0.957661933112155,
-36.6719029728387));
#17571=CARTESIAN_POINT('Ctrl Pts',(-3.84278823538565,-0.845484718295886,
-36.6777875827302));
#17572=CARTESIAN_POINT('Ctrl Pts',(-3.8660426999347,-0.731885884848342,
-36.6836721926216));
#17573=CARTESIAN_POINT('Ctrl Pts',(-3.88424901836939,-0.617331809723478,
-36.689556802513));
#17574=CARTESIAN_POINT('Ctrl Pts',(-3.90243252452278,-0.502921269371648,
-36.6954340390644));
#17575=CARTESIAN_POINT('Ctrl Pts',(-3.9155804009619,-0.387558270641264,
-36.7013112756158));
#17576=CARTESIAN_POINT('Ctrl Pts',(-3.92360241474224,-0.271722452198623,
-36.7071885121672));
#17577=CARTESIAN_POINT('Ctrl Pts',(-3.93161649544519,-0.156001185355937,
-36.7130599366403));
#17578=CARTESIAN_POINT('Ctrl Pts',(-3.9345147692093,-0.03980843702116,-36.7189313611134));
#17579=CARTESIAN_POINT('Ctrl Pts',(-3.93225849176958,0.0763685400279876,
-36.7248027855864));
#17580=CARTESIAN_POINT('Ctrl Pts',(-3.92997389183578,0.194003858009621,
-36.7307479126025));
#17581=CARTESIAN_POINT('Ctrl Pts',(-3.92240437347689,0.31162258351543,-36.7366930396185));
#17582=CARTESIAN_POINT('Ctrl Pts',(-3.90956413481056,0.428715845057024,
-36.7426381666345));
#17583=CARTESIAN_POINT('Ctrl Pts',(-3.8968967854855,0.544232486616664,-36.748503244586));
#17584=CARTESIAN_POINT('Ctrl Pts',(-3.87909983611869,0.659237307992045,
-36.7543683225375));
#17585=CARTESIAN_POINT('Ctrl Pts',(-3.85623924651464,0.773245028202716,
-36.760233400489));
#17586=CARTESIAN_POINT('Ctrl Pts',(-3.83338171200276,0.887237512406752,
-36.7660976946308));
#17587=CARTESIAN_POINT('Ctrl Pts',(-3.80546196394673,1.0002327573192,-36.7719619887725));
#17588=CARTESIAN_POINT('Ctrl Pts',(-3.77259719291646,1.11175510792567,-36.7778262829142));
#17589=CARTESIAN_POINT('Ctrl Pts',(-3.73972895520139,1.22328922227873,-36.7836911956411));
#17590=CARTESIAN_POINT('Ctrl Pts',(-3.70191477382609,1.33334973897271,-36.7895561083679));
#17591=CARTESIAN_POINT('Ctrl Pts',(-3.65932167946615,1.4414762731967,-36.7954210210948));
#17592=CARTESIAN_POINT('Ctrl Pts',(-3.61570830847756,1.55219287460091,-36.8014264221678));
#17593=CARTESIAN_POINT('Ctrl Pts',(-3.56708432021527,1.66088123559898,-36.8074318232409));
#17594=CARTESIAN_POINT('Ctrl Pts',(-3.51368071381787,1.76707012915287,-36.8134372243139));
#17595=CARTESIAN_POINT('Ctrl Pts',(-3.46145017200904,1.8709264755413,-36.8193107106378));
#17596=CARTESIAN_POINT('Ctrl Pts',(-3.40464808210247,1.9723916958076,-36.8251841969617));
#17597=CARTESIAN_POINT('Ctrl Pts',(-3.34353590907388,2.07105205746585,-36.8310576832857));
#17598=CARTESIAN_POINT('Ctrl Pts',(-3.28036492552098,2.17303619212785,-36.8371290417332));
#17599=CARTESIAN_POINT('Ctrl Pts',(-3.21258860658891,2.27202274920149,-36.8432004001808));
#17600=CARTESIAN_POINT('Ctrl Pts',(-3.14054196812054,2.36759057830394,-36.8492717586284));
#17601=CARTESIAN_POINT('Ctrl Pts',(-3.06849532965217,2.46315840740639,-36.855343117076));
#17602=CARTESIAN_POINT('Ctrl Pts',(-2.99217872658223,2.55530718110447,-36.8614144755235));
#17603=CARTESIAN_POINT('Ctrl Pts',(-2.91196921511862,2.64365737004655,-36.8674858339711));
#17604=CARTESIAN_POINT('Ctrl Pts',(-2.83422659571384,2.72929029546813,-36.8733704641159));
#17605=CARTESIAN_POINT('Ctrl Pts',(-2.75257986797348,2.81162715474329,-36.8792550942608));
#17606=CARTESIAN_POINT('Ctrl Pts',(-2.6673392546602,2.8902924247468,-36.8851397244056));
#17607=CARTESIAN_POINT('Ctrl Pts',(-2.58220544780444,2.96885912719558,-36.891016981111));
#17608=CARTESIAN_POINT('Ctrl Pts',(-2.49348701142665,3.04376311380706,-36.8968942378163));
#17609=CARTESIAN_POINT('Ctrl Pts',(-2.40153308591305,3.11466335857745,-36.9027714945217));
#17610=CARTESIAN_POINT('Ctrl Pts',(-2.30967009648456,3.18549348789973,-36.9086429390259));
#17611=CARTESIAN_POINT('Ctrl Pts',(-2.2145783070513,3.25232750222358,-36.9145143835301));
#17612=CARTESIAN_POINT('Ctrl Pts',(-2.11664174195745,3.31486300413808,-36.9203858280343));
#17613=CARTESIAN_POINT('Ctrl Pts',(-2.01747626765401,3.37818320229096,-36.9263309474955));
#17614=CARTESIAN_POINT('Ctrl Pts',(-1.91539444734215,3.43709597863483,-36.9322760669567));
#17615=CARTESIAN_POINT('Ctrl Pts',(-1.81082764429584,3.4913310130456,-36.938221186418));
#17616=CARTESIAN_POINT('Ctrl Pts',(-1.70766832093664,3.54483603843782,-36.9440862839732));
#17617=CARTESIAN_POINT('Ctrl Pts',(-1.60209088022816,3.59378828775386,-36.9499513815285));
#17618=CARTESIAN_POINT('Ctrl Pts',(-1.49453575747148,3.63797359386227,-36.9558164790838));
#17619=CARTESIAN_POINT('Ctrl Pts',(-1.38699501191209,3.6821529935959,-36.9616807926349));
#17620=CARTESIAN_POINT('Ctrl Pts',(-1.27747749040105,3.72156656118633,-36.9675451061859));
#17621=CARTESIAN_POINT('Ctrl Pts',(-1.16644402171783,3.75604810195486,-36.973409419737));
#17622=CARTESIAN_POINT('Ctrl Pts',(-1.05539884497981,3.79053327867005,-36.9792743516576));
#17623=CARTESIAN_POINT('Ctrl Pts',(-0.942837796059542,3.82008527273901,
-36.9851392835781));
#17624=CARTESIAN_POINT('Ctrl Pts',(-0.829236628951203,3.84458783398242,
-36.9910042154987));
#17625=CARTESIAN_POINT('Ctrl Pts',(-0.712915173716917,3.86967713238798,
-36.9970095887991));
#17626=CARTESIAN_POINT('Ctrl Pts',(-0.595503594897514,3.88947198999402,
-37.0030149620995));
#17627=CARTESIAN_POINT('Ctrl Pts',(-0.477522124356276,3.90390338260955,
-37.0090203353999));
#17628=CARTESIAN_POINT('Ctrl Pts',(-0.362131340119266,3.91801788469109,
-37.0148938402103));
#17629=CARTESIAN_POINT('Ctrl Pts',(-0.246195853650308,3.92700206931307,
-37.0207673450208));
#17630=CARTESIAN_POINT('Ctrl Pts',(-0.130204952198965,3.93084414221969,
-37.0266408498313));
#17631=CARTESIAN_POINT('Ctrl Pts',(-0.0103078110709597,3.93481560508226,
-37.0327121573767));
#17632=CARTESIAN_POINT('Ctrl Pts',(0.109648058222881,3.93329251379023,-37.038783464922));
#17633=CARTESIAN_POINT('Ctrl Pts',(0.229126433390375,3.92632017002203,-37.0448547724674));
#17634=CARTESIAN_POINT('Ctrl Pts',(0.34860480855787,3.91934782625383,-37.0509260800128));
#17635=CARTESIAN_POINT('Ctrl Pts',(0.467605220340459,3.90692634384008,-37.0569973875581));
#17636=CARTESIAN_POINT('Ctrl Pts',(0.58560277456768,3.88915908525463,-37.0630686951035));
#17637=CARTESIAN_POINT('Ctrl Pts',(0.699972824622961,3.87193803124999,-37.0689533573104));
#17638=CARTESIAN_POINT('Ctrl Pts',(0.813764377535811,3.84964035700378,-37.0748380195173));
#17639=CARTESIAN_POINT('Ctrl Pts',(0.926492909708655,3.82231603720304,-37.0807226817242));
#17640=CARTESIAN_POINT('Ctrl Pts',(1.0390801998307,3.79502595312676,-37.0865999708043));
#17641=CARTESIAN_POINT('Ctrl Pts',(1.15060672192642,3.76272184592289,-37.0924772598844));
#17642=CARTESIAN_POINT('Ctrl Pts',(1.26059508478111,3.72550520496559,-37.0983545489645));
#17643=CARTESIAN_POINT('Ctrl Pts',(1.37047468235874,3.68832536679506,-37.1042260261118));
#17644=CARTESIAN_POINT('Ctrl Pts',(1.47881875913099,3.64624278994846,-37.1100975032591));
#17645=CARTESIAN_POINT('Ctrl Pts',(1.58516273091977,3.59940941218181,-37.1159689804064));
#17646=CARTESIAN_POINT('Ctrl Pts',(1.69284028972156,3.55198872905769,-37.1219140877326));
#17647=CARTESIAN_POINT('Ctrl Pts',(1.79846681826055,3.49969737174488,-37.1278591950588));
#17648=CARTESIAN_POINT('Ctrl Pts',(1.90157819206338,3.44274445456949,-37.1338043023851));
#17649=CARTESIAN_POINT('Ctrl Pts',(2.00330245784964,3.38655769776096,-37.1396694330246));
#17650=CARTESIAN_POINT('Ctrl Pts',(2.10257845799757,3.3258342435757,-37.1455345636642));
#17651=CARTESIAN_POINT('Ctrl Pts',(2.19898375965077,3.2608218940617,-37.1513996943038));
#17652=CARTESIAN_POINT('Ctrl Pts',(2.29537617632454,3.1958182337253,-37.1572640410437));
#17653=CARTESIAN_POINT('Ctrl Pts',(2.38889831669172,3.1265270480034,-37.1631283877836));
#17654=CARTESIAN_POINT('Ctrl Pts',(2.47915636493696,3.0532397086034,-37.1689927345235));
#17655=CARTESIAN_POINT('Ctrl Pts',(2.56942393150794,2.97994464055445,-37.1748576996986));
#17656=CARTESIAN_POINT('Ctrl Pts',(2.65642640240147,2.90265284030614,-37.1807226648738));
#17657=CARTESIAN_POINT('Ctrl Pts',(2.73980325177983,2.82169579181326,-37.186587630049));
#17658=CARTESIAN_POINT('Ctrl Pts',(2.82517549952317,2.73880125631528,-37.1925929572312));
#17659=CARTESIAN_POINT('Ctrl Pts',(2.90674604863093,2.65206411590826,-37.1985982844134));
#17660=CARTESIAN_POINT('Ctrl Pts',(2.98416902896958,2.56187903823322,-37.2046036115957));
#17661=CARTESIAN_POINT('Ctrl Pts',(3.05989293159331,2.47367310751204,-37.210477149514));
#17662=CARTESIAN_POINT('Ctrl Pts',(3.13164922179133,2.38216937861496,-37.2163506874324));
#17663=CARTESIAN_POINT('Ctrl Pts',(3.1991568005265,2.28776851225054,-37.2222242253508));
#17664=CARTESIAN_POINT('Ctrl Pts',(3.2689364614968,2.19019042437312,-37.2282954471649));
#17665=CARTESIAN_POINT('Ctrl Pts',(3.33417611327404,2.08951715404321,-37.2343666689791));
#17666=CARTESIAN_POINT('Ctrl Pts',(3.39461616518399,1.98622005101941,-37.2404378907933));
#17667=CARTESIAN_POINT('Ctrl Pts',(3.45505621709394,1.88292294799562,-37.2465091126075));
#17668=CARTESIAN_POINT('Ctrl Pts',(3.51069650370839,1.77700246586642,-37.2525803344216));
#17669=CARTESIAN_POINT('Ctrl Pts',(3.56133203022404,1.66895271667604,-37.2586515562358));
#17670=CARTESIAN_POINT('Ctrl Pts',(3.61423885573669,1.55605630539188,-37.2649951077949));
#17671=CARTESIAN_POINT('Ctrl Pts',(3.66183034001354,1.44052089285038,-37.2713386593539));
#17672=CARTESIAN_POINT('Ctrl Pts',(3.70385729676319,1.32284924508202,-37.2776822109129));
#17673=CARTESIAN_POINT('Ctrl Pts',(3.74575017190444,1.20555301359443,-37.2840055241854));
#17674=CARTESIAN_POINT('Ctrl Pts',(3.78211381721462,1.0861344272398,-37.2903288374578));
#17675=CARTESIAN_POINT('Ctrl Pts',(3.81274711943031,0.965115746051162,-37.2966521507302));
#17676=CARTESIAN_POINT('Ctrl Pts',(3.84331913759382,0.844339171153237,-37.3029628137746));
#17677=CARTESIAN_POINT('Ctrl Pts',(3.86818358034013,0.721969177049568,-37.3092734768189));
#17678=CARTESIAN_POINT('Ctrl Pts',(3.88718829857242,0.598545012043067,-37.3155841398632));
#17679=CARTESIAN_POINT('Ctrl Pts',(3.90613595983782,0.475491397570901,-37.3218758567023));
#17680=CARTESIAN_POINT('Ctrl Pts',(3.91925892408688,0.351390225876226,-37.3281675735414));
#17681=CARTESIAN_POINT('Ctrl Pts',(3.9264557247084,0.226791626619253,-37.3344592903805));
#17682=CARTESIAN_POINT('Ctrl Pts',(3.9307936689416,0.151688562975241,-37.3382516862262));
#17683=CARTESIAN_POINT('Ctrl Pts',(3.93297948029164,0.0764050582108798,
-37.3420440820718));
#17684=CARTESIAN_POINT('Ctrl Pts',(3.93299985616677,0.00106366918621726,
-37.3458364779175));
#17685=CARTESIAN_POINT('Ctrl Pts',(3.93299985616703,0.00106366824158364,
-37.345836477965));
#17686=CARTESIAN_POINT('Ctrl Pts',(3.9330321879552,-0.118485748811121,-37.3518541359674));
#17687=CARTESIAN_POINT('Ctrl Pts',(3.92760934873402,-0.237986703531313,
-37.3578717939699));
#17688=CARTESIAN_POINT('Ctrl Pts',(3.91677077722735,-0.356925312436485,
-37.3638894519723));
#17689=CARTESIAN_POINT('Ctrl Pts',(3.9059248975669,-0.475944118408449,-37.3699111675177));
#17690=CARTESIAN_POINT('Ctrl Pts',(3.8896560441002,-0.594399445105386,-37.3759328830631));
#17691=CARTESIAN_POINT('Ctrl Pts',(3.86805530385929,-0.711784494271979,
-37.3819545986086));
#17692=CARTESIAN_POINT('Ctrl Pts',(3.84641826160541,-0.829366819713841,
-37.3879864341959));
#17693=CARTESIAN_POINT('Ctrl Pts',(3.81943149570112,-0.945874899042958,
-37.3940182697832));
#17694=CARTESIAN_POINT('Ctrl Pts',(3.78723705854409,-1.06081311379069,-37.4000501053705));
#17695=CARTESIAN_POINT('Ctrl Pts',(3.75501541025168,-1.17584847573518,-37.4060870391396));
#17696=CARTESIAN_POINT('Ctrl Pts',(3.71757743273379,-1.28931096675788,-37.4121239729087));
#17697=CARTESIAN_POINT('Ctrl Pts',(3.67511420835027,-1.40072286894374,-37.4181609066779));
#17698=CARTESIAN_POINT('Ctrl Pts',(3.63256382233341,-1.51236345944775,-37.4242102320874));
#17699=CARTESIAN_POINT('Ctrl Pts',(3.58496771857707,-1.62194469683356,-37.430259557497));
#17700=CARTESIAN_POINT('Ctrl Pts',(3.53256454584281,-1.72901033237352,-37.4363088829065));
#17701=CARTESIAN_POINT('Ctrl Pts',(3.48080368463642,-1.83476365248756,-37.4422840610604));
#17702=CARTESIAN_POINT('Ctrl Pts',(3.42435318210951,-1.93806242851611,-37.4482592392143));
#17703=CARTESIAN_POINT('Ctrl Pts',(3.36348441947456,-2.03849492517198,-37.4542344173682));
#17704=CARTESIAN_POINT('Ctrl Pts',(3.30353718729878,-2.13740691112987,-37.4601191335441));
#17705=CARTESIAN_POINT('Ctrl Pts',(3.23912784186652,-2.23382952484871,-37.46600384972));
#17706=CARTESIAN_POINT('Ctrl Pts',(3.17048913890051,-2.32733487494041,-37.4718885658958));
#17707=CARTESIAN_POINT('Ctrl Pts',(3.10193644549645,-2.42072305565313,-37.4777659080708));
#17708=CARTESIAN_POINT('Ctrl Pts',(3.02916517655114,-2.51120091460067,-37.4836432502457));
#17709=CARTESIAN_POINT('Ctrl Pts',(2.952452880109,-2.59836698538449,-37.4895205924206));
#17710=CARTESIAN_POINT('Ctrl Pts',(2.8758164543284,-2.6854468464241,-37.4953921217355));
#17711=CARTESIAN_POINT('Ctrl Pts',(2.79524702526215,-2.76922112821716,-37.5012636510505));
#17712=CARTESIAN_POINT('Ctrl Pts',(2.71106376348625,-2.84931961533131,-37.5071351803654));
#17713=CARTESIAN_POINT('Ctrl Pts',(2.62582585971236,-2.93042157067305,-37.5130802677877));
#17714=CARTESIAN_POINT('Ctrl Pts',(2.53688320539153,-3.00775465232699,-37.51902535521));
#17715=CARTESIAN_POINT('Ctrl Pts',(2.44460754525337,-3.0809711049749,-37.5249704426323));
#17716=CARTESIAN_POINT('Ctrl Pts',(2.35357215113052,-3.15320346411599,-37.5308356228518));
#17717=CARTESIAN_POINT('Ctrl Pts',(2.25929313613745,-3.22142892218565,-37.5367008030713));
#17718=CARTESIAN_POINT('Ctrl Pts',(2.16216190151178,-3.28535308782039,-37.5425659832908));
#17719=CARTESIAN_POINT('Ctrl Pts',(2.06504366620733,-3.34926869832077,-37.5484303785583));
#17720=CARTESIAN_POINT('Ctrl Pts',(1.96507431389771,-3.40888393523525,-37.5542947738257));
#17721=CARTESIAN_POINT('Ctrl Pts',(1.86267443087605,-3.46394759841436,-37.5601591690932));
#17722=CARTESIAN_POINT('Ctrl Pts',(1.76026376843625,-3.5190170580283,-37.5660241816931));
#17723=CARTESIAN_POINT('Ctrl Pts',(1.6554224288657,-3.56953379664985,-37.571889194293));
#17724=CARTESIAN_POINT('Ctrl Pts',(1.54859519303285,-3.61529278594633,-37.5777542068928));
#17725=CARTESIAN_POINT('Ctrl Pts',(1.43921351916066,-3.66214595784511,-37.5837594628602));
#17726=CARTESIAN_POINT('Ctrl Pts',(1.3277501828572,-3.7040107694697,-37.5897647188275));
#17727=CARTESIAN_POINT('Ctrl Pts',(1.21470259933593,-3.74072006372657,-37.5957699747948));
#17728=CARTESIAN_POINT('Ctrl Pts',(1.10413374470272,-3.77662445454986,-37.6016435569927));
#17729=CARTESIAN_POINT('Ctrl Pts',(0.992049819009357,-3.80759703358294,
-37.6075171391906));
#17730=CARTESIAN_POINT('Ctrl Pts',(0.878928848537685,-3.83353271529124,
-37.6133907213885));
#17731=CARTESIAN_POINT('Ctrl Pts',(0.762003964862561,-3.86034053486822,
-37.6194618142405));
#17732=CARTESIAN_POINT('Ctrl Pts',(0.643971540502412,-3.88176665637471,
-37.6255329070925));
#17733=CARTESIAN_POINT('Ctrl Pts',(0.525366507130672,-3.89775307493757,
-37.6316039999445));
#17734=CARTESIAN_POINT('Ctrl Pts',(0.406761473758932,-3.91373949350043,
-37.6376750927966));
#17735=CARTESIAN_POINT('Ctrl Pts',(0.287584313608817,-3.92428623115194,
-37.6437461856486));
#17736=CARTESIAN_POINT('Ctrl Pts',(0.168369936222375,-3.92939442720841,
-37.6498172785006));
#17737=CARTESIAN_POINT('Ctrl Pts',(0.052812542204191,-3.93434592582258,
-37.6557021363861));
#17738=CARTESIAN_POINT('Ctrl Pts',(-0.0631470300060075,-3.93420344049839,
-37.6615869942715));
#17739=CARTESIAN_POINT('Ctrl Pts',(-0.17902360411251,-3.92892345931689,
-37.667471852157));
#17740=CARTESIAN_POINT('Ctrl Pts',(-0.294755027470508,-3.92365009201076,
-37.6733493384789));
#17741=CARTESIAN_POINT('Ctrl Pts',(-0.410403252154865,-3.91325204689014,
-37.6792268248008));
#17742=CARTESIAN_POINT('Ctrl Pts',(-0.525480261887363,-3.89773774058322,
-37.6851043111228));
#17743=CARTESIAN_POINT('Ctrl Pts',(-0.640443503513937,-3.88223877212047,
-37.6909759868098));
#17744=CARTESIAN_POINT('Ctrl Pts',(-0.754836248274933,-3.86163365930045,
-37.6968476624969));
#17745=CARTESIAN_POINT('Ctrl Pts',(-0.868173413332504,-3.83598278468277,
-37.7027193381839));
#17746=CARTESIAN_POINT('Ctrl Pts',(-0.982926554842207,-3.81001144118433,
-37.7086643715776));
#17747=CARTESIAN_POINT('Ctrl Pts',(-1.09659713254844,-3.7788674114688,-37.7146094049713));
#17748=CARTESIAN_POINT('Ctrl Pts',(-1.20868965893546,-3.74266727193087,
-37.7205544383651));
#17749=CARTESIAN_POINT('Ctrl Pts',(-1.31927941210295,-3.70695245110235,
-37.7264197694159));
#17750=CARTESIAN_POINT('Ctrl Pts',(-1.42833276785933,-3.66631640021433,
-37.7322851004667));
#17751=CARTESIAN_POINT('Ctrl Pts',(-1.53538770225576,-3.6209216511493,-37.7381504315175));
#17752=CARTESIAN_POINT('Ctrl Pts',(-1.64242833489751,-3.57553296649007,
-37.7440149790031));
#17753=CARTESIAN_POINT('Ctrl Pts',(-1.74747069864278,-3.5253870085123,-37.7498795264887));
#17754=CARTESIAN_POINT('Ctrl Pts',(-1.85007253448565,-3.47069454391219,
-37.7557440739742));
#17755=CARTESIAN_POINT('Ctrl Pts',(-1.95268519180486,-3.41599631086548,
-37.7616092399971));
#17756=CARTESIAN_POINT('Ctrl Pts',(-2.0528564466283,-3.35675081137584,-37.76747440602));
#17757=CARTESIAN_POINT('Ctrl Pts',(-2.15016905196046,-3.29321454630449,
-37.7733395720429));
#17758=CARTESIAN_POINT('Ctrl Pts',(-2.24980251426086,-3.22816297308755,
-37.779344619342));
#17759=CARTESIAN_POINT('Ctrl Pts',(-2.34643885969176,-3.15861361566418,
-37.7853496666412));
#17760=CARTESIAN_POINT('Ctrl Pts',(-2.43966325082814,-3.0848877163616,-37.7913547139404));
#17761=CARTESIAN_POINT('Ctrl Pts',(-2.53084913873483,-3.01277395399022,
-37.7972284510946));
#17762=CARTESIAN_POINT('Ctrl Pts',(-2.61877048248721,-2.93666474777405,
-37.8031021882488));
#17763=CARTESIAN_POINT('Ctrl Pts',(-2.70307477628502,-2.85689967513941,
-37.808975925403));
#17764=CARTESIAN_POINT('Ctrl Pts',(-2.79020606303856,-2.7744598241715,-37.8150466277747));
#17765=CARTESIAN_POINT('Ctrl Pts',(-2.87347312209116,-2.68811496539785,
-37.8211173301463));
#17766=CARTESIAN_POINT('Ctrl Pts',(-2.9525311689054,-2.59827802527792,-37.827188032518));
#17767=CARTESIAN_POINT('Ctrl Pts',(-3.03158921571963,-2.50844108515799,
-37.8332587348896));
#17768=CARTESIAN_POINT('Ctrl Pts',(-3.1064380013842,-2.41511247701759,-37.8393294372613));
#17769=CARTESIAN_POINT('Ctrl Pts',(-3.17678195644198,-2.31873788972033,
-37.8454001396329));
#17770=CARTESIAN_POINT('Ctrl Pts',(-3.24495953773304,-2.22533133823407,
-37.8512838833618));
#17771=CARTESIAN_POINT('Ctrl Pts',(-3.30912257044277,-2.12876658268556,
-37.8571676270907));
#17772=CARTESIAN_POINT('Ctrl Pts',(-3.36896585726649,-2.02942308367985,
-37.8630513708196));
#17773=CARTESIAN_POINT('Ctrl Pts',(-3.42873413691139,-1.93020410115695,
-37.8689277399031));
#17774=CARTESIAN_POINT('Ctrl Pts',(-3.4841932287675,-1.82821365167522,-37.8748041089867));
#17775=CARTESIAN_POINT('Ctrl Pts',(-3.53507956927122,-1.72386236078209,
-37.8806804780702));
#17776=CARTESIAN_POINT('Ctrl Pts',(-3.5859155782458,-1.61961428344266,-37.8865510348544));
#17777=CARTESIAN_POINT('Ctrl Pts',(-3.63218765399647,-1.51301037771174,
-37.8924215916386));
#17778=CARTESIAN_POINT('Ctrl Pts',(-3.67367710123949,-1.4044876488701,-37.8982921484229));
#17779=CARTESIAN_POINT('Ctrl Pts',(-3.71569586260464,-1.29458040862218,
-37.9042376006038));
#17780=CARTESIAN_POINT('Ctrl Pts',(-3.75280888822166,-1.18270540918299,
-37.9101830527847));
#17781=CARTESIAN_POINT('Ctrl Pts',(-3.78483834382535,-1.06933984827526,
-37.9161285049657));
#17782=CARTESIAN_POINT('Ctrl Pts',(-3.81643015856616,-0.957523280347951,
-37.9219927202734));
#17783=CARTESIAN_POINT('Ctrl Pts',(-3.84307635110814,-0.844257040098927,
-37.9278569355812));
#17784=CARTESIAN_POINT('Ctrl Pts',(-3.8646560300124,-0.730015595510648,
-37.933721150889));
#17785=CARTESIAN_POINT('Ctrl Pts',(-3.8862328372021,-0.615789353596278,
-37.9395845858166));
#17786=CARTESIAN_POINT('Ctrl Pts',(-3.90274439532046,-0.500588569600884,
-37.9454480207442));
#17787=CARTESIAN_POINT('Ctrl Pts',(-3.91412091324391,-0.384898007927584,
-37.9513114556719));
#17788=CARTESIAN_POINT('Ctrl Pts',(-3.92549863990729,-0.269195154285753,
-37.9571755135817));
#17789=CARTESIAN_POINT('Ctrl Pts',(-3.93174020151445,-0.15300282894872,
-37.9630395714915));
#17790=CARTESIAN_POINT('Ctrl Pts',(-3.93282773574889,-0.0368103371924791,
-37.9689036294013));
#17791=CARTESIAN_POINT('Ctrl Pts',(-3.93394170814879,0.0822068162847243,
-37.9749102436816));
#17792=CARTESIAN_POINT('Ctrl Pts',(-3.92964781478223,0.201223689949559,
-37.980916857962));
#17793=CARTESIAN_POINT('Ctrl Pts',(-3.91998347243803,0.319716399036246,
-37.9869234722423));
#17794=CARTESIAN_POINT('Ctrl Pts',(-3.9105346715888,0.435566393828449,-37.992796122454));
#17795=CARTESIAN_POINT('Ctrl Pts',(-3.89595257684535,0.550914954431655,
-37.9986687726656));
#17796=CARTESIAN_POINT('Ctrl Pts',(-3.87632438227948,0.665280604967251,
-38.0045414228772));
#17797=CARTESIAN_POINT('Ctrl Pts',(-3.85602456432968,0.783559536724963,
-38.0106150191919));
#17798=CARTESIAN_POINT('Ctrl Pts',(-3.83032724130082,0.900786613951159,
-38.0166886155066));
#17799=CARTESIAN_POINT('Ctrl Pts',(-3.79938525225186,1.01644513131356,-38.0227622118213));
#17800=CARTESIAN_POINT('Ctrl Pts',(-3.76844326320291,1.13210364867596,-38.028835808136));
#17801=CARTESIAN_POINT('Ctrl Pts',(-3.73225681506575,1.24619316832321,-38.0349094044507));
#17802=CARTESIAN_POINT('Ctrl Pts',(-3.69103343471819,1.35821985841484,-38.0409830007653));
#17803=CARTESIAN_POINT('Ctrl Pts',(-3.65108579019771,1.46677966973685,-38.0468686381026));
#17804=CARTESIAN_POINT('Ctrl Pts',(-3.60628128121676,1.57374793813777,-38.0527542754398));
#17805=CARTESIAN_POINT('Ctrl Pts',(-3.55676669598073,1.67866008183978,-38.058639912777));
#17806=CARTESIAN_POINT('Ctrl Pts',(-3.50731417562142,1.78344072167815,-38.0645181726646));
#17807=CARTESIAN_POINT('Ctrl Pts',(-3.45316349549236,1.8861699941896,-38.0703964325523));
#17808=CARTESIAN_POINT('Ctrl Pts',(-3.39451045820645,1.98640070205561,-38.0762746924399));
#17809=CARTESIAN_POINT('Ctrl Pts',(-3.33591546662906,2.08653221706269,-38.0821471349347));
#17810=CARTESIAN_POINT('Ctrl Pts',(-3.27282718839415,2.18416973356207,-38.0880195774295));
#17811=CARTESIAN_POINT('Ctrl Pts',(-3.20548825147931,2.27888877956519,-38.0938920199243));
#17812=CARTESIAN_POINT('Ctrl Pts',(-3.13732024435269,2.37477399692662,-38.0998367633398));
#17813=CARTESIAN_POINT('Ctrl Pts',(-3.06479638493153,2.46766800685349,-38.1057815067554));
#17814=CARTESIAN_POINT('Ctrl Pts',(-2.98821500532626,2.55715859538336,-38.111726250171));
#17815=CARTESIAN_POINT('Ctrl Pts',(-2.91264702878933,2.64546495300133,-38.1175923266671));
#17816=CARTESIAN_POINT('Ctrl Pts',(-2.83312855279008,2.73045710576944,-38.1234584031633));
#17817=CARTESIAN_POINT('Ctrl Pts',(-2.74998758315251,2.81177120201964,-38.1293244796594));
#17818=CARTESIAN_POINT('Ctrl Pts',(-2.66685785092488,2.8930743077818,-38.1351897632913));
#17819=CARTESIAN_POINT('Ctrl Pts',(-2.58010689268395,2.97070005836383,-38.1410550469231));
#17820=CARTESIAN_POINT('Ctrl Pts',(-2.49009961654933,3.0443214185859,-38.146920330555));
#17821=CARTESIAN_POINT('Ctrl Pts',(-2.40008300349067,3.11795041593551,-38.1527862226233));
#17822=CARTESIAN_POINT('Ctrl Pts',(-2.30680971925093,3.18757393686283,-38.1586521146916));
#17823=CARTESIAN_POINT('Ctrl Pts',(-2.21067724698488,3.2529056410636,-38.1645180067599));
#17824=CARTESIAN_POINT('Ctrl Pts',(-2.11228160719673,3.31977539570273,-38.170521994688));
#17825=CARTESIAN_POINT('Ctrl Pts',(-2.01089084058811,3.38214846478323,-38.1765259826162));
#17826=CARTESIAN_POINT('Ctrl Pts',(-1.90696084634371,3.43976588309612,-38.1825299705443));
#17827=CARTESIAN_POINT('Ctrl Pts',(-1.80527349143156,3.4961400117363,-38.1884044022306));
#17828=CARTESIAN_POINT('Ctrl Pts',(-1.70115578424155,3.54796152023605,-38.1942788339168));
#17829=CARTESIAN_POINT('Ctrl Pts',(-1.59505694251843,3.59503579260677,-38.200153265603));
#17830=CARTESIAN_POINT('Ctrl Pts',(-1.48544820368334,3.64366734731872,-38.2062220316521));
#17831=CARTESIAN_POINT('Ctrl Pts',(-1.37372543203458,3.68723195741313,-38.2122907977013));
#17832=CARTESIAN_POINT('Ctrl Pts',(-1.26040190601216,3.72557056507066,-38.2183595637504));
#17833=CARTESIAN_POINT('Ctrl Pts',(-1.14707837998975,3.76390917272819,-38.2244283297995));
#17834=CARTESIAN_POINT('Ctrl Pts',(-1.03215457570478,3.79702170740404,-38.2304970958486));
#17835=CARTESIAN_POINT('Ctrl Pts',(-0.916155051025256,3.82480704382338,
-38.2365658618977));
#17836=CARTESIAN_POINT('Ctrl Pts',(-0.803651685067322,3.85175494624009,
-38.2424517188409));
#17837=CARTESIAN_POINT('Ctrl Pts',(-0.689780227077975,3.87377753991593,
-38.248337575784));
#17838=CARTESIAN_POINT('Ctrl Pts',(-0.575008792492617,3.89073950407325,
-38.2542234327272));
#17839=CARTESIAN_POINT('Ctrl Pts',(-0.460380857323033,3.90768026058465,
-38.260101930548));
#17840=CARTESIAN_POINT('Ctrl Pts',(-0.344855586843771,3.91957291266557,
-38.2659804283687));
#17841=CARTESIAN_POINT('Ctrl Pts',(-0.228913789094253,3.9263325734281,-38.2718589261895));
#17842=CARTESIAN_POINT('Ctrl Pts',(-0.113086377458502,3.93308556522965,
-38.277731624389));
#17843=CARTESIAN_POINT('Ctrl Pts',(0.00315633580555784,3.93471561623088,
-38.2836043225884));
#17844=CARTESIAN_POINT('Ctrl Pts',(0.119326508151583,3.93118941091018,-38.2894770207879));
#17845=CARTESIAN_POINT('Ctrl Pts',(0.2369200718725,3.92762000026287,-38.295421675048));
#17846=CARTESIAN_POINT('Ctrl Pts',(0.354438882306982,3.91876706389708,-38.3013663293081));
#17847=CARTESIAN_POINT('Ctrl Pts',(0.471374519808667,3.904650440446,-38.3073109835682));
#17848=CARTESIAN_POINT('Ctrl Pts',(0.586770322034666,3.89071970792798,-38.3131773572585));
#17849=CARTESIAN_POINT('Ctrl Pts',(0.701597799363148,3.87166314337651,-38.3190437309488));
#17850=CARTESIAN_POINT('Ctrl Pts',(0.815372247446922,3.84755209166729,-38.3249101046391));
#17851=CARTESIAN_POINT('Ctrl Pts',(0.929131607419284,3.82344423742675,-38.3307757003648));
#17852=CARTESIAN_POINT('Ctrl Pts',(1.041837813855,3.79428331435358,-38.3366412960904));
#17853=CARTESIAN_POINT('Ctrl Pts',(1.15301635419074,3.76019178858854,-38.3425068918161));
#17854=CARTESIAN_POINT('Ctrl Pts',(1.2642067012028,3.72609664245208,-38.3483731104424));
#17855=CARTESIAN_POINT('Ctrl Pts',(1.37386866660868,3.68706997321528,-38.3542393290688));
#17856=CARTESIAN_POINT('Ctrl Pts',(1.48154355541025,3.64328391611501,-38.3601055476951));
#17857=CARTESIAN_POINT('Ctrl Pts',(1.59174005204084,3.59847244570237,-38.3661091456397));
#17858=CARTESIAN_POINT('Ctrl Pts',(1.69985482087368,3.54867605575534,-38.3721127435843));
#17859=CARTESIAN_POINT('Ctrl Pts',(1.80541974179486,3.49413058656046,-38.3781163415289));
#17860=CARTESIAN_POINT('Ctrl Pts',(1.90871976619197,3.44075539099915,-38.3839911322144));
#17861=CARTESIAN_POINT('Ctrl Pts',(2.00957792592519,3.38283310951248,-38.3898659228999));
#17862=CARTESIAN_POINT('Ctrl Pts',(2.10758319170174,3.32062977310876,-38.3957407135854));
#17863=CARTESIAN_POINT('Ctrl Pts',(2.20881166754664,3.25638068519777,-38.4018087151595));
#17864=CARTESIAN_POINT('Ctrl Pts',(2.30699596806504,3.18756437599956,-38.4078767167337));
#17865=CARTESIAN_POINT('Ctrl Pts',(2.40171937904222,3.11451971005692,-38.4139447183078));
#17866=CARTESIAN_POINT('Ctrl Pts',(2.49644279001939,3.04147504411429,-38.4200127198819));
#17867=CARTESIAN_POINT('Ctrl Pts',(2.5877049892177,2.96420237824787,-38.426080721456));
#17868=CARTESIAN_POINT('Ctrl Pts',(2.67513119754383,2.88308204460569,-38.4321487230301));
#17869=CARTESIAN_POINT('Ctrl Pts',(2.75860512206978,2.8056289245675,-38.4379424079573));
#17870=CARTESIAN_POINT('Ctrl Pts',(2.83886598245247,2.72440488468828,-38.4437360928845));
#17871=CARTESIAN_POINT('Ctrl Pts',(2.91554707754647,2.63971101422301,-38.4495297778117));
#17872=CARTESIAN_POINT('Ctrl Pts',(2.99213073461557,2.55512476354914,-38.455316100752));
#17873=CARTESIAN_POINT('Ctrl Pts',(3.06514338501152,2.46707775853196,-38.4611024236923));
#17874=CARTESIAN_POINT('Ctrl Pts',(3.13425271576831,2.37591012323677,-38.4668887466326));
#17875=CARTESIAN_POINT('Ctrl Pts',(3.20328640624917,2.28484227106803,-38.472668736433));
#17876=CARTESIAN_POINT('Ctrl Pts',(3.26842502046197,2.19066092033031,-38.4784487262333));
#17877=CARTESIAN_POINT('Ctrl Pts',(3.32937499763355,2.09374094031057,-38.4842287160337));
#17878=CARTESIAN_POINT('Ctrl Pts',(3.39028834502291,1.9968792073637,-38.4900052321696));
#17879=CARTESIAN_POINT('Ctrl Pts',(3.44701783152,1.89728247437855,-38.4957817483056));
#17880=CARTESIAN_POINT('Ctrl Pts',(3.49931221790545,1.79535595401514,-38.5015582644415));
#17881=CARTESIAN_POINT('Ctrl Pts',(3.55158863562845,1.69346445621088,-38.5073327957321));
#17882=CARTESIAN_POINT('Ctrl Pts',(3.59943278871211,1.58924514041807,-38.5131073270227));
#17883=CARTESIAN_POINT('Ctrl Pts',(3.64263899416319,1.4831285036037,-38.5188818583133));
#17884=CARTESIAN_POINT('Ctrl Pts',(3.68584147265992,1.37702102037868,-38.5246558914945));
#17885=CARTESIAN_POINT('Ctrl Pts',(3.72440664034969,1.26901693610166,-38.5304299246758));
#17886=CARTESIAN_POINT('Ctrl Pts',(3.75817698400003,1.15956662461992,-38.536203957857));
#17887=CARTESIAN_POINT('Ctrl Pts',(3.79196743080534,1.05005115843927,-38.5419814282637));
#17888=CARTESIAN_POINT('Ctrl Pts',(3.8209572275429,0.939088152567181,-38.5477588986704));
#17889=CARTESIAN_POINT('Ctrl Pts',(3.84503885974989,0.827142773052661,-38.5535363690771));
#17890=CARTESIAN_POINT('Ctrl Pts',(3.86912863085394,0.715159559228866,-38.5593157921021));
#17891=CARTESIAN_POINT('Ctrl Pts',(3.88830686104604,0.602193729592473,-38.5650952151271));
#17892=CARTESIAN_POINT('Ctrl Pts',(3.90251752942964,0.488718663951327,-38.5708746381522));
#17893=CARTESIAN_POINT('Ctrl Pts',(3.91674398053681,0.375117570065492,-38.5766604799489));
#17894=CARTESIAN_POINT('Ctrl Pts',(3.92599182103187,0.261006534640592,-38.5824463217456));
#17895=CARTESIAN_POINT('Ctrl Pts',(3.93025706314013,0.146861899882653,-38.5882321635423));
#17896=CARTESIAN_POINT('Ctrl Pts',(3.9321256614196,0.0968552501530872,-38.5907669350166));
#17897=CARTESIAN_POINT('Ctrl Pts',(3.93303862096152,0.0468421311809369,
-38.5933017064908));
#17898=CARTESIAN_POINT('Ctrl Pts',(3.93299874843716,-0.00313764111372402,
-38.595836477965));
#17899=CARTESIAN_POINT('Origin',(0.,0.,-41.3107734492731));
#17900=CARTESIAN_POINT('',(-0.0655702737400695,-3.22208288250033,-31.));
#17901=CARTESIAN_POINT('Ctrl Pts',(2.26878022305635,-2.28883242330415,-32.0941031001172));
#17902=CARTESIAN_POINT('Ctrl Pts',(2.30269587212703,-2.25521390537326,-32.0913860187157));
#17903=CARTESIAN_POINT('Ctrl Pts',(2.3358768770722,-2.22082908129709,-32.0886515262801));
#17904=CARTESIAN_POINT('Ctrl Pts',(2.42800183076779,-2.12100791224114,-32.080811535697));
#17905=CARTESIAN_POINT('Ctrl Pts',(2.48502712952621,-2.05390013857292,-32.075654741596));
#17906=CARTESIAN_POINT('Ctrl Pts',(2.56922013911977,-1.94617499834573,-32.0674804372658));
#17907=CARTESIAN_POINT('Ctrl Pts',(2.59833431977136,-1.90713073244486,-32.0645377956117));
#17908=CARTESIAN_POINT('Ctrl Pts',(2.65220736995442,-1.83135850178335,-32.0588554205981));
#17909=CARTESIAN_POINT('Ctrl Pts',(2.67711578430642,-1.79475030915057,-32.0561221581938));
#17910=CARTESIAN_POINT('Ctrl Pts',(2.73439706965908,-1.7067166145575,-32.0495718775103));
#17911=CARTESIAN_POINT('Ctrl Pts',(2.76608429868254,-1.65486731084621,-32.0457314351963));
#17912=CARTESIAN_POINT('Ctrl Pts',(2.88793183107832,-1.44220356192964,-32.0300387521813));
#17913=CARTESIAN_POINT('Ctrl Pts',(2.96567304885764,-1.27470322518631,-32.0177849534717));
#17914=CARTESIAN_POINT('Ctrl Pts',(3.09331620330717,-0.92373781956942,-31.9926617500646));
#17915=CARTESIAN_POINT('Ctrl Pts',(3.14219487871066,-0.740619039081715,
-31.9798357952823));
#17916=CARTESIAN_POINT('Ctrl Pts',(3.18160946083803,-0.514858005776426,
-31.9650076082526));
#17917=CARTESIAN_POINT('Ctrl Pts',(3.187754919486,-0.47532770888958,-31.9624479761529));
#17918=CARTESIAN_POINT('Ctrl Pts',(3.1965876061699,-0.410593318744866,-31.9583269425027));
#17919=CARTESIAN_POINT('Ctrl Pts',(3.19971625413538,-0.385454612938542,
-31.9567440216313));
#17920=CARTESIAN_POINT('Ctrl Pts',(3.20580697930199,-0.331313765153808,
-31.9533751303039));
#17921=CARTESIAN_POINT('Ctrl Pts',(3.20867257801835,-0.302303866281698,
-31.9515940349341));
#17922=CARTESIAN_POINT('Ctrl Pts',(3.2162103680128,-0.213724791241191,-31.946218100288));
#17923=CARTESIAN_POINT('Ctrl Pts',(3.21962021866489,-0.154058392539949,
-31.942682792648));
#17924=CARTESIAN_POINT('Ctrl Pts',(3.22399641357307,-0.00460818804654803,
-31.933967563008));
#17925=CARTESIAN_POINT('Ctrl Pts',(3.22287433168171,0.0851871518327197,
-31.9288565421208));
#17926=CARTESIAN_POINT('Ctrl Pts',(3.2046632018971,0.420403909893013,-31.9098902301207));
#17927=CARTESIAN_POINT('Ctrl Pts',(3.16325636419336,0.663632865041635,-31.8962881436646));
#17928=CARTESIAN_POINT('Ctrl Pts',(3.07709233789193,0.959973655136131,-31.8781473582528));
#17929=CARTESIAN_POINT('Ctrl Pts',(3.05784011597213,1.0196370668197,-31.8744161814322));
#17930=CARTESIAN_POINT('Ctrl Pts',(3.0219427872718,1.12069886589051,-31.8679379879319));
#17931=CARTESIAN_POINT('Ctrl Pts',(3.00615508434449,1.16238352830986,-31.8652188469219));
#17932=CARTESIAN_POINT('Ctrl Pts',(2.97156368826825,1.24829285180367,-31.8595096973298));
#17933=CARTESIAN_POINT('Ctrl Pts',(2.95262524849007,1.29245098684563,-31.8565158170679));
#17934=CARTESIAN_POINT('Ctrl Pts',(2.89794265830359,1.41247190050719,-31.8482076961596));
#17935=CARTESIAN_POINT('Ctrl Pts',(2.86021568274914,1.4873845560476,-31.8428297275885));
#17936=CARTESIAN_POINT('Ctrl Pts',(2.76453808458551,1.660234932916,-31.8299589198227));
#17937=CARTESIAN_POINT('Ctrl Pts',(2.7042386826883,1.75674145185515,-31.8224025883023));
#17938=CARTESIAN_POINT('Ctrl Pts',(2.51835046277141,2.02192649814793,-31.8006806392809));
#17939=CARTESIAN_POINT('Ctrl Pts',(2.38118727065392,2.18179513333603,-31.7863673364536));
#17940=CARTESIAN_POINT('Ctrl Pts',(2.19910212015222,2.35623250327597,-31.7700197899927));
#17941=CARTESIAN_POINT('Ctrl Pts',(2.16820519540113,2.38469460311477,-31.7673272032451));
#17942=CARTESIAN_POINT('Ctrl Pts',(2.1192441238804,2.42805875671053,-31.7631965030385));
#17943=CARTESIAN_POINT('Ctrl Pts',(2.10155990629271,2.44338106947639,-31.7617312102999));
#17944=CARTESIAN_POINT('Ctrl Pts',(2.062636805982,2.4763703300216,-31.7585665859691));
#17945=CARTESIAN_POINT('Ctrl Pts',(2.04133452434316,2.49395951995371,-31.7568726621206));
#17946=CARTESIAN_POINT('Ctrl Pts',(1.98016617939621,2.54315699397321,-31.7521071192955));
#17947=CARTESIAN_POINT('Ctrl Pts',(1.93977274742268,2.57409943223772,-31.7490763838719));
#17948=CARTESIAN_POINT('Ctrl Pts',(1.68799945715152,2.75767031803509,-31.7307714439952));
#17949=CARTESIAN_POINT('Ctrl Pts',(1.45946248703766,2.88514861247454,-31.716552284361));
#17950=CARTESIAN_POINT('Ctrl Pts',(1.11508615136928,3.02573419869209,-31.6953322758645));
#17951=CARTESIAN_POINT('Ctrl Pts',(1.01002941456809,3.06240460224482,-31.6888950791099));
#17952=CARTESIAN_POINT('Ctrl Pts',(0.851906628966527,3.10857498452044,-31.6791138783058));
#17953=CARTESIAN_POINT('Ctrl Pts',(0.800155972205574,3.12229615346054,-31.6758990856793));
#17954=CARTESIAN_POINT('Ctrl Pts',(0.705447768261373,3.14489791590229,-31.6699781646605));
#17955=CARTESIAN_POINT('Ctrl Pts',(0.662604332069828,3.15420269890428,-31.6672859744977));
#17956=CARTESIAN_POINT('Ctrl Pts',(0.566881153817695,3.17295567740038,-31.6612346210127));
#17957=CARTESIAN_POINT('Ctrl Pts',(0.513929102191623,3.18196139420478,-31.6578626683127));
#17958=CARTESIAN_POINT('Ctrl Pts',(0.338186920964142,3.20734931902271,-31.6465827152656));
#17959=CARTESIAN_POINT('Ctrl Pts',(0.214688733257574,3.21797498435541,-31.6385086451206));
#17960=CARTESIAN_POINT('Ctrl Pts',(-0.164398127653997,3.22867126088657,
-31.6133465045129));
#17961=CARTESIAN_POINT('Ctrl Pts',(-0.419630197333096,3.20550307952549,
-31.5958110542406));
#17962=CARTESIAN_POINT('Ctrl Pts',(-0.715661544293251,3.14263875912357,
-31.5760935929661));
#17963=CARTESIAN_POINT('Ctrl Pts',(-0.761659009348888,3.13180872361144,
-31.573051191581));
#17964=CARTESIAN_POINT('Ctrl Pts',(-0.833431711139318,3.11323496455642,
-31.5683542780195));
#17965=CARTESIAN_POINT('Ctrl Pts',(-0.859374979166682,3.10617371097775,
-31.5666669691321));
#17966=CARTESIAN_POINT('Ctrl Pts',(-0.911158601851891,3.09138073372402,
-31.5633241894602));
#17967=CARTESIAN_POINT('Ctrl Pts',(-0.936996283277776,3.08364766297524,
-31.5616690316654));
#17968=CARTESIAN_POINT('Ctrl Pts',(-1.00880741785217,3.06116903065983,-31.5570967016156));
#17969=CARTESIAN_POINT('Ctrl Pts',(-1.05455284652535,3.0457128996373,-31.5542161352676));
#17970=CARTESIAN_POINT('Ctrl Pts',(-1.32227346001728,2.94850165182541,-31.5374550333712));
#17971=CARTESIAN_POINT('Ctrl Pts',(-1.53506666740538,2.84352973759563,-31.5244859336924));
#17972=CARTESIAN_POINT('Ctrl Pts',(-1.8486230714047,2.64330393188778,-31.503442160978));
#17973=CARTESIAN_POINT('Ctrl Pts',(-1.95805997802934,2.5632906514834,-31.4956768753677));
#17974=CARTESIAN_POINT('Ctrl Pts',(-2.10495182836704,2.4409833879626,-31.4843667723144));
#17975=CARTESIAN_POINT('Ctrl Pts',(-2.14683672580388,2.40422828016424,-31.481031037112));
#17976=CARTESIAN_POINT('Ctrl Pts',(-2.21973917301845,2.33682989497028,-31.4750084337969));
#17977=CARTESIAN_POINT('Ctrl Pts',(-2.25112785249876,2.30660769562419,-31.4723393004983));
#17978=CARTESIAN_POINT('Ctrl Pts',(-2.317892180431,2.23966342732664,-31.4664879098487));
#17979=CARTESIAN_POINT('Ctrl Pts',(-2.35302801223078,2.202719940847,-31.4632964038722));
#17980=CARTESIAN_POINT('Ctrl Pts',(-2.45722597128624,2.0878223097116,-31.4534750989155));
#17981=CARTESIAN_POINT('Ctrl Pts',(-2.52339422669504,2.00734636645594,-31.4467340633678));
#17982=CARTESIAN_POINT('Ctrl Pts',(-2.68520786206053,1.78987402617002,-31.4288816559198));
#17983=CARTESIAN_POINT('Ctrl Pts',(-2.77430483842334,1.648397997535,-31.4176029251084));
#17984=CARTESIAN_POINT('Ctrl Pts',(-2.91043134972012,1.38968839206108,-31.397928445544));
#17985=CARTESIAN_POINT('Ctrl Pts',(-2.96230373536414,1.27538452830868,-31.389534996897));
#17986=CARTESIAN_POINT('Ctrl Pts',(-3.02236140857858,1.11945758137157,-31.3787011399939));
#17987=CARTESIAN_POINT('Ctrl Pts',(-3.03658318505253,1.08028546676466,-31.3760297322998));
#17988=CARTESIAN_POINT('Ctrl Pts',(-3.05755513936169,1.01883035529114,-31.3719281059413));
#17989=CARTESIAN_POINT('Ctrl Pts',(-3.06483007944046,0.996732371151817,
-31.3704710348326));
#17990=CARTESIAN_POINT('Ctrl Pts',(-3.08019773835946,0.948292502860615,
-31.367318589169));
#17991=CARTESIAN_POINT('Ctrl Pts',(-3.08819316807161,0.921921828038814,
-31.3656286564869));
#17992=CARTESIAN_POINT('Ctrl Pts',(-3.10991403963639,0.846826073182173,
-31.3608820573509));
#17993=CARTESIAN_POINT('Ctrl Pts',(-3.12283166864551,0.797873862074177,
-31.3578658852015));
#17994=CARTESIAN_POINT('Ctrl Pts',(-3.15080775411709,0.68073585731148,-31.3507895851501));
#17995=CARTESIAN_POINT('Ctrl Pts',(-3.16481450273892,0.61232424050743,-31.3467688140367));
#17996=CARTESIAN_POINT('Ctrl Pts',(-3.19910731805787,0.411896488304255,
-31.3351797423718));
#17997=CARTESIAN_POINT('Ctrl Pts',(-3.21342524759083,0.279009445096801,
-31.3277297440384));
#17998=CARTESIAN_POINT('Ctrl Pts',(-3.22617513392283,-0.00288311090345444,
-31.3118281237634));
#17999=CARTESIAN_POINT('Ctrl Pts',(-3.22260910205966,-0.151655446097844,
-31.3033745228977));
#18000=CARTESIAN_POINT('Ctrl Pts',(-3.20296404878469,-0.362028737096515,
-31.2909499679528));
#18001=CARTESIAN_POINT('Ctrl Pts',(-3.19532051171561,-0.424228219590455,
-31.2872189729755));
#18002=CARTESIAN_POINT('Ctrl Pts',(-3.17912239871893,-0.530375980310534,
-31.2807310808168));
#18003=CARTESIAN_POINT('Ctrl Pts',(-3.17145607016934,-0.574442338233476,
-31.2780017416837));
#18004=CARTESIAN_POINT('Ctrl Pts',(-3.15359270007901,-0.665816384975227,
-31.2722606617297));
#18005=CARTESIAN_POINT('Ctrl Pts',(-3.14324221796188,-0.713082283954703,
-31.2692448158096));
#18006=CARTESIAN_POINT('Ctrl Pts',(-3.11176594421387,-0.842774434622913,
-31.2608354659203));
#18007=CARTESIAN_POINT('Ctrl Pts',(-3.08843516383748,-0.924620061884636,
-31.2553763052914));
#18008=CARTESIAN_POINT('Ctrl Pts',(-3.02558624848566,-1.11601539650809,
-31.2422465991681));
#18009=CARTESIAN_POINT('Ctrl Pts',(-2.98331645446263,-1.2245333145831,-31.2345092128059));
#18010=CARTESIAN_POINT('Ctrl Pts',(-2.84683434058708,-1.52562782989232,
-31.2123349254712));
#18011=CARTESIAN_POINT('Ctrl Pts',(-2.73915864165989,-1.71143953051354,
-31.1977602821704));
#18012=CARTESIAN_POINT('Ctrl Pts',(-2.59200322478139,-1.91547121703878,
-31.1815462251745));
#18013=CARTESIAN_POINT('Ctrl Pts',(-2.56964415841414,-1.94536368647978,
-31.179166091185));
#18014=CARTESIAN_POINT('Ctrl Pts',(-2.53109526381668,-1.99507609176752,
-31.1752088826466));
#18015=CARTESIAN_POINT('Ctrl Pts',(-2.51518061578726,-2.01510259144709,
-31.1736154309618));
#18016=CARTESIAN_POINT('Ctrl Pts',(-2.47892010326292,-2.05963267355287,
-31.1700746107593));
#18017=CARTESIAN_POINT('Ctrl Pts',(-2.45844685070412,-2.08402756333465,
-31.168135528056));
#18018=CARTESIAN_POINT('Ctrl Pts',(-2.38849551672843,-2.16491228950299,
-31.1616931827404));
#18019=CARTESIAN_POINT('Ctrl Pts',(-2.33740288336412,-2.21997870014927,
-31.1572851492136));
#18020=CARTESIAN_POINT('Ctrl Pts',(-2.19097751449322,-2.3671265401398,-31.1452814776906));
#18021=CARTESIAN_POINT('Ctrl Pts',(-2.09181904310293,-2.45519179676638,
-31.1378321512879));
#18022=CARTESIAN_POINT('Ctrl Pts',(-1.85325953013115,-2.64208918767056,
-31.1207230777363));
#18023=CARTESIAN_POINT('Ctrl Pts',(-1.71087525839875,-2.7364402932757,-31.1110608474382));
#18024=CARTESIAN_POINT('Ctrl Pts',(-1.50651259155632,-2.84965223764059,
-31.0973114263493));
#18025=CARTESIAN_POINT('Ctrl Pts',(-1.45044094734478,-2.87859659783319,
-31.093552525306));
#18026=CARTESIAN_POINT('Ctrl Pts',(-1.35288614956159,-2.92538054189175,
-31.0870124948111));
#18027=CARTESIAN_POINT('Ctrl Pts',(-1.31181042617959,-2.94402876150796,
-31.084258834697));
#18028=CARTESIAN_POINT('Ctrl Pts',(-1.22533804724394,-2.9811178989734,-31.078454839349));
#18029=CARTESIAN_POINT('Ctrl Pts',(-1.17988536754214,-2.99939783501842,
-31.0754001215773));
#18030=CARTESIAN_POINT('Ctrl Pts',(-1.05268546505144,-3.04721577114661,
-31.0668333619798));
#18031=CARTESIAN_POINT('Ctrl Pts',(-0.97013804256901,-3.07449193760006,
-31.0612525060389));
#18032=CARTESIAN_POINT('Ctrl Pts',(-0.771583036524189,-3.13130771240993,
-31.0477775922899));
#18033=CARTESIAN_POINT('Ctrl Pts',(-0.654836372250052,-3.15778621998811,
-31.0398119698717));
#18034=CARTESIAN_POINT('Ctrl Pts',(-0.381070158534853,-3.2040408954779,
-31.0211616860773));
#18035=CARTESIAN_POINT('Ctrl Pts',(-0.223536725865423,-3.21886822170937,
-31.0104465088182));
#18036=CARTESIAN_POINT('Ctrl Pts',(-0.0655702737400695,-3.22208288250033,
-31.));
#18037=CARTESIAN_POINT('',(-3.05625919777041,-1.02244671183577,-31.));
#18038=CARTESIAN_POINT('Origin',(0.,0.,-31.));
#18039=CARTESIAN_POINT('Ctrl Pts',(-3.05625919777041,-1.02244671183577,
-31.));
#18040=CARTESIAN_POINT('Ctrl Pts',(-3.06368966725375,-1.00023583234511,
-31.0014457916658));
#18041=CARTESIAN_POINT('Ctrl Pts',(-3.07087800392366,-0.977943988332985,
-31.002880504093));
#18042=CARTESIAN_POINT('Ctrl Pts',(-3.08701830394628,-0.925957511541264,
-31.0061922236022));
#18043=CARTESIAN_POINT('Ctrl Pts',(-3.09578601304777,-0.896207788930303,
-31.0080617128447));
#18044=CARTESIAN_POINT('Ctrl Pts',(-3.1589685710295,-0.66982147584979,-31.0221223008988));
#18045=CARTESIAN_POINT('Ctrl Pts',(-3.19503326635304,-0.468528200778728,
-31.0336998688189));
#18046=CARTESIAN_POINT('Ctrl Pts',(-3.22382371044213,-0.119802007364771,
-31.0538520637253));
#18047=CARTESIAN_POINT('Ctrl Pts',(-3.225941836979,0.0261969329579913,-31.0623149907551));
#18048=CARTESIAN_POINT('Ctrl Pts',(-3.2150766966268,0.229687745429387,-31.0744904123262));
#18049=CARTESIAN_POINT('Ctrl Pts',(-3.21042786623023,0.287449115648635,
-31.0779882507207));
#18050=CARTESIAN_POINT('Ctrl Pts',(-3.1990117194526,0.39346197962638,-31.0845041375768));
#18051=CARTESIAN_POINT('Ctrl Pts',(-3.19270235691127,0.441746090229753,
-31.0875087640725));
#18052=CARTESIAN_POINT('Ctrl Pts',(-3.17598813756868,0.55042832070649,-31.0943654185429));
#18053=CARTESIAN_POINT('Ctrl Pts',(-3.16494966697735,0.610708475448756,
-31.0982344076252));
#18054=CARTESIAN_POINT('Ctrl Pts',(-3.11743162289897,0.834058741912733,
-31.1128358535922));
#18055=CARTESIAN_POINT('Ctrl Pts',(-3.07001141816015,0.994510294080951,
-31.1238758879573));
#18056=CARTESIAN_POINT('Ctrl Pts',(-2.94714504766617,1.31598743195748,-31.1470409037298));
#18057=CARTESIAN_POINT('Ctrl Pts',(-2.87038463933554,1.4759330295311,-31.1591527075447));
#18058=CARTESIAN_POINT('Ctrl Pts',(-2.74962979707509,1.68210439534145,-31.1751409476614));
#18059=CARTESIAN_POINT('Ctrl Pts',(-2.71685642060489,1.73454063375296,-31.1792406023768));
#18060=CARTESIAN_POINT('Ctrl Pts',(-2.65662281659608,1.82501201368435,-31.186337945505));
#18061=CARTESIAN_POINT('Ctrl Pts',(-2.62980306552993,1.86345109653001,-31.1893613441493));
#18062=CARTESIAN_POINT('Ctrl Pts',(-2.58623635035271,1.9230774748852,-31.1940486022615));
#18063=CARTESIAN_POINT('Ctrl Pts',(-2.57004619167942,1.94466144229419,-31.195744757829));
#18064=CARTESIAN_POINT('Ctrl Pts',(-2.53956426353007,1.98425281189865,-31.1988513756385));
#18065=CARTESIAN_POINT('Ctrl Pts',(-2.52534787880142,2.00231465682156,-31.2002664296262));
#18066=CARTESIAN_POINT('Ctrl Pts',(-2.48449699589171,2.05308829189956,-31.2042423177796));
#18067=CARTESIAN_POINT('Ctrl Pts',(-2.45741070761794,2.0854327744636,-31.2067730287731));
#18068=CARTESIAN_POINT('Ctrl Pts',(-2.29511517705172,2.27167957011959,-31.2213978453259));
#18069=CARTESIAN_POINT('Ctrl Pts',(-2.14610099964124,2.41295476041724,-31.2327303683791));
#18070=CARTESIAN_POINT('Ctrl Pts',(-1.86011285301185,2.63649192477108,-31.2531034964869));
#18071=CARTESIAN_POINT('Ctrl Pts',(-1.728572126257,2.72454428744957,-31.2620448358675));
#18072=CARTESIAN_POINT('Ctrl Pts',(-1.53847462413816,2.83246837849274,-31.274878888015));
#18073=CARTESIAN_POINT('Ctrl Pts',(-1.48500867909494,2.86086172410591,-31.2784777954861));
#18074=CARTESIAN_POINT('Ctrl Pts',(-1.39258807477507,2.90665313853114,-31.2847013887399));
#18075=CARTESIAN_POINT('Ctrl Pts',(-1.35402868087581,2.9248145364131,-31.2872986236609));
#18076=CARTESIAN_POINT('Ctrl Pts',(-1.27376644301661,2.96069055920054,-31.2927122448261));
#18077=CARTESIAN_POINT('Ctrl Pts',(-1.23202769743837,2.97830101775068,-31.2955315294312));
#18078=CARTESIAN_POINT('Ctrl Pts',(-1.11916203578566,3.02314291374768,-31.3031718607527));
#18079=CARTESIAN_POINT('Ctrl Pts',(-1.04742167105526,3.04874121795445,-31.3080463126545));
#18080=CARTESIAN_POINT('Ctrl Pts',(-0.722510290549048,3.15185389725355,
-31.330210741756));
#18081=CARTESIAN_POINT('Ctrl Pts',(-0.46128815079424,3.20052802961832,-31.3483791259836));
#18082=CARTESIAN_POINT('Ctrl Pts',(-0.127446697404474,3.22098540369439,
-31.3708753888323));
#18083=CARTESIAN_POINT('Ctrl Pts',(-0.0576529010695713,3.22299035606959,
-31.3755313199506));
#18084=CARTESIAN_POINT('Ctrl Pts',(0.0623773136828261,3.2225376660785,-31.3834024835212));
#18085=CARTESIAN_POINT('Ctrl Pts',(0.112592210636624,3.22117425371005,-31.386654333067));
#18086=CARTESIAN_POINT('Ctrl Pts',(0.189303426318992,3.21729517610779,-31.3915388576666));
#18087=CARTESIAN_POINT('Ctrl Pts',(0.215833062098524,3.21562440419861,-31.3932127962895));
#18088=CARTESIAN_POINT('Ctrl Pts',(0.268190723828241,3.21167609133527,-31.396482340816));
#18089=CARTESIAN_POINT('Ctrl Pts',(0.294017176982475,3.20941483523529,-31.3980790765947));
#18090=CARTESIAN_POINT('Ctrl Pts',(0.361997564615379,3.20263523238189,-31.4022462306662));
#18091=CARTESIAN_POINT('Ctrl Pts',(0.404095715928131,3.19759623734473,-31.4047904924148));
#18092=CARTESIAN_POINT('Ctrl Pts',(0.60860659234301,3.16901325569792,-31.4170253917112));
#18093=CARTESIAN_POINT('Ctrl Pts',(0.769172918918247,3.13391614655204,-31.4262542217489));
#18094=CARTESIAN_POINT('Ctrl Pts',(1.06241237340047,3.04591024737248,-31.4434607677009));
#18095=CARTESIAN_POINT('Ctrl Pts',(1.19559428055507,2.99613773100335,-31.4514208837747));
#18096=CARTESIAN_POINT('Ctrl Pts',(1.41269034876644,2.89821775327242,-31.4651117496847));
#18097=CARTESIAN_POINT('Ctrl Pts',(1.49850783341695,2.85479108607176,-31.4707228556424));
#18098=CARTESIAN_POINT('Ctrl Pts',(1.62620156623365,2.78282790186384,-31.4794690676037));
#18099=CARTESIAN_POINT('Ctrl Pts',(1.66956217675269,2.75703180770333,-31.4825120780828));
#18100=CARTESIAN_POINT('Ctrl Pts',(1.75017032253303,2.70647739744948,-31.4883189821727));
#18101=CARTESIAN_POINT('Ctrl Pts',(1.78754300763295,2.6819406690684,-31.491074558226));
#18102=CARTESIAN_POINT('Ctrl Pts',(1.87277349881676,2.62341031381723,-31.4975127638752));
#18103=CARTESIAN_POINT('Ctrl Pts',(1.92023587157573,2.58887152363114,-31.5012145268787));
#18104=CARTESIAN_POINT('Ctrl Pts',(2.151877929996,2.41042801712911,-31.5198836809907));
#18105=CARTESIAN_POINT('Ctrl Pts',(2.32094072454142,2.248098242461,-31.5355387515505));
#18106=CARTESIAN_POINT('Ctrl Pts',(2.53282185524368,1.99504928356514,-31.5576717531323));
#18107=CARTESIAN_POINT('Ctrl Pts',(2.59135730808181,1.9184048147051,-31.5641166666995));
#18108=CARTESIAN_POINT('Ctrl Pts',(2.68203956004036,1.7879282463809,-31.5745573751123));
#18109=CARTESIAN_POINT('Ctrl Pts',(2.71620988307163,1.735577282764,-31.5786149286894));
#18110=CARTESIAN_POINT('Ctrl Pts',(2.76448768556705,1.65669074393811,-31.5845030371213));
#18111=CARTESIAN_POINT('Ctrl Pts',(2.77978038810149,1.63090083366546,-31.5863934382334));
#18112=CARTESIAN_POINT('Ctrl Pts',(2.80752340019051,1.5825902181051,-31.5898656822868));
#18113=CARTESIAN_POINT('Ctrl Pts',(2.82006683015137,1.56012901686155,-31.5914523496926));
#18114=CARTESIAN_POINT('Ctrl Pts',(2.85177300000097,1.50172145041604,-31.5955115941272));
#18115=CARTESIAN_POINT('Ctrl Pts',(2.87052556326866,1.46555787469823,-31.5979611657829));
#18116=CARTESIAN_POINT('Ctrl Pts',(2.96951586831282,1.26546487276322,-31.6112206540704));
#18117=CARTESIAN_POINT('Ctrl Pts',(3.03641006742162,1.09528688862761,-31.6214442160957));
#18118=CARTESIAN_POINT('Ctrl Pts',(3.12589044186297,0.795004422728859,-31.6390740870646));
#18119=CARTESIAN_POINT('Ctrl Pts',(3.15557468942645,0.66750968059083,-31.6464383820955));
#18120=CARTESIAN_POINT('Ctrl Pts',(3.19268269695692,0.448581385771919,-31.659241738571));
#18121=CARTESIAN_POINT('Ctrl Pts',(3.20410480734677,0.357992238509676,-31.6645829008062));
#18122=CARTESIAN_POINT('Ctrl Pts',(3.21575888037754,0.217832593882884,-31.6729882330568));
#18123=CARTESIAN_POINT('Ctrl Pts',(3.21871900304368,0.168534277721682,-31.6759710652802));
#18124=CARTESIAN_POINT('Ctrl Pts',(3.2221876273703,0.0748105921557126,-31.6817018316883));
#18125=CARTESIAN_POINT('Ctrl Pts',(3.22291250222038,0.0304044745985394,
-31.6844425394197));
#18126=CARTESIAN_POINT('Ctrl Pts',(3.22245805109125,-0.0742015105409391,
-31.6909645857511));
#18127=CARTESIAN_POINT('Ctrl Pts',(3.22050975858975,-0.134379685467865,
-31.6947681564767));
#18128=CARTESIAN_POINT('Ctrl Pts',(3.20098917367345,-0.45729290420798,-31.7154690395089));
#18129=CARTESIAN_POINT('Ctrl Pts',(3.15295114961931,-0.717150366740733,
-31.7332802961136));
#18130=CARTESIAN_POINT('Ctrl Pts',(3.04863743216703,-1.04832299439081,-31.7566078811022));
#18131=CARTESIAN_POINT('Ctrl Pts',(3.02028215730451,-1.12741666957471,-31.7622183823982));
#18132=CARTESIAN_POINT('Ctrl Pts',(2.96744270566311,-1.2584447131418,-31.7714948272407));
#18133=CARTESIAN_POINT('Ctrl Pts',(2.94460319285558,-1.31099663952812,-31.7752100388339));
#18134=CARTESIAN_POINT('Ctrl Pts',(2.90820949774069,-1.3889788952928,-31.7806870682699));
#18135=CARTESIAN_POINT('Ctrl Pts',(2.8956967382222,-1.41487999232281,-31.7825000701201));
#18136=CARTESIAN_POINT('Ctrl Pts',(2.87147338060518,-1.46335388131127,-31.7858767548139));
#18137=CARTESIAN_POINT('Ctrl Pts',(2.85983970098786,-1.48596126225074,-31.7874442407776));
#18138=CARTESIAN_POINT('Ctrl Pts',(2.82879287135425,-1.54457819228725,-31.7914942835404));
#18139=CARTESIAN_POINT('Ctrl Pts',(2.80895881611487,-1.58036122910465,-31.7939528305251));
#18140=CARTESIAN_POINT('Ctrl Pts',(2.70191715950857,-1.7650918279723,-31.8066229361826));
#18141=CARTESIAN_POINT('Ctrl Pts',(2.60352100332794,-1.90724827281157,-31.8163069293231));
#18142=CARTESIAN_POINT('Ctrl Pts',(2.42340092316841,-2.12738003006174,-31.832286277038));
#18143=CARTESIAN_POINT('Ctrl Pts',(2.34815673343164,-2.21015132447384,-31.8385591031073));
#18144=CARTESIAN_POINT('Ctrl Pts',(2.26878017977789,-2.28883246620346,-31.8449383693487));
#18145=CARTESIAN_POINT('Ctrl Pts',(-0.500000469481151,-0.249903141543597,
-18.9999974608925));
#18146=CARTESIAN_POINT('Ctrl Pts',(-0.499985698708809,-0.249901829883283,
-18.9999972921557));
#18147=CARTESIAN_POINT('Ctrl Pts',(-0.499943925311476,-0.225581277443933,
-18.9999914184955));
#18148=CARTESIAN_POINT('Ctrl Pts',(-0.49990522080778,-0.0968325121338559,
-18.9999912742066));
#18149=CARTESIAN_POINT('Ctrl Pts',(-0.49990535449692,0.0576086556106972,
-18.9999912543048));
#18150=CARTESIAN_POINT('Ctrl Pts',(-0.499924487061938,0.161824257995483,
-18.9999913623149));
#18151=CARTESIAN_POINT('Ctrl Pts',(-0.49995797003322,0.233166202229003,
-18.9999933695672));
#18152=CARTESIAN_POINT('Ctrl Pts',(-0.499985738345136,0.249901825054466,
-18.999997299666));
#18153=CARTESIAN_POINT('Ctrl Pts',(-0.500000469481151,0.249903141543597,
-18.9999974608925));
#18154=CARTESIAN_POINT('Ctrl Pts',(-0.500005798667243,-1.0727321416819,
-18.9999686389119));
#18155=CARTESIAN_POINT('Ctrl Pts',(-0.617767115371394,-1.05838542886533,
-19.0222827327148));
#18156=CARTESIAN_POINT('Ctrl Pts',(-0.961750910786003,-0.9263461965772,
-19.0706508378555));
#18157=CARTESIAN_POINT('Ctrl Pts',(-1.28046409080139,-0.399643500127231,
-19.0718389690549));
#18158=CARTESIAN_POINT('Ctrl Pts',(-1.27936322016631,0.237312703455417,
-19.0720028526044));
#18159=CARTESIAN_POINT('Ctrl Pts',(-1.12181565277689,0.665712549520801,
-19.071113446577));
#18160=CARTESIAN_POINT('Ctrl Pts',(-0.846099392010201,0.968022332176519,
-19.0545842535533));
#18161=CARTESIAN_POINT('Ctrl Pts',(-0.617440729391164,1.05842519205801,
-19.0222208872159));
#18162=CARTESIAN_POINT('Ctrl Pts',(-0.500005798667244,1.0727321416819,-18.9999686389119));
#18163=CARTESIAN_POINT('Ctrl Pts',(-0.374652368818645,-2.49810309995234,
-19.6779209672235));
#18164=CARTESIAN_POINT('Ctrl Pts',(-0.709305686727837,-2.46080605400923,
-19.7142757163881));
#18165=CARTESIAN_POINT('Ctrl Pts',(-1.68368326934235,-2.14240101116334,
-19.7931584654386));
#18166=CARTESIAN_POINT('Ctrl Pts',(-2.57589728694922,-0.923785230808655,
-19.797316584276));
#18167=CARTESIAN_POINT('Ctrl Pts',(-2.57299505475586,0.5493050318438,-19.7976926645488));
#18168=CARTESIAN_POINT('Ctrl Pts',(-2.1316902523392,1.54026532815555,-19.7949687092533));
#18169=CARTESIAN_POINT('Ctrl Pts',(-1.35624613497006,2.24246988768653,-19.767059280983));
#18170=CARTESIAN_POINT('Ctrl Pts',(-0.708378165244041,2.46090942609474,
-19.7141749559621));
#18171=CARTESIAN_POINT('Ctrl Pts',(-0.374652368818646,2.49810309995235,
-19.6779209672235));
#18172=CARTESIAN_POINT('Ctrl Pts',(-0.112199737628206,-3.,-21.0973505959298));
#18173=CARTESIAN_POINT('Ctrl Pts',(-0.545411427143743,-2.98330034061038,
-21.1128737181934));
#18174=CARTESIAN_POINT('Ctrl Pts',(-1.8433426587387,-2.65791691005246,-21.1489665252715));
#18175=CARTESIAN_POINT('Ctrl Pts',(-3.03119195141778,-1.14304648239468,
-21.1569911263128));
#18176=CARTESIAN_POINT('Ctrl Pts',(-3.02358946238589,0.679679924198355,
-21.1570610940823));
#18177=CARTESIAN_POINT('Ctrl Pts',(-2.44325522122211,1.90810624850608,-21.152940585479));
#18178=CARTESIAN_POINT('Ctrl Pts',(-1.40427919869758,2.75990650054913,-21.1369518532818));
#18179=CARTESIAN_POINT('Ctrl Pts',(-0.544210742352787,2.98334662520411,
-21.1128306944771));
#18180=CARTESIAN_POINT('Ctrl Pts',(-0.112199737628208,3.,-21.0973505959298));
#18181=CARTESIAN_POINT('Ctrl Pts',(1.23694807792704E-15,-3.,-21.704163456598));
#18182=CARTESIAN_POINT('Ctrl Pts',(-0.443076803624563,-3.,-21.7109905340956));
#18183=CARTESIAN_POINT('Ctrl Pts',(-1.79348272300302,-2.70799641386265,
-21.7291868478869));
#18184=CARTESIAN_POINT('Ctrl Pts',(-3.03256791313562,-1.16243137143974,
-21.7388525256077));
#18185=CARTESIAN_POINT('Ctrl Pts',(-3.02252425451967,0.691565714094212,
-21.7387856518469));
#18186=CARTESIAN_POINT('Ctrl Pts',(-2.42127475768073,1.9426253115599,-21.7340800035291));
#18187=CARTESIAN_POINT('Ctrl Pts',(-1.33503228345836,2.79906518555955,-21.7230542680391));
#18188=CARTESIAN_POINT('Ctrl Pts',(-0.441848776791001,3.,-21.7109716122421));
#18189=CARTESIAN_POINT('Ctrl Pts',(-1.51085184250722E-15,3.,-21.704163456598));
#18190=CARTESIAN_POINT('',(-0.500000234886957,0.250003172328595,-18.999998729662));
#18191=CARTESIAN_POINT('',(-0.499951156893989,2.95746669263463,-21.7115242851505));
#18192=CARTESIAN_POINT('Ctrl Pts',(-0.500000469773915,0.250006344657191,
-18.9999974593239));
#18193=CARTESIAN_POINT('Ctrl Pts',(-0.500000469773915,0.267897220596353,
-18.9999975513786));
#18194=CARTESIAN_POINT('Ctrl Pts',(-0.5,0.285781297776546,-19.0001870446818));
#18195=CARTESIAN_POINT('Ctrl Pts',(-0.5,0.647589705255165,-19.007829931103));
#18196=CARTESIAN_POINT('Ctrl Pts',(-0.500000000105581,0.988814386378878,
-19.0846439716327));
#18197=CARTESIAN_POINT('Ctrl Pts',(-0.500000000105581,1.62420230789884,
-19.3558232592152));
#18198=CARTESIAN_POINT('Ctrl Pts',(-0.500000000128244,1.9184553255922,-19.5513503907418));
#18199=CARTESIAN_POINT('Ctrl Pts',(-0.500000000128245,2.44455222346988,
-20.0714825223491));
#18200=CARTESIAN_POINT('Ctrl Pts',(-0.499999999835989,2.62277718310116,
-20.3702706616735));
#18201=CARTESIAN_POINT('Ctrl Pts',(-0.499999999835989,2.81085194241867,
-20.8142013992923));
#18202=CARTESIAN_POINT('Ctrl Pts',(-0.499999999999019,2.86545769478055,
-20.9898894108025));
#18203=CARTESIAN_POINT('Ctrl Pts',(-0.499999999999019,2.93869922770866,
-21.3474407116196));
#18204=CARTESIAN_POINT('Ctrl Pts',(-0.500000000000001,2.95754616741604,
-21.5294711463845));
#18205=CARTESIAN_POINT('Ctrl Pts',(-0.500000000000001,2.95745837384903,
-21.7115232284929));
#18206=CARTESIAN_POINT('',(-0.500115915134107,-2.95873777012636,-21.7115199198582));
#18207=CARTESIAN_POINT('Ctrl Pts',(-0.499951156893989,2.95746669263463,
-21.7115242851505));
#18208=CARTESIAN_POINT('Ctrl Pts',(-0.77304186182352,2.91095244475281,-21.7153647174257));
#18209=CARTESIAN_POINT('Ctrl Pts',(-1.47173376114598,2.69128391286519,-21.7244418351522));
#18210=CARTESIAN_POINT('Ctrl Pts',(-2.42127475768073,1.9426253115599,-21.7340800035291));
#18211=CARTESIAN_POINT('Ctrl Pts',(-3.02252425451967,0.691565714094212,
-21.7387856518469));
#18212=CARTESIAN_POINT('Ctrl Pts',(-3.03256791313562,-1.16243137143974,
-21.7388525256077));
#18213=CARTESIAN_POINT('Ctrl Pts',(-1.91000215743889,-2.56265663733954,
-21.7300957759497));
#18214=CARTESIAN_POINT('Ctrl Pts',(-0.775090713331855,-2.91314336467866,
-21.7153814269834));
#18215=CARTESIAN_POINT('Ctrl Pts',(-0.500115915134107,-2.95873777012636,
-21.7115199198582));
#18216=CARTESIAN_POINT('',(-0.500000234886961,-0.250003167767838,-18.9999987296619));
#18217=CARTESIAN_POINT('Ctrl Pts',(-0.499999999999999,-2.95875698808065,
-21.7115182923403));
#18218=CARTESIAN_POINT('Ctrl Pts',(-0.499999999999999,-2.95871464996716,
-21.5295301198306));
#18219=CARTESIAN_POINT('Ctrl Pts',(-0.499999999998966,-2.93976151442474,
-21.3475736692592));
#18220=CARTESIAN_POINT('Ctrl Pts',(-0.499999999998966,-2.86636109777345,
-20.9901733930264));
#18221=CARTESIAN_POINT('Ctrl Pts',(-0.499999999825091,-2.81169983008533,
-20.8145582299835));
#18222=CARTESIAN_POINT('Ctrl Pts',(-0.499999999825091,-2.62343698647115,
-20.3705392694364));
#18223=CARTESIAN_POINT('Ctrl Pts',(-0.500000000056254,-2.44498872388035,
-20.0715359155249));
#18224=CARTESIAN_POINT('Ctrl Pts',(-0.500000000056255,-1.91832221676201,
-19.5511146046992));
#18225=CARTESIAN_POINT('Ctrl Pts',(-0.500000000109656,-1.62379237768017,
-19.3555089426616));
#18226=CARTESIAN_POINT('Ctrl Pts',(-0.500000000109656,-0.988284848212895,
-19.0845211957907));
#18227=CARTESIAN_POINT('Ctrl Pts',(-0.5,-0.647287344063983,-19.0078130433352));
#18228=CARTESIAN_POINT('Ctrl Pts',(-0.5,-0.285729446825272,-19.000186495383));
#18229=CARTESIAN_POINT('Ctrl Pts',(-0.500000469773922,-0.267871294986009,
-18.9999975511487));
#18230=CARTESIAN_POINT('Ctrl Pts',(-0.500000469773922,-0.250006335535676,
-18.9999974593238));
#18231=CARTESIAN_POINT('',(-0.5,-5.55111512312578E-17,-19.));
#18232=CARTESIAN_POINT('Origin',(-0.5,0.,0.));
#18233=CARTESIAN_POINT('',(-0.499999999999999,-2.95803989154981,-24.3207730140306));
#18234=CARTESIAN_POINT('',(-0.499999999999999,-2.95803989154981,-39.));
#18235=CARTESIAN_POINT('',(-0.500000000000001,2.95803989154981,-24.3207730140306));
#18236=CARTESIAN_POINT('Origin',(-0.5,0.,0.));
#18237=CARTESIAN_POINT('',(-0.500000000000001,2.95803989154981,-39.));
#18238=CARTESIAN_POINT('Origin',(0.,0.,-39.));
#18239=CARTESIAN_POINT('',(0.499940272430435,-2.95804998673149,-21.711522214267));
#18240=CARTESIAN_POINT('',(2.99999997687933,-0.000372456737699808,-21.7386095076915));
#18241=CARTESIAN_POINT('Ctrl Pts',(0.499940272430435,-2.95804998673149,
-21.711522214267));
#18242=CARTESIAN_POINT('Ctrl Pts',(0.590943823703178,-2.94266946901898,
-21.7128013793572));
#18243=CARTESIAN_POINT('Ctrl Pts',(0.681385576598305,-2.92306001474672,
-21.7140408866948));
#18244=CARTESIAN_POINT('Ctrl Pts',(0.770831732736946,-2.89927895170605,
-21.7152369587624));
#18245=CARTESIAN_POINT('Ctrl Pts',(0.860461624499595,-2.87544903884728,
-21.7164354877387));
#18246=CARTESIAN_POINT('Ctrl Pts',(0.949091358165715,-2.8474304009286,-21.7175904028168));
#18247=CARTESIAN_POINT('Ctrl Pts',(1.03629244274752,-2.81533265762758,-21.7186979031526));
#18248=CARTESIAN_POINT('Ctrl Pts',(1.12349352732932,-2.78323491432656,-21.7198054034884));
#18249=CARTESIAN_POINT('Ctrl Pts',(1.20926550868456,-2.74705819021273,-21.7208654890818));
#18250=CARTESIAN_POINT('Ctrl Pts',(1.29319479444907,-2.70696273036956,-21.7218743590889));
#18251=CARTESIAN_POINT('Ctrl Pts',(1.38514345926628,-2.66303618000959,-21.7229796258535));
#18252=CARTESIAN_POINT('Ctrl Pts',(1.47489868199608,-2.61439858546958,-21.7240234222307));
#18253=CARTESIAN_POINT('Ctrl Pts',(1.56199112027725,-2.56128556396491,-21.7250074208905));
#18254=CARTESIAN_POINT('Ctrl Pts',(1.64895180070953,-2.50825289452753,-21.7259899309072));
#18255=CARTESIAN_POINT('Ctrl Pts',(1.73325744965887,-2.45075848007837,-21.7269128239996));
#18256=CARTESIAN_POINT('Ctrl Pts',(1.81446485280803,-2.38908294077965,-21.7277777652573));
#18257=CARTESIAN_POINT('Ctrl Pts',(1.89558419876958,-2.3274742793064,-21.7286417686166));
#18258=CARTESIAN_POINT('Ctrl Pts',(1.97361172962793,-2.26169373032095,-21.7294479457531));
#18259=CARTESIAN_POINT('Ctrl Pts',(2.04813400568942,-2.19206457357866,-21.7301979563459));
#18260=CARTESIAN_POINT('Ctrl Pts',(2.12254107022213,-2.12254306359679,-21.7309468074213));
#18261=CARTESIAN_POINT('Ctrl Pts',(2.19345344471056,-2.04918503990753,-21.7316396654859));
#18262=CARTESIAN_POINT('Ctrl Pts',(2.26049198244141,-1.9723529089182,-21.7322781825327));
#18263=CARTESIAN_POINT('Ctrl Pts',(2.28763948139665,-1.94123945885854,-21.7325367523263));
#18264=CARTESIAN_POINT('Ctrl Pts',(2.31415211222994,-1.90955674624072,-21.7327864108756));
#18265=CARTESIAN_POINT('Ctrl Pts',(2.34000635954708,-1.87733061480369,-21.7330272678849));
#18266=CARTESIAN_POINT('Ctrl Pts',(2.39854660163678,-1.80436289260329,-21.7335726261566));
#18267=CARTESIAN_POINT('Ctrl Pts',(2.45373712959435,-1.72857119950941,-21.7340728608125));
#18268=CARTESIAN_POINT('Ctrl Pts',(2.50529507107785,-1.65030197443773,-21.7345302491155));
#18269=CARTESIAN_POINT('Ctrl Pts',(2.55682398716703,-1.57207681231841,-21.7349873799241));
#18270=CARTESIAN_POINT('Ctrl Pts',(2.60472412694322,-1.49137726307369,-21.7354017126085));
#18271=CARTESIAN_POINT('Ctrl Pts',(2.64875443563976,-1.40858082468799,-21.7357755205876));
#18272=CARTESIAN_POINT('Ctrl Pts',(2.69276900633143,-1.32581398070645,-21.7361491949543));
#18273=CARTESIAN_POINT('Ctrl Pts',(2.73291628446364,-1.24095213736414,-21.7364823735806));
#18274=CARTESIAN_POINT('Ctrl Pts',(2.76900059729431,-1.1543984113744,-21.7367773274486));
#18275=CARTESIAN_POINT('Ctrl Pts',(2.805096072164,-1.06781791153224,-21.7370723725553));
#18276=CARTESIAN_POINT('Ctrl Pts',(2.83712589208258,-0.979544899685551,
-21.7373291692517));
#18277=CARTESIAN_POINT('Ctrl Pts',(2.86494239747023,-0.890002842230036,
-21.737549990628));
#18278=CARTESIAN_POINT('Ctrl Pts',(2.88763517731577,-0.816954191134653,
-21.7377301373003));
#18279=CARTESIAN_POINT('Ctrl Pts',(2.90752472746022,-0.74306142296919,-21.737886341173));
#18280=CARTESIAN_POINT('Ctrl Pts',(2.92455565394967,-0.668561311287938,
-21.738019836408));
#18281=CARTESIAN_POINT('Ctrl Pts',(2.94760303630648,-0.567742805576745,
-21.738200491038));
#18282=CARTESIAN_POINT('Ctrl Pts',(2.96542043503695,-0.465786149542869,
-21.7383395586531));
#18283=CARTESIAN_POINT('Ctrl Pts',(2.97792997673742,-0.363225898923373,
-21.7384371460061));
#18284=CARTESIAN_POINT('Ctrl Pts',(2.99045332846363,-0.260552425954423,
-21.7385348410916));
#18285=CARTESIAN_POINT('Ctrl Pts',(2.99765708173621,-0.157274332776194,
-21.7385909642795));
#18286=CARTESIAN_POINT('Ctrl Pts',(2.99951519319889,-0.0539314914409496,
-21.7386056226765));
#18287=CARTESIAN_POINT('Ctrl Pts',(2.9998361735633,-0.0360794822708074,
-21.7386081548484));
#18288=CARTESIAN_POINT('Ctrl Pts',(2.99999776037856,-0.0182255429702799,
-21.7386094496693));
#18289=CARTESIAN_POINT('Ctrl Pts',(2.99999997687933,-0.000372456737699808,
-21.7386095076915));
#18290=CARTESIAN_POINT('',(0.500000000000001,-2.95803989154981,-24.3207730140306));
#18291=CARTESIAN_POINT('',(0.500000000000001,-2.95803989154981,-39.));
#18292=CARTESIAN_POINT('Ctrl Pts',(0.5,-2.95803989154981,-24.3207730140306));
#18293=CARTESIAN_POINT('Ctrl Pts',(0.331796881873696,-2.98647140773842,
-24.3173150006272));
#18294=CARTESIAN_POINT('Ctrl Pts',(0.163503365753253,-3.,-24.3156328315757));
#18295=CARTESIAN_POINT('Ctrl Pts',(6.93889390390723E-16,-3.,-24.3156328315757));
#18296=CARTESIAN_POINT('Ctrl Pts',(-0.163503365753251,-3.,-24.3156328315757));
#18297=CARTESIAN_POINT('Ctrl Pts',(-0.331796881873694,-2.98647140773842,
-24.3173150006272));
#18298=CARTESIAN_POINT('Ctrl Pts',(-0.499999999999998,-2.95803989154981,
-24.3207730140306));
#18299=CARTESIAN_POINT('',(0.499999999999999,2.95803989154981,-24.3207730140306));
#18300=CARTESIAN_POINT('Ctrl Pts',(-0.500000000000001,2.95803989154981,
-24.3207730140306));
#18301=CARTESIAN_POINT('Ctrl Pts',(-0.331796881873696,2.98647140773842,
-24.3173150006272));
#18302=CARTESIAN_POINT('Ctrl Pts',(-0.163503365753253,3.,-24.3156328315757));
#18303=CARTESIAN_POINT('Ctrl Pts',(0.163503365753251,3.,-24.3156328315757));
#18304=CARTESIAN_POINT('Ctrl Pts',(0.331796881873695,2.98647140773842,-24.3173150006272));
#18305=CARTESIAN_POINT('Ctrl Pts',(0.499999999999999,2.95803989154981,-24.3207730140306));
#18306=CARTESIAN_POINT('',(0.50001018530813,2.95803816990047,-21.711526659174));
#18307=CARTESIAN_POINT('',(0.499999999999999,2.95803989154981,-39.));
#18308=CARTESIAN_POINT('Ctrl Pts',(2.99999997687942,-0.00037245602236802,
-21.7386095076915));
#18309=CARTESIAN_POINT('Ctrl Pts',(3.0000127845348,0.102788624854442,-21.7386098429627));
#18310=CARTESIAN_POINT('Ctrl Pts',(2.99470015339322,0.205905039166103,-21.7385688825926));
#18311=CARTESIAN_POINT('Ctrl Pts',(2.984101926097,0.308440747412134,-21.7384867331043));
#18312=CARTESIAN_POINT('Ctrl Pts',(2.9734946788889,0.411063721483705,-21.7384045137005));
#18313=CARTESIAN_POINT('Ctrl Pts',(2.95759288398216,0.513104691368237,-21.7382810350385));
#18314=CARTESIAN_POINT('Ctrl Pts',(2.93648812652496,0.614033779834593,-21.7381164039139));
#18315=CARTESIAN_POINT('Ctrl Pts',(2.93249970587827,0.633107567396801,-21.7380852915841));
#18316=CARTESIAN_POINT('Ctrl Pts',(2.92832561220341,0.652141674306716,-21.738052709526));
#18317=CARTESIAN_POINT('Ctrl Pts',(2.92396666800349,0.671132568427846,-21.7380186584606));
#18318=CARTESIAN_POINT('Ctrl Pts',(2.90131380514578,0.769825761169153,-21.7378416995278));
#18319=CARTESIAN_POINT('Ctrl Pts',(2.87365847471177,0.867377264682175,-21.7376250664534));
#18320=CARTESIAN_POINT('Ctrl Pts',(2.84113991255455,0.963288117485888,-21.7373656504818));
#18321=CARTESIAN_POINT('Ctrl Pts',(2.80862455432068,1.05918952057843,-21.7371062600695));
#18322=CARTESIAN_POINT('Ctrl Pts',(2.77124703002945,1.1534502658333,-21.73680409519));
#18323=CARTESIAN_POINT('Ctrl Pts',(2.72919602839704,1.24558782852989,-21.7364560480066));
#18324=CARTESIAN_POINT('Ctrl Pts',(2.68715453496819,1.33770455788917,-21.7361080795205));
#18325=CARTESIAN_POINT('Ctrl Pts',(2.64044181798012,1.42769874705926,-21.735714249477));
#18326=CARTESIAN_POINT('Ctrl Pts',(2.58929405009832,1.51510934329026,-21.7352714521471));
#18327=CARTESIAN_POINT('Ctrl Pts',(2.53815579233109,1.60250368691006,-21.7348287371483));
#18328=CARTESIAN_POINT('Ctrl Pts',(2.48258430377546,1.68731509589525,-21.7343370730706));
#18329=CARTESIAN_POINT('Ctrl Pts',(2.42286088774972,1.7691085660899,-21.733793355917));
#18330=CARTESIAN_POINT('Ctrl Pts',(2.3964348284965,1.80530005066537,-21.7335527752088));
#18331=CARTESIAN_POINT('Ctrl Pts',(2.36919646981116,1.84090103915332,-21.7333020033804));
#18332=CARTESIAN_POINT('Ctrl Pts',(2.34117286728839,1.87587569030377,-21.7330407715356));
#18333=CARTESIAN_POINT('Ctrl Pts',(2.28254921400658,1.94904050988863,-21.7324942905796));
#18334=CARTESIAN_POINT('Ctrl Pts',(2.22046791995484,2.01948508884061,-21.7319020344294));
#18335=CARTESIAN_POINT('Ctrl Pts',(2.15522082010883,2.08686923801407,-21.7312628877286));
#18336=CARTESIAN_POINT('Ctrl Pts',(2.08995164894374,2.15427618141227,-21.7306235248219));
#18337=CARTESIAN_POINT('Ctrl Pts',(2.02151484114231,2.21862029555148,-21.7299372396356));
#18338=CARTESIAN_POINT('Ctrl Pts',(1.95024012850979,2.2795972102874,-21.7292029156811));
#18339=CARTESIAN_POINT('Ctrl Pts',(1.87895512064779,2.3405829327941,-21.7284684856577));
#18340=CARTESIAN_POINT('Ctrl Pts',(1.80483174370816,2.39820020280533,-21.7276860029873));
#18341=CARTESIAN_POINT('Ctrl Pts',(1.72823246505674,2.45218525946225,-21.7268543506973));
#18342=CARTESIAN_POINT('Ctrl Pts',(1.65154865351808,2.50622989256409,-21.7260217806185));
#18343=CARTESIAN_POINT('Ctrl Pts',(1.57238386054189,2.55663405610847,-21.7251399323357));
#18344=CARTESIAN_POINT('Ctrl Pts',(1.4911288350491,2.60317782667361,-21.7242076851744));
#18345=CARTESIAN_POINT('Ctrl Pts',(1.42637349841828,2.64027039433615,-21.7234647406195));
#18346=CARTESIAN_POINT('Ctrl Pts',(1.36029123456075,2.67491201703164,-21.7226897871063));
#18347=CARTESIAN_POINT('Ctrl Pts',(1.29308953927524,2.70701301131283,-21.7218822574094));
#18348=CARTESIAN_POINT('Ctrl Pts',(1.20152615241017,2.75075113050215,-21.7207819852553));
#18349=CARTESIAN_POINT('Ctrl Pts',(1.10784733971323,2.78978932872495,-21.7196212370477));
#18350=CARTESIAN_POINT('Ctrl Pts',(1.01254488240596,2.82396049213042,-21.7184045040822));
#18351=CARTESIAN_POINT('Ctrl Pts',(0.91697196252464,2.8582286312181,-21.7171843181026));
#18352=CARTESIAN_POINT('Ctrl Pts',(0.819766510469706,2.88760200735712,-21.7159078291516));
#18353=CARTESIAN_POINT('Ctrl Pts',(0.721435405590029,2.91196341933774,-21.7145795668714));
#18354=CARTESIAN_POINT('Ctrl Pts',(0.648180881864355,2.93011213874966,-21.7135900405069));
#18355=CARTESIAN_POINT('Ctrl Pts',(0.574301882693173,2.94548031795849,-21.7125717803367));
#18356=CARTESIAN_POINT('Ctrl Pts',(0.50001018530813,2.95803816990047,-21.711526659174));
#18357=CARTESIAN_POINT('',(3.,-3.67394039744206E-16,-31.));
#18358=CARTESIAN_POINT('',(3.,3.67394039744206E-16,-39.));
#18359=CARTESIAN_POINT('Origin',(0.,0.,-31.));
#18360=CARTESIAN_POINT('Ctrl Pts',(0.500000469469733,0.249901395253279,
-18.9999974609542));
#18361=CARTESIAN_POINT('Ctrl Pts',(0.499985448741165,0.249900114038217,
-18.9999972448598));
#18362=CARTESIAN_POINT('Ctrl Pts',(0.499957241892024,0.233340007311912,
-18.9999932538032));
#18363=CARTESIAN_POINT('Ctrl Pts',(0.499923116192456,0.161617649106977,
-18.999991205498));
#18364=CARTESIAN_POINT('Ctrl Pts',(0.499903664329549,0.0578515636974027,
-18.9999911080249));
#18365=CARTESIAN_POINT('Ctrl Pts',(0.499903654156312,-0.0575152632728968,
-18.9999911064299));
#18366=CARTESIAN_POINT('Ctrl Pts',(0.499923182383946,-0.161934911996989,
-18.9999912099571));
#18367=CARTESIAN_POINT('Ctrl Pts',(0.499957222601439,-0.2331464309115,-18.9999932557911));
#18368=CARTESIAN_POINT('Ctrl Pts',(0.499985489070265,-0.249900109125001,
-18.9999972525014));
#18369=CARTESIAN_POINT('Ctrl Pts',(0.500000469469733,-0.249901395253278,
-18.9999974609542));
#18370=CARTESIAN_POINT('Ctrl Pts',(0.500005900016648,1.07273098925591,-18.9999680907812));
#18371=CARTESIAN_POINT('Ctrl Pts',(0.617767041361557,1.05838429499492,-19.022282173232));
#18372=CARTESIAN_POINT('Ctrl Pts',(0.846046576080114,0.968758311001584,
-19.0545829182515));
#18373=CARTESIAN_POINT('Ctrl Pts',(1.12222781977421,0.664689166031461,-19.0711604080831));
#18374=CARTESIAN_POINT('Ctrl Pts',(1.27965290692711,0.238169452169252,-19.0719492566763));
#18375=CARTESIAN_POINT('Ctrl Pts',(1.27973523736976,-0.237098271262147,
-19.0719621646337));
#18376=CARTESIAN_POINT('Ctrl Pts',(1.12169212850501,-0.666446847723124,
-19.0711243191322));
#18377=CARTESIAN_POINT('Ctrl Pts',(0.846202696406831,-0.968026558196811,
-19.0545668296603));
#18378=CARTESIAN_POINT('Ctrl Pts',(0.617440655867346,-1.05842405813617,
-19.0222203277647));
#18379=CARTESIAN_POINT('Ctrl Pts',(0.500005900016646,-1.07273098925591,
-18.9999680907812));
#18380=CARTESIAN_POINT('Ctrl Pts',(0.374652474916355,2.49810289705817,-19.6779203934124));
#18381=CARTESIAN_POINT('Ctrl Pts',(0.709305752982863,2.46080584278846,-19.7142751509983));
#18382=CARTESIAN_POINT('Ctrl Pts',(1.35615168283393,2.24374271780176,-19.7670860721376));
#18383=CARTESIAN_POINT('Ctrl Pts',(2.1329201530783,1.53847021337198,-19.7950950890783));
#18384=CARTESIAN_POINT('Ctrl Pts',(2.57376683871501,0.551282961402653,-19.7975916138405));
#18385=CARTESIAN_POINT('Ctrl Pts',(2.57408967206061,-0.547867981449944,
-19.7976642591583));
#18386=CARTESIAN_POINT('Ctrl Pts',(2.13140251423125,-1.54147604638236,-19.7950284546789));
#18387=CARTESIAN_POINT('Ctrl Pts',(1.35656907690939,-2.24213495858108,-19.7670579619609));
#18388=CARTESIAN_POINT('Ctrl Pts',(0.708378231609485,-2.46090921489704,
-19.714174390549));
#18389=CARTESIAN_POINT('Ctrl Pts',(0.374652474916349,-2.49810289705816,
-19.6779203934123));
#18390=CARTESIAN_POINT('Ctrl Pts',(0.112199737628205,3.,-21.0973505959298));
#18391=CARTESIAN_POINT('Ctrl Pts',(0.545411427143746,2.98330034061039,-21.1128737181934));
#18392=CARTESIAN_POINT('Ctrl Pts',(1.40427349900891,2.76191133949964,-21.1369675122343));
#18393=CARTESIAN_POINT('Ctrl Pts',(2.44430058904568,1.90558580922904,-21.1529929864137));
#18394=CARTESIAN_POINT('Ctrl Pts',(3.02549037952742,0.682395833387457,-21.157041989878));
#18395=CARTESIAN_POINT('Ctrl Pts',(3.0259004610393,-0.678602295043218,-21.1570750782405));
#18396=CARTESIAN_POINT('Ctrl Pts',(2.44234453420329,-1.90963524646961,-21.1529563713896));
#18397=CARTESIAN_POINT('Ctrl Pts',(1.40492007795907,-2.75971795905596,-21.1369594501161));
#18398=CARTESIAN_POINT('Ctrl Pts',(0.544210742352774,-2.9833466252041,-21.1128306944771));
#18399=CARTESIAN_POINT('Ctrl Pts',(0.112199737628197,-3.,-21.0973505959298));
#18400=CARTESIAN_POINT('Ctrl Pts',(-1.54352792291549E-15,3.,-21.704163456598));
#18401=CARTESIAN_POINT('Ctrl Pts',(0.443076803624565,3.,-21.7109905340956));
#18402=CARTESIAN_POINT('Ctrl Pts',(1.33511706912935,2.80117039424009,-21.7230605835255));
#18403=CARTESIAN_POINT('Ctrl Pts',(2.4220516933108,1.94015762628841,-21.734095700974));
#18404=CARTESIAN_POINT('Ctrl Pts',(3.0250024087078,0.694486097636399,-21.7388012417923));
#18405=CARTESIAN_POINT('Ctrl Pts',(3.02547331281169,-0.690449402995863,
-21.7388112826209));
#18406=CARTESIAN_POINT('Ctrl Pts',(2.42004703065636,-1.94396691644154,-21.7340726461722));
#18407=CARTESIAN_POINT('Ctrl Pts',(1.33584761178912,-2.79884667955486,-21.7230617399995));
#18408=CARTESIAN_POINT('Ctrl Pts',(0.441848776790988,-3.,-21.7109716122421));
#18409=CARTESIAN_POINT('Ctrl Pts',(-1.02690891338221E-14,-3.,-21.704163456598));
#18410=CARTESIAN_POINT('',(0.500000234886957,-0.250003172328592,-18.999998729662));
#18411=CARTESIAN_POINT('Ctrl Pts',(0.500000469773915,-0.250006344657184,
-18.9999974593239));
#18412=CARTESIAN_POINT('Ctrl Pts',(0.500000469773915,-0.267897220477188,
-18.9999975513786));
#18413=CARTESIAN_POINT('Ctrl Pts',(0.5,-0.285781297573261,-19.0001870446798));
#18414=CARTESIAN_POINT('Ctrl Pts',(0.5,-0.647592139377092,-19.0078299813172));
#18415=CARTESIAN_POINT('Ctrl Pts',(0.500000000107083,-0.988819809921417,
-19.0846450518276));
#18416=CARTESIAN_POINT('Ctrl Pts',(0.500000000107083,-1.62420594756027,
-19.3558259127742));
#18417=CARTESIAN_POINT('Ctrl Pts',(0.500000000134817,-1.91845500253887,
-19.5513515847871));
#18418=CARTESIAN_POINT('Ctrl Pts',(0.500000000134817,-2.44454481720606,
-20.0714810657466));
#18419=CARTESIAN_POINT('Ctrl Pts',(0.499999999833624,-2.62276820685551,
-20.3702686628235));
#18420=CARTESIAN_POINT('Ctrl Pts',(0.499999999833624,-2.8108434657848,-20.8141963403292));
#18421=CARTESIAN_POINT('Ctrl Pts',(0.499999999999008,-2.86545068011728,
-20.9898853131812));
#18422=CARTESIAN_POINT('Ctrl Pts',(0.499999999999008,-2.93869493016462,
-21.34743767588));
#18423=CARTESIAN_POINT('Ctrl Pts',(0.500000000000001,-2.95754307939312,
-21.52946525912));
#18424=CARTESIAN_POINT('Ctrl Pts',(0.500000000000001,-2.95745543349273,
-21.7115181370337));
#18425=CARTESIAN_POINT('',(0.500000234886961,0.250003167767864,-18.9999987296619));
#18426=CARTESIAN_POINT('Ctrl Pts',(0.499999999999999,2.957907651092,-21.7115138352691));
#18427=CARTESIAN_POINT('Ctrl Pts',(0.499999999999999,2.95794618991124,-21.5294887787061));
#18428=CARTESIAN_POINT('Ctrl Pts',(0.499999999999071,2.93905776709014,-21.3474868610508));
#18429=CARTESIAN_POINT('Ctrl Pts',(0.499999999999071,2.86575493753945,-20.9899915011559));
#18430=CARTESIAN_POINT('Ctrl Pts',(0.499999999845862,2.81112639164981,-20.814326068996));
#18431=CARTESIAN_POINT('Ctrl Pts',(0.499999999845862,2.62297984800933,-20.3703581369862));
#18432=CARTESIAN_POINT('Ctrl Pts',(0.500000000064459,2.44467766128549,-20.071497650565));
#18433=CARTESIAN_POINT('Ctrl Pts',(0.500000000064459,1.91840198171423,-19.5512716141705));
#18434=CARTESIAN_POINT('Ctrl Pts',(0.500000000096094,1.6240590615628,-19.3557175409153));
#18435=CARTESIAN_POINT('Ctrl Pts',(0.500000000096094,0.988617937234748,
-19.0845954286414));
#18436=CARTESIAN_POINT('Ctrl Pts',(0.5,0.647452490142017,-19.007816540113));
#18437=CARTESIAN_POINT('Ctrl Pts',(0.5,0.285729437884547,-19.0001864952732));
#18438=CARTESIAN_POINT('Ctrl Pts',(0.500000469773922,0.267871290073013,
-18.9999975511486));
#18439=CARTESIAN_POINT('Ctrl Pts',(0.500000469773922,0.250006335535729,
-18.9999974593238));
#18440=CARTESIAN_POINT('',(0.5,1.66533453693773E-16,-19.));
#18441=CARTESIAN_POINT('Origin',(0.5,2.22044604925031E-16,0.));
#18442=CARTESIAN_POINT('Origin',(0.5,2.22044604925031E-16,0.));
#18443=CARTESIAN_POINT('Origin',(-0.5,0.,0.));
#18444=CARTESIAN_POINT('Ctrl Pts',(1.43046189829788,-2.88176118076299,-39.4132320681314));
#18445=CARTESIAN_POINT('Ctrl Pts',(2.37482146118144,-2.41299562794209,-39.3480377810873));
#18446=CARTESIAN_POINT('Ctrl Pts',(3.75195145870749,-0.483252427376924,
-39.2176492069991));
#18447=CARTESIAN_POINT('Ctrl Pts',(2.48093138115386,2.86039701702348,-39.0220663458667));
#18448=CARTESIAN_POINT('Ctrl Pts',(-1.00431634631447,3.64773132007517,-38.8264834847344));
#18449=CARTESIAN_POINT('Ctrl Pts',(-3.59288022276291,1.18807557140504,-38.6309006236019));
#18450=CARTESIAN_POINT('Ctrl Pts',(-2.98062062312938,-2.33209228359478,
-38.4353177624696));
#18451=CARTESIAN_POINT('Ctrl Pts',(0.288167629773712,-3.77318109983691,
-38.2397349013372));
#18452=CARTESIAN_POINT('Ctrl Pts',(3.29994356574598,-1.85236689627126,-38.0441520402049));
#18453=CARTESIAN_POINT('Ctrl Pts',(3.37118335473764,1.71935931877143,-37.8485691790725));
#18454=CARTESIAN_POINT('Ctrl Pts',(0.438236617843253,3.75881325515087,-37.6529863179401));
#18455=CARTESIAN_POINT('Ctrl Pts',(-2.88520346695894,2.44877028859547,-37.4574034568077));
#18456=CARTESIAN_POINT('Ctrl Pts',(-3.63759395527955,-1.04345151662343,
-37.2618205956754));
#18457=CARTESIAN_POINT('Ctrl Pts',(-1.14844282939652,-3.60581742991611,
-37.066237734543));
#18458=CARTESIAN_POINT('Ctrl Pts',(2.36410557671837,-2.95497314639522,-36.8706548734106));
#18459=CARTESIAN_POINT('Ctrl Pts',(3.76995295045892,0.329111973093684,-36.6750720122782));
#18460=CARTESIAN_POINT('Ctrl Pts',(1.8163171711215,3.3199167664903,-36.4794891511459));
#18461=CARTESIAN_POINT('Ctrl Pts',(-1.75587554620208,3.35227674819956,-36.2839062900135));
#18462=CARTESIAN_POINT('Ctrl Pts',(-3.76337186360745,0.397353826106389,
-36.0883234288811));
#18463=CARTESIAN_POINT('Ctrl Pts',(-2.41725037419006,-2.91165897783182,
-35.8927405677487));
#18464=CARTESIAN_POINT('Ctrl Pts',(1.08293233547133,-3.6260329995702,-35.6971577066164));
#18465=CARTESIAN_POINT('Ctrl Pts',(3.61809190721629,-1.10917474504408,-35.501574845484));
#18466=CARTESIAN_POINT('Ctrl Pts',(2.92909571917959,2.39609179780073,-35.3059919843517));
#18467=CARTESIAN_POINT('Ctrl Pts',(-0.370077606085909,3.76615190892214,
-35.1104091232193));
#18468=CARTESIAN_POINT('Ctrl Pts',(-3.33946720062995,1.78011698492664,-34.9148262620869));
#18469=CARTESIAN_POINT('Ctrl Pts',(-3.33298923708603,-1.79221664500977,
-34.7192434009545));
#18470=CARTESIAN_POINT('Ctrl Pts',(-0.356416329777662,-3.76746927984535,
-34.5236605398222));
#18471=CARTESIAN_POINT('Ctrl Pts',(2.93776641840763,-2.38545306342213,-34.3280776786898));
#18472=CARTESIAN_POINT('Ctrl Pts',(3.61404547698157,1.12228945489961,-34.1324948175575));
#18473=CARTESIAN_POINT('Ctrl Pts',(1.06977446774459,3.629936361797,-33.9369119564251));
#18474=CARTESIAN_POINT('Ctrl Pts',(-2.42779410945176,2.90287369715232,-33.7413290952927));
#18475=CARTESIAN_POINT('Ctrl Pts',(-3.76190637086622,-0.411001132144213,
-33.5457462341603));
#18476=CARTESIAN_POINT('Ctrl Pts',(-1.74370548238732,-3.35862046992087,
-33.350163373028));
#18477=CARTESIAN_POINT('Ctrl Pts',(1.82834428848415,-3.3133122421223,-33.1545805118956));
#18478=CARTESIAN_POINT('Ctrl Pts',(3.77112451550319,-0.315428059358477,
-32.9589976507632));
#18479=CARTESIAN_POINT('Ctrl Pts',(2.35336766298509,2.96350958546327,-32.7634147896309));
#18480=CARTESIAN_POINT('Ctrl Pts',(-1.16150178032287,3.60166451694395,-32.5678319284985));
#18481=CARTESIAN_POINT('Ctrl Pts',(-3.64137583224079,1.03018090832754,-32.3722490673661));
#18482=CARTESIAN_POINT('Ctrl Pts',(-2.8762608737732,-2.45907697744851,-32.1766662062337));
#18483=CARTESIAN_POINT('Ctrl Pts',(0.451781530523055,-3.75747883119848,
-31.9810833451013));
#18484=CARTESIAN_POINT('Ctrl Pts',(3.37756428501257,-1.70656712704126,-31.785500483969));
#18485=CARTESIAN_POINT('Ctrl Pts',(3.29287076467101,1.86322227179335,-31.5899176228366));
#18486=CARTESIAN_POINT('Ctrl Pts',(0.275155398406671,3.77639790272669,-31.3943347617042));
#18487=CARTESIAN_POINT('Ctrl Pts',(-2.99125666928477,2.31641984474353,-31.1987098698809));
#18488=CARTESIAN_POINT('Ctrl Pts',(-3.3857956881288,-0.0223753480619818,
-31.0682792651016));
#18489=CARTESIAN_POINT('Ctrl Pts',(-3.05040623055311,-1.02263886777266,
-31.0030429473666));
#18490=CARTESIAN_POINT('Ctrl Pts',(1.53694905724646,-3.0962866856177,-39.2749561275222));
#18491=CARTESIAN_POINT('Ctrl Pts',(2.55160910628562,-2.59262505343092,-39.2097618404781));
#18492=CARTESIAN_POINT('Ctrl Pts',(4.03125610277118,-0.519226945892664,
-39.0793732663898));
#18493=CARTESIAN_POINT('Ctrl Pts',(2.66561811390768,3.07333212013268,-38.8837904052575));
#18494=CARTESIAN_POINT('Ctrl Pts',(-1.07908016528225,3.91927755653543,-38.6882075441251));
#18495=CARTESIAN_POINT('Ctrl Pts',(-3.86034320644659,1.27651888636902,-38.4926246829927));
#18496=CARTESIAN_POINT('Ctrl Pts',(-3.20250547195918,-2.5056990619238,-38.2970418218604));
#18497=CARTESIAN_POINT('Ctrl Pts',(0.309619548368721,-4.05406613144679,
-38.1014589607279));
#18498=CARTESIAN_POINT('Ctrl Pts',(3.54559961252715,-1.99026171776147,-37.9058760995957));
#18499=CARTESIAN_POINT('Ctrl Pts',(3.62214266946524,1.84735272375873,-37.7102932384632));
#18500=CARTESIAN_POINT('Ctrl Pts',(0.47086004698659,4.03862870849191,-37.5147103773309));
#18501=CARTESIAN_POINT('Ctrl Pts',(-3.09998522420157,2.6310628692371,-37.3191275161985));
#18502=CARTESIAN_POINT('Ctrl Pts',(-3.9083855409675,-1.12112865548188,-37.1235446550661));
#18503=CARTESIAN_POINT('Ctrl Pts',(-1.2339357839889,-3.87424349163502,-36.9279617939337));
#18504=CARTESIAN_POINT('Ctrl Pts',(2.54009550460026,-3.17494873295464,-36.7323789328014));
#18505=CARTESIAN_POINT('Ctrl Pts',(4.05059767056079,0.353611890940086,-36.536796071669));
#18506=CARTESIAN_POINT('Ctrl Pts',(1.95152836097032,3.5670596682551,-36.3412132105366));
#18507=CARTESIAN_POINT('Ctrl Pts',(-1.88658731042651,3.60182860788203,-36.1456303494043));
#18508=CARTESIAN_POINT('Ctrl Pts',(-4.0435266711556,0.42693383805202,-35.9500474882719));
#18509=CARTESIAN_POINT('Ctrl Pts',(-2.59719653362373,-3.12841014942569,
-35.7544646271396));
#18510=CARTESIAN_POINT('Ctrl Pts',(1.1635485251616,-3.89596395882014,-35.5588817660071));
#18511=CARTESIAN_POINT('Ctrl Pts',(3.88743171170376,-1.19174448529219,-35.3632989048749));
#18512=CARTESIAN_POINT('Ctrl Pts',(3.14714492538008,2.57446285992508,-35.1677160437424));
#18513=CARTESIAN_POINT('Ctrl Pts',(-0.39762710804012,4.04651366999184,-34.9721331826101));
#18514=CARTESIAN_POINT('Ctrl Pts',(-3.58806548557568,1.91263334243781,-34.7765503214776));
#18515=CARTESIAN_POINT('Ctrl Pts',(-3.58110528623479,-1.92563373145894,
-34.5809674603453));
#18516=CARTESIAN_POINT('Ctrl Pts',(-0.382948852179039,-4.04792910929916,
-34.3853845992129));
#18517=CARTESIAN_POINT('Ctrl Pts',(3.15646109312986,-2.56303215156931,-34.1898017380806));
#18518=CARTESIAN_POINT('Ctrl Pts',(3.88308405508889,1.20583548692774,-33.9942188769482));
#18519=CARTESIAN_POINT('Ctrl Pts',(1.14941115287504,3.90015789708702,-33.7986360158158));
#18520=CARTESIAN_POINT('Ctrl Pts',(-2.6085251708909,3.11897087049483,-33.6030531546835));
#18521=CARTESIAN_POINT('Ctrl Pts',(-4.04195208347193,-0.44159708366083,
-33.4074702935511));
#18522=CARTESIAN_POINT('Ctrl Pts',(-1.873511276644,-3.60864457210354,-33.2118874324187));
#18523=CARTESIAN_POINT('Ctrl Pts',(1.96445080700954,-3.55996348658607,-33.0163045712863));
#18524=CARTESIAN_POINT('Ctrl Pts',(4.05185644983512,-0.338909312465405,
-32.820721710154));
#18525=CARTESIAN_POINT('Ctrl Pts',(2.52855823373077,3.18412064588255,-32.6251388490216));
#18526=CARTESIAN_POINT('Ctrl Pts',(-1.24796687586121,3.86978142544159,-32.4295559878892));
#18527=CARTESIAN_POINT('Ctrl Pts',(-3.912448950302,1.10687014993642,-32.2339731267569));
#18528=CARTESIAN_POINT('Ctrl Pts',(-3.09037692202834,-2.64213681376848,
-32.0383902656245));
#18529=CARTESIAN_POINT('Ctrl Pts',(0.485413276819888,-4.03719494668529,
-31.8428074044921));
#18530=CARTESIAN_POINT('Ctrl Pts',(3.62899861213807,-1.83360824930386,-31.6472245433597));
#18531=CARTESIAN_POINT('Ctrl Pts',(3.53800029446268,2.00192519456892,-31.4516416822274));
#18532=CARTESIAN_POINT('Ctrl Pts',(0.295638653976472,4.05752240118364,-31.256058821095));
#18533=CARTESIAN_POINT('Ctrl Pts',(-3.21393329197368,2.48885992755341,-31.0604339292716));
#18534=CARTESIAN_POINT('Ctrl Pts',(-3.63784278147551,-0.0240410248957648,
-30.9300033244924));
#18535=CARTESIAN_POINT('Ctrl Pts',(-3.27748609441888,-1.09876666103236,
-30.8647670067574));
#18536=CARTESIAN_POINT('Ctrl Pts',(1.64343621619505,-3.3108121904724,-39.136680186913));
#18537=CARTESIAN_POINT('Ctrl Pts',(2.7283967513898,-2.77225447891975,-39.0714858998688));
#18538=CARTESIAN_POINT('Ctrl Pts',(4.31056074683487,-0.555201464408408,
-38.9410973257805));
#18539=CARTESIAN_POINT('Ctrl Pts',(2.8503048466615,3.28626722324188,-38.7455144646482));
#18540=CARTESIAN_POINT('Ctrl Pts',(-1.15384398425004,4.19082379299567,-38.5499316035159));
#18541=CARTESIAN_POINT('Ctrl Pts',(-4.12780619013028,1.36496220133301,-38.3543487423834));
#18542=CARTESIAN_POINT('Ctrl Pts',(-3.42439032078898,-2.67930584025284,
-38.1587658812511));
#18543=CARTESIAN_POINT('Ctrl Pts',(0.331071466963731,-4.33495116305667,
-37.9631830201187));
#18544=CARTESIAN_POINT('Ctrl Pts',(3.79125565930832,-2.12815653925168,-37.7676001589864));
#18545=CARTESIAN_POINT('Ctrl Pts',(3.87310198419283,1.97534612874602,-37.572017297854));
#18546=CARTESIAN_POINT('Ctrl Pts',(0.503483476129927,4.31844416183293,-37.3764344367216));
#18547=CARTESIAN_POINT('Ctrl Pts',(-3.31476698144421,2.81335544987872,-37.1808515755893));
#18548=CARTESIAN_POINT('Ctrl Pts',(-4.17917712665544,-1.19880579434034,
-36.9852687144569));
#18549=CARTESIAN_POINT('Ctrl Pts',(-1.31942873858128,-4.14266955335393,
-36.7896858533245));
#18550=CARTESIAN_POINT('Ctrl Pts',(2.71608543248216,-3.39492431951407,-36.5941029921921));
#18551=CARTESIAN_POINT('Ctrl Pts',(4.33124239066266,0.378111808786486,-36.3985201310598));
#18552=CARTESIAN_POINT('Ctrl Pts',(2.08673955081914,3.8142025700199,-36.2029372699274));
#18553=CARTESIAN_POINT('Ctrl Pts',(-2.01729907465095,3.85138046756452,-36.007354408795));
#18554=CARTESIAN_POINT('Ctrl Pts',(-4.32368147870374,0.456513849997653,
-35.8117715476627));
#18555=CARTESIAN_POINT('Ctrl Pts',(-2.7771426930574,-3.34516132101955,-35.6161886865303));
#18556=CARTESIAN_POINT('Ctrl Pts',(1.24416471485188,-4.16589491807009,-35.4206058253979));
#18557=CARTESIAN_POINT('Ctrl Pts',(4.15677151619123,-1.2743142255403,-35.2250229642655));
#18558=CARTESIAN_POINT('Ctrl Pts',(3.36519413158057,2.75283392204944,-35.0294401031332));
#18559=CARTESIAN_POINT('Ctrl Pts',(-0.42517660999433,4.32687543106154,-34.8338572420008));
#18560=CARTESIAN_POINT('Ctrl Pts',(-3.83666377052141,2.04514969994899,-34.6382743808684));
#18561=CARTESIAN_POINT('Ctrl Pts',(-3.82922133538355,-2.05905081790811,
-34.442691519736));
#18562=CARTESIAN_POINT('Ctrl Pts',(-0.409481374580417,-4.32838893875298,
-34.2471086586037));
#18563=CARTESIAN_POINT('Ctrl Pts',(3.37515576785208,-2.7406112397165,-34.0515257974713));
#18564=CARTESIAN_POINT('Ctrl Pts',(4.1521226331962,1.28938151895587,-33.855942936339));
#18565=CARTESIAN_POINT('Ctrl Pts',(1.22904783800549,4.17037943237703,-33.6603600752066));
#18566=CARTESIAN_POINT('Ctrl Pts',(-2.78925623233004,3.33506804383733,-33.4647772140742));
#18567=CARTESIAN_POINT('Ctrl Pts',(-4.32199779607761,-0.472193035177443,
-33.2691943529418));
#18568=CARTESIAN_POINT('Ctrl Pts',(-2.0033170709007,-3.8586686742862,-33.0736114918095));
#18569=CARTESIAN_POINT('Ctrl Pts',(2.10055732553492,-3.80661473104982,-32.8780286306771));
#18570=CARTESIAN_POINT('Ctrl Pts',(4.33258838416705,-0.362390565572336,
-32.6824457695447));
#18571=CARTESIAN_POINT('Ctrl Pts',(2.70374880447645,3.40473170630184,-32.4868629084123));
#18572=CARTESIAN_POINT('Ctrl Pts',(-1.33443197139957,4.13789833393923,-32.29128004728));
#18573=CARTESIAN_POINT('Ctrl Pts',(-4.1835220683632,1.18355939154531,-32.0956971861476));
#18574=CARTESIAN_POINT('Ctrl Pts',(-3.30449297028347,-2.82519665008844,
-31.9001143250153));
#18575=CARTESIAN_POINT('Ctrl Pts',(0.519045023116724,-4.31691106217212,
-31.7045314638828));
#18576=CARTESIAN_POINT('Ctrl Pts',(3.88043293926357,-1.96064937156648,-31.5089486027505));
#18577=CARTESIAN_POINT('Ctrl Pts',(3.78312982425436,2.14062811734448,-31.3133657416181));
#18578=CARTESIAN_POINT('Ctrl Pts',(0.316121909546268,4.33864689964057,-31.1177828804858));
#18579=CARTESIAN_POINT('Ctrl Pts',(-3.43660991466259,2.66130001036329,-30.9221579886624));
#18580=CARTESIAN_POINT('Ctrl Pts',(-3.88988987482222,-0.0257067017295483,
-30.7917273838832));
#18581=CARTESIAN_POINT('Ctrl Pts',(-3.50456595828466,-1.17489445429207,
-30.7264910661481));
#18582=CARTESIAN_POINT('Ctrl Pts',(1.74992337514364,-3.52533769532709,-38.9984042463037));
#18583=CARTESIAN_POINT('Ctrl Pts',(2.90518439649398,-2.95188390440858,-38.9332099592596));
#18584=CARTESIAN_POINT('Ctrl Pts',(4.58986539089856,-0.591175982924146,
-38.8028213851713));
#18585=CARTESIAN_POINT('Ctrl Pts',(3.03499157941532,3.49920232635108,-38.607238524039));
#18586=CARTESIAN_POINT('Ctrl Pts',(-1.22860780321782,4.46237002945592,-38.4116556629066));
#18587=CARTESIAN_POINT('Ctrl Pts',(-4.39526917381396,1.45340551629699,-38.2160728017742));
#18588=CARTESIAN_POINT('Ctrl Pts',(-3.64627516961878,-2.85291261858187,
-38.0204899406419));
#18589=CARTESIAN_POINT('Ctrl Pts',(0.352523385558738,-4.61583619466654,
-37.8249070795095));
#18590=CARTESIAN_POINT('Ctrl Pts',(4.0369117060895,-2.26605136074189,-37.6293242183772));
#18591=CARTESIAN_POINT('Ctrl Pts',(4.12406129892043,2.10333953373333,-37.4337413572447));
#18592=CARTESIAN_POINT('Ctrl Pts',(0.536106905273268,4.59825961517397,-37.2381584961124));
#18593=CARTESIAN_POINT('Ctrl Pts',(-3.52954873868685,2.99564803052035,-37.04257563498));
#18594=CARTESIAN_POINT('Ctrl Pts',(-4.44996871234337,-1.2764829331988,-36.8469927738476));
#18595=CARTESIAN_POINT('Ctrl Pts',(-1.40492169317366,-4.41109561507284,
-36.6514099127152));
#18596=CARTESIAN_POINT('Ctrl Pts',(2.89207536036405,-3.6148999060735,-36.4558270515829));
#18597=CARTESIAN_POINT('Ctrl Pts',(4.61188711076453,0.402611726632887,-36.2602441904505));
#18598=CARTESIAN_POINT('Ctrl Pts',(2.22195074066797,4.06134547178471,-36.0646613293182));
#18599=CARTESIAN_POINT('Ctrl Pts',(-2.14801083887538,4.100932327247,-35.8690784681858));
#18600=CARTESIAN_POINT('Ctrl Pts',(-4.60383628625188,0.486093861943285,
-35.6734956070534));
#18601=CARTESIAN_POINT('Ctrl Pts',(-2.95708885249107,-3.56191249261342,
-35.4779127459211));
#18602=CARTESIAN_POINT('Ctrl Pts',(1.32478090454216,-4.43582587732003,-35.2823298847886));
#18603=CARTESIAN_POINT('Ctrl Pts',(4.42611132067871,-1.3568839657884,-35.0867470236564));
#18604=CARTESIAN_POINT('Ctrl Pts',(3.58324333778105,2.93120498417377,-34.8911641625239));
#18605=CARTESIAN_POINT('Ctrl Pts',(-0.45272611194854,4.60723719213125,-34.6955813013916));
#18606=CARTESIAN_POINT('Ctrl Pts',(-4.08526205546715,2.17766605746016,-34.4999984402592));
#18607=CARTESIAN_POINT('Ctrl Pts',(-4.07733738453231,-2.19246790435728,
-34.3044155791268));
#18608=CARTESIAN_POINT('Ctrl Pts',(-0.436013896981797,-4.60884876820679,
-34.1088327179944));
#18609=CARTESIAN_POINT('Ctrl Pts',(3.5938504425743,-2.91819032786367,-33.913249856862));
#18610=CARTESIAN_POINT('Ctrl Pts',(4.42116121130352,1.37292755098399,-33.7176669957297));
#18611=CARTESIAN_POINT('Ctrl Pts',(1.30868452313593,4.44060096766705,-33.5220841345973));
#18612=CARTESIAN_POINT('Ctrl Pts',(-2.96998729376919,3.55116521717984,-33.326501273465));
#18613=CARTESIAN_POINT('Ctrl Pts',(-4.60204350868331,-0.502788986694056,
-33.1309184123326));
#18614=CARTESIAN_POINT('Ctrl Pts',(-2.1331228651574,-4.10869277646887,-32.9353355512002));
#18615=CARTESIAN_POINT('Ctrl Pts',(2.23666384406031,-4.05326597551358,-32.7397526900678));
#18616=CARTESIAN_POINT('Ctrl Pts',(4.61332031849898,-0.385871818679268,
-32.5441698289355));
#18617=CARTESIAN_POINT('Ctrl Pts',(2.87893937522212,3.62534276672113,-32.3485869678031));
#18618=CARTESIAN_POINT('Ctrl Pts',(-1.42089706693793,4.40601524243686,-32.1530041066707));
#18619=CARTESIAN_POINT('Ctrl Pts',(-4.45459518642441,1.26024863315421,-31.9574212455384));
#18620=CARTESIAN_POINT('Ctrl Pts',(-3.51860901853861,-3.00825648640842,
-31.761838384406));
#18621=CARTESIAN_POINT('Ctrl Pts',(0.552676769413556,-4.59662717765893,
-31.5662555232737));
#18622=CARTESIAN_POINT('Ctrl Pts',(4.13186726638907,-2.08769049382909,-31.3706726621412));
#18623=CARTESIAN_POINT('Ctrl Pts',(4.02825935404604,2.27933104012005,-31.1750898010089));
#18624=CARTESIAN_POINT('Ctrl Pts',(0.336605165116067,4.61977139809752,-30.9795069398765));
#18625=CARTESIAN_POINT('Ctrl Pts',(-3.6592865373515,2.83374009317316,-30.7838820480532));
#18626=CARTESIAN_POINT('Ctrl Pts',(-4.14193696816894,-0.0273723785633317,
-30.653451443274));
#18627=CARTESIAN_POINT('Ctrl Pts',(-3.73164582215044,-1.25102224755177,
-30.5882151255389));
#18628=CARTESIAN_POINT('Ctrl Pts',(0.65442808399584,3.88366537266789,-31.));
#18629=CARTESIAN_POINT('Ctrl Pts',(0.530799992980382,3.89427684154009,-31.));
#18630=CARTESIAN_POINT('Ctrl Pts',(0.407028067198408,3.89867666407562,-31.));
#18631=CARTESIAN_POINT('Ctrl Pts',(0.283462307316361,3.89662818837984,-31.));
#18632=CARTESIAN_POINT('Ctrl Pts',(0.162992985921285,3.89463104550466,-31.));
#18633=CARTESIAN_POINT('Ctrl Pts',(0.0427188591126211,3.8865043164729,-31.));
#18634=CARTESIAN_POINT('Ctrl Pts',(-0.076989455381779,3.87248877284768,
-31.));
#18635=CARTESIAN_POINT('Ctrl Pts',(-0.1982861832848,3.85828725653111,-31.));
#18636=CARTESIAN_POINT('Ctrl Pts',(-0.319002835924176,3.83803917771155,
-31.));
#18637=CARTESIAN_POINT('Ctrl Pts',(-0.438735032843909,3.81194478664408,
-31.));
#18638=CARTESIAN_POINT('Ctrl Pts',(-0.558467229763642,3.78585039557661,
-31.));
#18639=CARTESIAN_POINT('Ctrl Pts',(-0.677215788457317,3.75390915529031,
-31.));
#18640=CARTESIAN_POINT('Ctrl Pts',(-0.794545113588183,3.71627889103425,
-31.));
#18641=CARTESIAN_POINT('Ctrl Pts',(-0.814657844220622,3.70982826696592,
-31.));
#18642=CARTESIAN_POINT('Ctrl Pts',(-0.83473197297741,3.70320920941588,-31.));
#18643=CARTESIAN_POINT('Ctrl Pts',(-0.854740931745014,3.69643088850593,
-31.));
#18644=CARTESIAN_POINT('Ctrl Pts',(-0.968165833818036,3.65800658095652,
-31.));
#18645=CARTESIAN_POINT('Ctrl Pts',(-1.07965301146909,3.61442076053118,-31.));
#18646=CARTESIAN_POINT('Ctrl Pts',(-1.18884413184658,3.56590670523799,-31.));
#18647=CARTESIAN_POINT('Ctrl Pts',(-1.29790943786314,3.51744854977294,-31.));
#18648=CARTESIAN_POINT('Ctrl Pts',(-1.4046847353241,3.46407295073166,-31.));
#18649=CARTESIAN_POINT('Ctrl Pts',(-1.50878571903602,3.4059682136783,-31.));
#18650=CARTESIAN_POINT('Ctrl Pts',(-1.61069021754416,3.34908946115127,-31.));
#18651=CARTESIAN_POINT('Ctrl Pts',(-1.71003263238448,3.28767841965964,-31.));
#18652=CARTESIAN_POINT('Ctrl Pts',(-1.80641677157113,3.2218782094244,-31.));
#18653=CARTESIAN_POINT('Ctrl Pts',(-1.8932173104265,3.16262059968267,-31.));
#18654=CARTESIAN_POINT('Ctrl Pts',(-1.97761850464391,3.09980260999695,-31.));
#18655=CARTESIAN_POINT('Ctrl Pts',(-2.05929965551334,3.03351053092812,-31.));
#18656=CARTESIAN_POINT('Ctrl Pts',(-2.07743120272542,3.01879504334464,-31.));
#18657=CARTESIAN_POINT('Ctrl Pts',(-2.0954329855743,3.00390448148057,-31.));
#18658=CARTESIAN_POINT('Ctrl Pts',(-2.11327637207231,2.9888610591179,-31.));
#18659=CARTESIAN_POINT('Ctrl Pts',(-2.2012290911024,2.91470978181062,-31.));
#18660=CARTESIAN_POINT('Ctrl Pts',(-2.28543470612264,2.83677091891449,-31.));
#18661=CARTESIAN_POINT('Ctrl Pts',(-2.36554425549263,2.75521673120583,-31.));
#18662=CARTESIAN_POINT('Ctrl Pts',(-2.44359400126818,2.67575949211696,-31.));
#18663=CARTESIAN_POINT('Ctrl Pts',(-2.5177560405726,2.59286986985704,-31.));
#18664=CARTESIAN_POINT('Ctrl Pts',(-2.58766793658226,2.50667951356563,-31.));
#18665=CARTESIAN_POINT('Ctrl Pts',(-2.65718277945497,2.42097866125412,-31.));
#18666=CARTESIAN_POINT('Ctrl Pts',(-2.72249613097522,2.3320140186649,-31.));
#18667=CARTESIAN_POINT('Ctrl Pts',(-2.7832047862205,2.23989471833288,-31.));
#18668=CARTESIAN_POINT('Ctrl Pts',(-2.7947489485025,2.22237760898432,-31.));
#18669=CARTESIAN_POINT('Ctrl Pts',(-2.80612645692971,2.20474638032351,-31.));
#18670=CARTESIAN_POINT('Ctrl Pts',(-2.81733432202403,2.18700171933814,-31.));
#18671=CARTESIAN_POINT('Ctrl Pts',(-2.8680715957088,2.10667279734618,-31.));
#18672=CARTESIAN_POINT('Ctrl Pts',(-2.91533425130486,2.02401925455049,-31.));
#18673=CARTESIAN_POINT('Ctrl Pts',(-2.95906936290355,1.93927703870198,-31.));
#18674=CARTESIAN_POINT('Ctrl Pts',(-2.96640259530189,1.9250679892666,-31.));
#18675=CARTESIAN_POINT('Ctrl Pts',(-2.97363186370474,1.91080938650722,-31.));
#18676=CARTESIAN_POINT('Ctrl Pts',(-2.98075699694485,1.89650307013396,-31.));
#18677=CARTESIAN_POINT('Ctrl Pts',(-3.03037412840343,1.79687849382657,-31.));
#18678=CARTESIAN_POINT('Ctrl Pts',(-3.07495051482241,1.69493226765915,-31.));
#18679=CARTESIAN_POINT('Ctrl Pts',(-3.11450209358653,1.59107365622641,-31.));
#18680=CARTESIAN_POINT('Ctrl Pts',(-3.15440656891242,1.48628837263471,-31.));
#18681=CARTESIAN_POINT('Ctrl Pts',(-3.18919620871934,1.37955547585428,-31.));
#18682=CARTESIAN_POINT('Ctrl Pts',(-3.21883515641334,1.27128356748666,-31.));
#18683=CARTESIAN_POINT('Ctrl Pts',(-3.24825524174243,1.16381116948505,-31.));
#18684=CARTESIAN_POINT('Ctrl Pts',(-3.27260033027765,1.05482148127186,-31.));
#18685=CARTESIAN_POINT('Ctrl Pts',(-3.29178473526898,0.944716681198161,
-31.));
#18686=CARTESIAN_POINT('Ctrl Pts',(-3.30603349555463,0.862938961052112,
-31.));
#18687=CARTESIAN_POINT('Ctrl Pts',(-3.31743436418504,0.780546081363158,
-31.));
#18688=CARTESIAN_POINT('Ctrl Pts',(-3.32593436134209,0.697708237182895,
-31.));
#18689=CARTESIAN_POINT('Ctrl Pts',(-3.32858825065657,0.671844408590687,
-31.));
#18690=CARTESIAN_POINT('Ctrl Pts',(-3.33095964050156,0.645930844620501,
-31.));
#18691=CARTESIAN_POINT('Ctrl Pts',(-3.33304413859681,0.620008089466332,
-31.));
#18692=CARTESIAN_POINT('Ctrl Pts',(-3.34186404098015,0.510324050662291,
-31.));
#18693=CARTESIAN_POINT('Ctrl Pts',(-3.34556409252275,0.400379798786449,
-31.));
#18694=CARTESIAN_POINT('Ctrl Pts',(-3.34408794001819,0.290567571373062,
-31.));
#18695=CARTESIAN_POINT('Ctrl Pts',(-3.34264022976402,0.182871186908495,
-31.));
#18696=CARTESIAN_POINT('Ctrl Pts',(-3.33621365424332,0.0753010039520607,
-31.));
#18697=CARTESIAN_POINT('Ctrl Pts',(-3.3247077506334,-0.0317580568508979,
-31.));
#18698=CARTESIAN_POINT('Ctrl Pts',(-3.31869249632875,-0.0877282351333704,
-31.));
#18699=CARTESIAN_POINT('Ctrl Pts',(-3.3112882052149,-0.143558394636405,
-31.));
#18700=CARTESIAN_POINT('Ctrl Pts',(-3.30247549609232,-0.199190797499773,
-31.));
#18701=CARTESIAN_POINT('Ctrl Pts',(-3.29984045792571,-0.215825126717531,
-31.));
#18702=CARTESIAN_POINT('Ctrl Pts',(-3.29707959885014,-0.232440680412909,
-31.));
#18703=CARTESIAN_POINT('Ctrl Pts',(-3.29419424747565,-0.249026088786987,
-31.));
#18704=CARTESIAN_POINT('Ctrl Pts',(-3.27606532868822,-0.353233681709253,
-31.));
#18705=CARTESIAN_POINT('Ctrl Pts',(-3.2530091964803,-0.456358937838572,
-31.));
#18706=CARTESIAN_POINT('Ctrl Pts',(-3.22494481912661,-0.558036044516438,
-31.));
#18707=CARTESIAN_POINT('Ctrl Pts',(-3.1976427103111,-0.656951455878645,
-31.));
#18708=CARTESIAN_POINT('Ctrl Pts',(-3.16560046250666,-0.754496902145692,
-31.));
#18709=CARTESIAN_POINT('Ctrl Pts',(-3.12870144491393,-0.850310755848633,
-31.));
#18710=CARTESIAN_POINT('Ctrl Pts',(-3.10634825322454,-0.908354182965307,
-31.));
#18711=CARTESIAN_POINT('Ctrl Pts',(-3.08221189711736,-0.965761619215496,
-31.));
#18712=CARTESIAN_POINT('Ctrl Pts',(-3.05625919777042,-1.02244671183575,
-31.));
#18713=CARTESIAN_POINT('',(1.87402501333402,2.62458822954938,-39.0012934619393));
#18714=CARTESIAN_POINT('Ctrl Pts',(1.87544346703979,2.62635034242884,-39.));
#18715=CARTESIAN_POINT('Ctrl Pts',(1.96556023181235,2.57633844914819,-39.));
#18716=CARTESIAN_POINT('Ctrl Pts',(2.05286117778038,2.52194281889414,-39.));
#18717=CARTESIAN_POINT('Ctrl Pts',(2.13698205793886,2.46326372726737,-39.));
#18718=CARTESIAN_POINT('Ctrl Pts',(2.22110684510665,2.40458191027971,-39.));
#18719=CARTESIAN_POINT('Ctrl Pts',(2.30205267959337,2.34161687861634,-39.));
#18720=CARTESIAN_POINT('Ctrl Pts',(2.37974275969731,2.27476660503621,-39.));
#18721=CARTESIAN_POINT('Ctrl Pts',(2.45973180397527,2.20593813316127,-39.));
#18722=CARTESIAN_POINT('Ctrl Pts',(2.53627010144683,2.13299070404304,-39.));
#18723=CARTESIAN_POINT('Ctrl Pts',(2.60925066612413,2.05630756533797,-39.));
#18724=CARTESIAN_POINT('Ctrl Pts',(2.6744743326814,1.98777486089014,-39.));
#18725=CARTESIAN_POINT('Ctrl Pts',(2.73685627038916,1.91625734338406,-39.));
#18726=CARTESIAN_POINT('Ctrl Pts',(2.79629976611078,1.84199988886912,-39.));
#18727=CARTESIAN_POINT('Ctrl Pts',(2.80703184372368,1.82859326202935,-39.));
#18728=CARTESIAN_POINT('Ctrl Pts',(2.81766808406566,1.81509726340499,-39.));
#18729=CARTESIAN_POINT('Ctrl Pts',(2.82820784020875,1.80151325565358,-39.));
#18730=CARTESIAN_POINT('Ctrl Pts',(2.83770979103154,1.78926680783468,-39.));
#18731=CARTESIAN_POINT('Ctrl Pts',(2.84712744324627,1.77695639545417,-39.));
#18732=CARTESIAN_POINT('Ctrl Pts',(2.85645967612864,1.76458452012062,-39.));
#18733=CARTESIAN_POINT('Ctrl Pts',(2.92213524453377,1.67751747464407,-39.));
#18734=CARTESIAN_POINT('Ctrl Pts',(2.98359709732638,1.58739136414667,-39.));
#18735=CARTESIAN_POINT('Ctrl Pts',(3.04075842469254,1.49464028713778,-39.));
#18736=CARTESIAN_POINT('Ctrl Pts',(3.09884554061698,1.40038700768156,-39.));
#18737=CARTESIAN_POINT('Ctrl Pts',(3.15249224301479,1.30342243618241,-39.));
#18738=CARTESIAN_POINT('Ctrl Pts',(3.20157784681904,1.20415578313502,-39.));
#18739=CARTESIAN_POINT('Ctrl Pts',(3.25108154673065,1.10404360720491,-39.));
#18740=CARTESIAN_POINT('Ctrl Pts',(3.29594667342186,1.00158923234391,-39.));
#18741=CARTESIAN_POINT('Ctrl Pts',(3.33601128466594,0.89717595563536,-39.));
#18742=CARTESIAN_POINT('Ctrl Pts',(3.36918521344763,0.810720640137817,-39.));
#18743=CARTESIAN_POINT('Ctrl Pts',(3.39906735707174,0.722921418403139,-39.));
#18744=CARTESIAN_POINT('Ctrl Pts',(3.42554208875469,0.633982806809461,-39.));
#18745=CARTESIAN_POINT('Ctrl Pts',(3.42999792814444,0.619013961287074,-39.));
#18746=CARTESIAN_POINT('Ctrl Pts',(3.4343566153323,0.604014581578844,-39.));
#18747=CARTESIAN_POINT('Ctrl Pts',(3.4386145432116,0.588996991314884,-39.));
#18748=CARTESIAN_POINT('Ctrl Pts',(3.46996387338543,0.478428797361006,-39.));
#18749=CARTESIAN_POINT('Ctrl Pts',(3.49590482509719,0.366708654043199,-39.));
#18750=CARTESIAN_POINT('Ctrl Pts',(3.51631639386122,0.254269119245185,-39.));
#18751=CARTESIAN_POINT('Ctrl Pts',(3.53705216924863,0.140043654010752,-39.));
#18752=CARTESIAN_POINT('Ctrl Pts',(3.5520821545375,0.025074956185946,-39.));
#18753=CARTESIAN_POINT('Ctrl Pts',(3.56123498540351,-0.0902151504387328,
-39.));
#18754=CARTESIAN_POINT('Ctrl Pts',(3.57038781626952,-0.205505257063412,
-39.));
#18755=CARTESIAN_POINT('Ctrl Pts',(3.57366404579988,-0.321117698045253,
-39.));
#18756=CARTESIAN_POINT('Ctrl Pts',(3.57083933718373,-0.436648879008429,
-39.));
#18757=CARTESIAN_POINT('Ctrl Pts',(3.57067942988942,-0.443189121230482,
-39.));
#18758=CARTESIAN_POINT('Ctrl Pts',(3.57049995539871,-0.449729105665625,
-39.));
#18759=CARTESIAN_POINT('Ctrl Pts',(3.57030086735777,-0.456268759879904,
-39.));
#18760=CARTESIAN_POINT('Ctrl Pts',(3.56748577448715,-0.548739075365919,
-39.));
#18761=CARTESIAN_POINT('Ctrl Pts',(3.56075124083497,-0.641143385283898,
-39.));
#18762=CARTESIAN_POINT('Ctrl Pts',(3.55021768944235,-0.733320321140995,
-39.));
#18763=CARTESIAN_POINT('Ctrl Pts',(3.54828067526101,-0.75027073276307,-39.));
#18764=CARTESIAN_POINT('Ctrl Pts',(3.54621613084359,-0.767204492865389,
-39.));
#18765=CARTESIAN_POINT('Ctrl Pts',(3.54402575312891,-0.784116253844053,
-39.));
#18766=CARTESIAN_POINT('Ctrl Pts',(3.52956892168877,-0.895736490018808,
-39.));
#18767=CARTESIAN_POINT('Ctrl Pts',(3.50962805978994,-1.00645761926625,-39.));
#18768=CARTESIAN_POINT('Ctrl Pts',(3.48451903279364,-1.11598728492715,-39.));
#18769=CARTESIAN_POINT('Ctrl Pts',(3.45894659598721,-1.22753841966266,-39.));
#18770=CARTESIAN_POINT('Ctrl Pts',(3.42801334193673,-1.3378543461902,-39.));
#18771=CARTESIAN_POINT('Ctrl Pts',(3.3919981550628,-1.44663447817002,-39.));
#18772=CARTESIAN_POINT('Ctrl Pts',(3.35525611427244,-1.5576099969248,-39.));
#18773=CARTESIAN_POINT('Ctrl Pts',(3.31322480411686,-1.66698785775475,-39.));
#18774=CARTESIAN_POINT('Ctrl Pts',(3.26614584317667,-1.77444675519679,-39.));
#18775=CARTESIAN_POINT('Ctrl Pts',(3.22751572378073,-1.86262096200685,-39.));
#18776=CARTESIAN_POINT('Ctrl Pts',(3.18548600942944,-1.94950332129944,-39.));
#18777=CARTESIAN_POINT('Ctrl Pts',(3.14016485218617,-2.03490971596286,-39.));
#18778=CARTESIAN_POINT('Ctrl Pts',(3.13182152067277,-2.05063248006214,-39.));
#18779=CARTESIAN_POINT('Ctrl Pts',(3.1233665817419,-2.06630519897744,-39.));
#18780=CARTESIAN_POINT('Ctrl Pts',(3.11480063144269,-2.08192668848259,-39.));
#18781=CARTESIAN_POINT('Ctrl Pts',(3.10623133858838,-2.09755427371415,-39.));
#18782=CARTESIAN_POINT('Ctrl Pts',(3.09755504214375,-2.11312309191788,-39.));
#18783=CARTESIAN_POINT('Ctrl Pts',(3.08877426972652,-2.12862929451707,-39.));
#18784=CARTESIAN_POINT('Ctrl Pts',(3.02953329395956,-2.23324452980258,-39.));
#18785=CARTESIAN_POINT('Ctrl Pts',(2.96551860353768,-2.33505128318285,-39.));
#18786=CARTESIAN_POINT('Ctrl Pts',(2.89700764639407,-2.43371931800978,-39.));
#18787=CARTESIAN_POINT('Ctrl Pts',(2.82795254228743,-2.5331710218108,-39.));
#18788=CARTESIAN_POINT('Ctrl Pts',(2.75432915537798,-2.62943477948419,-39.));
#18789=CARTESIAN_POINT('Ctrl Pts',(2.67637106031584,-2.72215810254695,-39.));
#18790=CARTESIAN_POINT('Ctrl Pts',(2.64144532396051,-2.7636987575963,-39.));
#18791=CARTESIAN_POINT('Ctrl Pts',(2.60564892511554,-2.80452854603288,-39.));
#18792=CARTESIAN_POINT('Ctrl Pts',(2.56899987285092,-2.84461416378751,-39.));
#18793=CARTESIAN_POINT('Ctrl Pts',(2.55485781801488,-2.86008231287714,-39.));
#18794=CARTESIAN_POINT('Ctrl Pts',(2.54058712398963,-2.87544139331927,-39.));
#18795=CARTESIAN_POINT('Ctrl Pts',(2.52619415150278,-2.89068374218847,-39.));
#18796=CARTESIAN_POINT('Ctrl Pts',(2.44149799814195,-2.98037809257957,-39.));
#18797=CARTESIAN_POINT('Ctrl Pts',(2.35271110511445,-3.06588609255451,-39.));
#18798=CARTESIAN_POINT('Ctrl Pts',(2.26009625880497,-3.14685732724484,-39.));
#18799=CARTESIAN_POINT('Ctrl Pts',(2.16854211452571,-3.22690121220187,-39.));
#18800=CARTESIAN_POINT('Ctrl Pts',(2.0732467193182,-3.30251241448694,-39.));
#18801=CARTESIAN_POINT('Ctrl Pts',(1.97442050833738,-3.37332724884043,-39.));
#18802=CARTESIAN_POINT('Ctrl Pts',(1.90109880310675,-3.42586659400901,-39.));
#18803=CARTESIAN_POINT('Ctrl Pts',(1.8258326265828,-3.47576531076396,-39.));
#18804=CARTESIAN_POINT('Ctrl Pts',(1.74869447533105,-3.52286199445091,-39.));
#18805=CARTESIAN_POINT('Ctrl Pts',(1.87273482856638,2.62278131463042,-39.0012934619393));
#18806=CARTESIAN_POINT('Ctrl Pts',(1.86214992567493,2.63033921364061,-39.0008623079595));
#18807=CARTESIAN_POINT('Ctrl Pts',(1.85151926948493,2.6378330347527,-39.0004311539798));
#18808=CARTESIAN_POINT('Ctrl Pts',(1.84084363913124,2.64526222873462,-39.));
#18809=CARTESIAN_POINT('Ctrl Pts',(-2.28363142167593,3.20550397776343,-39.4117842388297));
#18810=CARTESIAN_POINT('Ctrl Pts',(-3.33480719872521,2.45671378832311,-39.3465479133207));
#18811=CARTESIAN_POINT('Ctrl Pts',(-4.6260492952095,-0.141677978900424,
-39.2161173007676));
#18812=CARTESIAN_POINT('Ctrl Pts',(-2.44311639859766,-3.9353202317016,-39.0204924011703));
#18813=CARTESIAN_POINT('Ctrl Pts',(1.91917397033554,-4.2117711101878,-38.824909540038));
#18814=CARTESIAN_POINT('Ctrl Pts',(4.56986349694134,-0.739671892207571,
-38.6293266789055));
#18815=CARTESIAN_POINT('Ctrl Pts',(3.14895438396229,3.39389291624858,-38.4337438177732));
#18816=CARTESIAN_POINT('Ctrl Pts',(-1.07840564522595,4.50191710105457,-38.2381609566408));
#18817=CARTESIAN_POINT('Ctrl Pts',(-4.3445982160595,1.59878229949656,-38.0425780955084));
#18818=CARTESIAN_POINT('Ctrl Pts',(-3.73932021527481,-2.72935836966409,
-37.8469952343761));
#18819=CARTESIAN_POINT('Ctrl Pts',(0.198187846293384,-4.62516155268335,
-37.6514123732437));
#18820=CARTESIAN_POINT('Ctrl Pts',(3.95906382568818,-2.39946444773747,-37.4558295121113));
#18821=CARTESIAN_POINT('Ctrl Pts',(4.19194851914756,1.96448277024395,-37.260246650979));
#18822=CARTESIAN_POINT('Ctrl Pts',(0.689296288855085,4.57781990637833,-37.0646637898466));
#18823=CARTESIAN_POINT('Ctrl Pts',(-3.42759904373314,3.11177775663152,-36.8690809287142));
#18824=CARTESIAN_POINT('Ctrl Pts',(-4.49009219582733,-1.12723813956051,
-36.6734980675819));
#18825=CARTESIAN_POINT('Ctrl Pts',(-1.55137155401476,-4.36174658783765,
-36.4779152064495));
#18826=CARTESIAN_POINT('Ctrl Pts',(2.76980765447308,-3.70941463084786,-36.2823323453171));
#18827=CARTESIAN_POINT('Ctrl Pts',(4.62275476464721,0.248453248376883,-36.0867494841847));
#18828=CARTESIAN_POINT('Ctrl Pts',(2.35627039986063,3.98491903692357,-35.8911666230524));
#18829=CARTESIAN_POINT('Ctrl Pts',(-2.00993469357045,4.170342075127,-35.69558376192));
#18830=CARTESIAN_POINT('Ctrl Pts',(-4.5850458702089,0.639487862475723,-35.5000009007876));
#18831=CARTESIAN_POINT('Ctrl Pts',(-3.07432882350545,-3.46122703685094,
-35.3044180396553));
#18832=CARTESIAN_POINT('Ctrl Pts',(1.1759855524789,-4.47757169635789,-35.1088351785229));
#18833=CARTESIAN_POINT('Ctrl Pts',(4.37835513438434,-1.50386059040847,-34.9132523173905));
#18834=CARTESIAN_POINT('Ctrl Pts',(3.67908285493235,2.80997150208605,-34.7176694562581));
#18835=CARTESIAN_POINT('Ctrl Pts',(-0.298695466335132,4.61978040024479,
-34.5220865951258));
#18836=CARTESIAN_POINT('Ctrl Pts',(-4.01030011550478,2.31280859871278,-34.3265037339934));
#18837=CARTESIAN_POINT('Ctrl Pts',(-4.14824431536964,-2.05515460399684,
-34.130920872861));
#18838=CARTESIAN_POINT('Ctrl Pts',(-0.589602992809679,-4.59172683268392,
-33.9353380117287));
#18839=CARTESIAN_POINT('Ctrl Pts',(3.49444539435696,-3.03651858814776,-33.7397551505963));
#18840=CARTESIAN_POINT('Ctrl Pts',(4.4645224279339,1.22459605655993,-33.5441722894639));
#18841=CARTESIAN_POINT('Ctrl Pts',(1.4561712544547,4.39444305307998,-33.3485894283316));
#18842=CARTESIAN_POINT('Ctrl Pts',(-2.84980213881879,3.64832190347186,-33.1530065671991));
#18843=CARTESIAN_POINT('Ctrl Pts',(-4.61626206619028,-0.348913381918043,
-32.9574237060669));
#18844=CARTESIAN_POINT('Ctrl Pts',(-2.2690693624265,-4.03518550246901,-32.7618408449344));
#18845=CARTESIAN_POINT('Ctrl Pts',(2.10012355103143,-4.12569919562993,-32.5662579838021));
#18846=CARTESIAN_POINT('Ctrl Pts',(4.59788102830434,-0.539563295388051,
-32.3706751226697));
#18847=CARTESIAN_POINT('Ctrl Pts',(2.99831780357273,3.52708189147934,-32.1750922615373));
#18848=CARTESIAN_POINT('Ctrl Pts',(-1.2729990573875,4.4512802921326,-31.979509400405));
#18849=CARTESIAN_POINT('Ctrl Pts',(-4.41013611933087,1.40764565774636,-31.7839265392726));
#18850=CARTESIAN_POINT('Ctrl Pts',(-3.61688161784874,-2.88797714248122,
-31.5883436781402));
#18851=CARTESIAN_POINT('Ctrl Pts',(0.398584418807236,-4.6148340733141,-31.3927608170078));
#18852=CARTESIAN_POINT('Ctrl Pts',(4.06075387717163,-2.21958879719896,-31.1971779558755));
#18853=CARTESIAN_POINT('Ctrl Pts',(4.08541618930864,0.680499503299397,-31.0667893817872));
#18854=CARTESIAN_POINT('Ctrl Pts',(3.48785824455754,1.82347842508433,-31.0015950947431));
#18855=CARTESIAN_POINT('Ctrl Pts',(-2.14466679415544,3.01044112214796,-39.2735083224912));
#18856=CARTESIAN_POINT('Ctrl Pts',(-3.13187592188922,2.30721667014621,-39.2082719969821));
#18857=CARTESIAN_POINT('Ctrl Pts',(-4.34454273898582,-0.13305652301272,
-39.0778413844289));
#18858=CARTESIAN_POINT('Ctrl Pts',(-2.29444671526008,-3.69584624961263,
-38.8822164848317));
#18859=CARTESIAN_POINT('Ctrl Pts',(1.80238748132369,-3.95547440750044,-38.6866336236993));
#18860=CARTESIAN_POINT('Ctrl Pts',(4.29177598568882,-0.694661025737465,
-38.4910507625669));
#18861=CARTESIAN_POINT('Ctrl Pts',(2.95733271117712,3.18736612717297,-38.2954679014345));
#18862=CARTESIAN_POINT('Ctrl Pts',(-1.01278199099596,4.22796429626393,-38.0998850403022));
#18863=CARTESIAN_POINT('Ctrl Pts',(-4.08021865502781,1.50149243711901,-37.9043021791698));
#18864=CARTESIAN_POINT('Ctrl Pts',(-3.51177331958788,-2.56327015349656,
-37.7087193180375));
#18865=CARTESIAN_POINT('Ctrl Pts',(0.1861276250257,-4.34370901779091,-37.513136456905));
#18866=CARTESIAN_POINT('Ctrl Pts',(3.71814498710309,-2.25345109371567,-37.3175535957727));
#18867=CARTESIAN_POINT('Ctrl Pts',(3.9368580702165,1.84493912854848,-37.1219707346403));
#18868=CARTESIAN_POINT('Ctrl Pts',(0.647350902606326,4.29924822790718,-36.926387873508));
#18869=CARTESIAN_POINT('Ctrl Pts',(-3.21902115332542,2.92241837368895,-36.7308050123756));
#18870=CARTESIAN_POINT('Ctrl Pts',(-4.21685896580465,-1.05864290711448,
-36.5352221512432));
#18871=CARTESIAN_POINT('Ctrl Pts',(-1.45696675291454,-4.09632350591459,
-36.3396392901108));
#18872=CARTESIAN_POINT('Ctrl Pts',(2.60125799915053,-3.48368756403579,-36.1440564289785));
#18873=CARTESIAN_POINT('Ctrl Pts',(4.34144868876728,0.233334252907989,-35.9484735678461));
#18874=CARTESIAN_POINT('Ctrl Pts',(2.21288551062404,3.74242684470326,-35.7528907067137));
#18875=CARTESIAN_POINT('Ctrl Pts',(-1.88762518977692,3.91656643182389,-35.5573078455814));
#18876=CARTESIAN_POINT('Ctrl Pts',(-4.30603447394324,0.600573442324858,
-35.361724984449));
#18877=CARTESIAN_POINT('Ctrl Pts',(-2.88724830088749,-3.25060279978084,
-35.1661421233167));
#18878=CARTESIAN_POINT('Ctrl Pts',(1.10442391923172,-4.20510036973548,-34.9705592621842));
#18879=CARTESIAN_POINT('Ctrl Pts',(4.11192138127212,-1.41234694910663,-34.7749764010519));
#18880=CARTESIAN_POINT('Ctrl Pts',(3.45520155180266,2.63897777716875,-34.5793935399195));
#18881=CARTESIAN_POINT('Ctrl Pts',(-0.280519107476459,4.3386553218049,-34.3838106787871));
#18882=CARTESIAN_POINT('Ctrl Pts',(-3.76626342179548,2.17206846771106,-34.1882278176548));
#18883=CARTESIAN_POINT('Ctrl Pts',(-3.8958133754738,-1.93009335666479,-33.9926449565224));
#18884=CARTESIAN_POINT('Ctrl Pts',(-0.55372419052002,-4.31230888330598,
-33.7970620953901));
#18885=CARTESIAN_POINT('Ctrl Pts',(3.28179973796592,-2.85173891198998,-33.6014792342576));
#18886=CARTESIAN_POINT('Ctrl Pts',(4.19284518161218,1.15007635375341,-33.4058963731253));
#18887=CARTESIAN_POINT('Ctrl Pts',(1.36755962735034,4.1270303102727,-33.2103135119929));
#18888=CARTESIAN_POINT('Ctrl Pts',(-2.67638462101401,3.42631248041938,-33.0147306508605));
#18889=CARTESIAN_POINT('Ctrl Pts',(-4.3353510870909,-0.327681138529325,
-32.8191477897282));
#18890=CARTESIAN_POINT('Ctrl Pts',(-2.13099087227491,-3.7896344713332,-32.6235649285958));
#18891=CARTESIAN_POINT('Ctrl Pts',(1.9723258319048,-3.87464018210422,-32.4279820674634));
#18892=CARTESIAN_POINT('Ctrl Pts',(4.31808858088176,-0.506729532611965,
-32.232399206331));
#18893=CARTESIAN_POINT('Ctrl Pts',(2.81586273976224,3.31245022341271,-32.0368163451987));
#18894=CARTESIAN_POINT('Ctrl Pts',(-1.19553391210851,4.1804088625691,-31.8412334840663));
#18895=CARTESIAN_POINT('Ctrl Pts',(-4.14176841457767,1.32198693337744,-31.645650622934));
#18896=CARTESIAN_POINT('Ctrl Pts',(-3.39678541403965,-2.71223658116154,
-31.4500677618016));
#18897=CARTESIAN_POINT('Ctrl Pts',(0.374329569811351,-4.33400999111772,
-31.2544849006692));
#18898=CARTESIAN_POINT('Ctrl Pts',(3.81364694711398,-2.08452132198221,-31.0589020395368));
#18899=CARTESIAN_POINT('Ctrl Pts',(3.83680849648018,0.639089423237321,-30.9285134654486));
#18900=CARTESIAN_POINT('Ctrl Pts',(3.27561343254516,1.71251524699515,-30.8633191784045));
#18901=CARTESIAN_POINT('Ctrl Pts',(-2.00570216663496,2.81537826653249,-39.1352324061526));
#18902=CARTESIAN_POINT('Ctrl Pts',(-2.92894464505323,2.15771955196932,-39.0699960806435));
#18903=CARTESIAN_POINT('Ctrl Pts',(-4.06303618276213,-0.124435067125018,
-38.9395654680904));
#18904=CARTESIAN_POINT('Ctrl Pts',(-2.1457770319225,-3.45637226752366,-38.7439405684931));
#18905=CARTESIAN_POINT('Ctrl Pts',(1.68560099231183,-3.69917770481307,-38.5483577073607));
#18906=CARTESIAN_POINT('Ctrl Pts',(4.0136884744363,-0.649650159267356,-38.3527748462284));
#18907=CARTESIAN_POINT('Ctrl Pts',(2.76571103839194,2.98083933809737,-38.157191985096));
#18908=CARTESIAN_POINT('Ctrl Pts',(-0.94715833676596,3.95401149147329,-37.9616091239636));
#18909=CARTESIAN_POINT('Ctrl Pts',(-3.81583909399612,1.40420257474148,-37.7660262628312));
#18910=CARTESIAN_POINT('Ctrl Pts',(-3.28422642390096,-2.39718193732903,
-37.5704434016989));
#18911=CARTESIAN_POINT('Ctrl Pts',(0.174067403758018,-4.06225648289848,
-37.3748605405665));
#18912=CARTESIAN_POINT('Ctrl Pts',(3.477226148518,-2.10743773969387,-37.1792776794341));
#18913=CARTESIAN_POINT('Ctrl Pts',(3.68176762128544,1.72539548685299,-36.9836948183018));
#18914=CARTESIAN_POINT('Ctrl Pts',(0.605405516357568,4.02067654943603,-36.7881119571694));
#18915=CARTESIAN_POINT('Ctrl Pts',(-3.01044326291771,2.73305899074637,-36.592529096037));
#18916=CARTESIAN_POINT('Ctrl Pts',(-3.94362573578198,-0.990047674668459,
-36.3969462349047));
#18917=CARTESIAN_POINT('Ctrl Pts',(-1.36256195181432,-3.8309004239915,-36.2013633737723));
#18918=CARTESIAN_POINT('Ctrl Pts',(2.43270834382797,-3.2579604972237,-36.00578051264));
#18919=CARTESIAN_POINT('Ctrl Pts',(4.06014261288736,0.218215257439091,-35.8101976515075));
#18920=CARTESIAN_POINT('Ctrl Pts',(2.06950062138747,3.49993465248296,-35.6146147903752));
#18921=CARTESIAN_POINT('Ctrl Pts',(-1.76531568598338,3.66279078852076,-35.4190319292428));
#18922=CARTESIAN_POINT('Ctrl Pts',(-4.02702307767759,0.561659022173995,
-35.2234490681104));
#18923=CARTESIAN_POINT('Ctrl Pts',(-2.70016777826954,-3.03997856271072,
-35.0278662069781));
#18924=CARTESIAN_POINT('Ctrl Pts',(1.03286228598455,-3.93262904311309,-34.8322833458457));
#18925=CARTESIAN_POINT('Ctrl Pts',(3.8454876281599,-1.32083330780479,-34.6367004847133));
#18926=CARTESIAN_POINT('Ctrl Pts',(3.23132024867299,2.46798405225144,-34.4411176235809));
#18927=CARTESIAN_POINT('Ctrl Pts',(-0.262342748617795,4.05753024336501,
-34.2455347624486));
#18928=CARTESIAN_POINT('Ctrl Pts',(-3.52222672808616,2.03132833670935,-34.0499519013162));
#18929=CARTESIAN_POINT('Ctrl Pts',(-3.64338243557798,-1.80503210933276,
-33.8543690401839));
#18930=CARTESIAN_POINT('Ctrl Pts',(-0.517845388230359,-4.03289093392803,
-33.6587861790514));
#18931=CARTESIAN_POINT('Ctrl Pts',(3.06915408157487,-2.66695923583222,-33.4632033179192));
#18932=CARTESIAN_POINT('Ctrl Pts',(3.92116793529046,1.07555665094691,-33.2676204567867));
#18933=CARTESIAN_POINT('Ctrl Pts',(1.27894800024599,3.85961756746542,-33.0720375956544));
#18934=CARTESIAN_POINT('Ctrl Pts',(-2.50296710320924,3.2043030573669,-32.8764547345219));
#18935=CARTESIAN_POINT('Ctrl Pts',(-4.05444010799154,-0.306448895140604,
-32.6808718733897));
#18936=CARTESIAN_POINT('Ctrl Pts',(-1.99291238212331,-3.54408344019739,
-32.4852890122572));
#18937=CARTESIAN_POINT('Ctrl Pts',(1.84452811277818,-3.62358116857851,-32.2897061511249));
#18938=CARTESIAN_POINT('Ctrl Pts',(4.03829613345918,-0.473895769835876,
-32.0941232899925));
#18939=CARTESIAN_POINT('Ctrl Pts',(2.63340767595175,3.09781855534609,-31.8985404288602));
#18940=CARTESIAN_POINT('Ctrl Pts',(-1.11806876682953,3.90953743300561,-31.7029575677278));
#18941=CARTESIAN_POINT('Ctrl Pts',(-3.87340070982448,1.23632820900851,-31.5073747065954));
#18942=CARTESIAN_POINT('Ctrl Pts',(-3.17668921023055,-2.53649601984187,
-31.311791845463));
#18943=CARTESIAN_POINT('Ctrl Pts',(0.350074720815462,-4.05318590892136,
-31.1162089843306));
#18944=CARTESIAN_POINT('Ctrl Pts',(3.56654001705634,-1.94945384676547,-30.9206261231983));
#18945=CARTESIAN_POINT('Ctrl Pts',(3.58820080365172,0.597679343175246,-30.79023754911));
#18946=CARTESIAN_POINT('Ctrl Pts',(3.06336862053276,1.60155206890597,-30.7250432620659));
#18947=CARTESIAN_POINT('Ctrl Pts',(-1.86673753911448,2.62031541091702,-38.996956489814));
#18948=CARTESIAN_POINT('Ctrl Pts',(-2.72601336821725,2.00822243379242,-38.9317201643049));
#18949=CARTESIAN_POINT('Ctrl Pts',(-3.78152962653845,-0.115813611237318,
-38.8012895517517));
#18950=CARTESIAN_POINT('Ctrl Pts',(-1.99710734858491,-3.21689828543468,
-38.6056646521545));
#18951=CARTESIAN_POINT('Ctrl Pts',(1.56881450329997,-3.44288100212573,-38.4100817910221));
#18952=CARTESIAN_POINT('Ctrl Pts',(3.73560096318379,-0.604639292797246,
-38.2144989298897));
#18953=CARTESIAN_POINT('Ctrl Pts',(2.57408936560678,2.77431254902176,-38.0189160687574));
#18954=CARTESIAN_POINT('Ctrl Pts',(-0.881534682535969,3.68005868668266,
-37.823333207625));
#18955=CARTESIAN_POINT('Ctrl Pts',(-3.55145953296442,1.30691271236393,-37.6277503464926));
#18956=CARTESIAN_POINT('Ctrl Pts',(-3.05667952821403,-2.23109372116149,
-37.4321674853603));
#18957=CARTESIAN_POINT('Ctrl Pts',(0.162007182490337,-3.78080394800605,
-37.2365846242278));
#18958=CARTESIAN_POINT('Ctrl Pts',(3.23630730993291,-1.96142438567206,-37.0410017630955));
#18959=CARTESIAN_POINT('Ctrl Pts',(3.42667717235439,1.60585184515752,-36.8454189019631));
#18960=CARTESIAN_POINT('Ctrl Pts',(0.563460130108804,3.74210487096489,-36.6498360408308));
#18961=CARTESIAN_POINT('Ctrl Pts',(-2.80186537250999,2.5436996078038,-36.4542531796984));
#18962=CARTESIAN_POINT('Ctrl Pts',(-3.67039250575931,-0.921452442222433,
-36.258670318566));
#18963=CARTESIAN_POINT('Ctrl Pts',(-1.2681571507141,-3.56547734206843,-36.0630874574336));
#18964=CARTESIAN_POINT('Ctrl Pts',(2.26415868850542,-3.03223343041163,-35.8675045963013));
#18965=CARTESIAN_POINT('Ctrl Pts',(3.77883653700745,0.203096261970197,-35.6719217351689));
#18966=CARTESIAN_POINT('Ctrl Pts',(1.92611573215089,3.25744246026265,-35.4763388740365));
#18967=CARTESIAN_POINT('Ctrl Pts',(-1.64300618218985,3.40901514521765,-35.2807560129042));
#18968=CARTESIAN_POINT('Ctrl Pts',(-3.74801168141193,0.522744602023131,
-35.0851731517718));
#18969=CARTESIAN_POINT('Ctrl Pts',(-2.51308725565157,-2.82935432564062,
-34.8895902906395));
#18970=CARTESIAN_POINT('Ctrl Pts',(0.961300652737371,-3.66015771649069,
-34.6940074295071));
#18971=CARTESIAN_POINT('Ctrl Pts',(3.57905387504768,-1.22931966650296,-34.4984245683747));
#18972=CARTESIAN_POINT('Ctrl Pts',(3.00743894554333,2.29699032733414,-34.3028417072423));
#18973=CARTESIAN_POINT('Ctrl Pts',(-0.24416638975912,3.77640516492511,-34.1072588461099));
#18974=CARTESIAN_POINT('Ctrl Pts',(-3.27819003437687,1.89058820570765,-33.9116759849776));
#18975=CARTESIAN_POINT('Ctrl Pts',(-3.39095149568214,-1.67997086200072,
-33.7160931238452));
#18976=CARTESIAN_POINT('Ctrl Pts',(-0.481966585940703,-3.75347298455009,
-33.5205102627128));
#18977=CARTESIAN_POINT('Ctrl Pts',(2.85650842518383,-2.48217955967445,-33.3249274015805));
#18978=CARTESIAN_POINT('Ctrl Pts',(3.64949068896873,1.0010369481404,-33.1293445404481));
#18979=CARTESIAN_POINT('Ctrl Pts',(1.19033637314163,3.59220482465815,-32.9337616793157));
#18980=CARTESIAN_POINT('Ctrl Pts',(-2.32954958540446,2.98229363431442,-32.7381788181833));
#18981=CARTESIAN_POINT('Ctrl Pts',(-3.77352912889216,-0.285216651751885,
-32.542595957051));
#18982=CARTESIAN_POINT('Ctrl Pts',(-1.85483389197172,-3.29853240906158,
-32.3470130959186));
#18983=CARTESIAN_POINT('Ctrl Pts',(1.71673039365155,-3.37252215505281,-32.1514302347862));
#18984=CARTESIAN_POINT('Ctrl Pts',(3.75850368603659,-0.441062007059785,
-31.9558473736539));
#18985=CARTESIAN_POINT('Ctrl Pts',(2.45095261214126,2.88318688727946,-31.7602645125215));
#18986=CARTESIAN_POINT('Ctrl Pts',(-1.04060362155055,3.63866600344211,-31.5646816513891));
#18987=CARTESIAN_POINT('Ctrl Pts',(-3.60503300507128,1.15066948463959,-31.3690987902567));
#18988=CARTESIAN_POINT('Ctrl Pts',(-2.95659300642146,-2.36075545852219,
-31.1735159291244));
#18989=CARTESIAN_POINT('Ctrl Pts',(0.325819871819575,-3.772361826725,-30.977933067992));
#18990=CARTESIAN_POINT('Ctrl Pts',(3.3194330869987,-1.81438637154873,-30.7823502068597));
#18991=CARTESIAN_POINT('Ctrl Pts',(3.33959311082326,0.556269263113169,-30.6519616327714));
#18992=CARTESIAN_POINT('Ctrl Pts',(2.85112380852038,1.49058889081678,-30.5867673457273));
#18993=CARTESIAN_POINT('',(-0.026575674920773,-3.22485156263098,-30.9987013393169));
#18994=CARTESIAN_POINT('Ctrl Pts',(-0.0264634121681443,-3.22711996923596,
-31.));
#18995=CARTESIAN_POINT('Ctrl Pts',(0.0758388090705951,-3.23962881840859,
-31.));
#18996=CARTESIAN_POINT('Ctrl Pts',(0.178439658895469,-3.24693606621664,
-31.));
#18997=CARTESIAN_POINT('Ctrl Pts',(0.280985511217878,-3.24890874069818,
-31.));
#18998=CARTESIAN_POINT('Ctrl Pts',(0.383279979523717,-3.2508765793056,-31.));
#18999=CARTESIAN_POINT('Ctrl Pts',(0.485520482367711,-3.24753728876359,
-31.));
#19000=CARTESIAN_POINT('Ctrl Pts',(0.587413164141851,-3.23916568357852,
-31.));
#19001=CARTESIAN_POINT('Ctrl Pts',(0.692190255801988,-3.23055709237702,
-31.));
#19002=CARTESIAN_POINT('Ctrl Pts',(0.796600205213911,-3.21662724834392,
-31.));
#19003=CARTESIAN_POINT('Ctrl Pts',(0.900334660288271,-3.19762078169955,
-31.));
#19004=CARTESIAN_POINT('Ctrl Pts',(0.956443167896035,-3.18734045123898,
-31.));
#19005=CARTESIAN_POINT('Ctrl Pts',(1.012354186777,-3.1755739904251,-31.));
#19006=CARTESIAN_POINT('Ctrl Pts',(1.06801915047778,-3.16235380686495,-31.));
#19007=CARTESIAN_POINT('Ctrl Pts',(1.10531324032011,-3.15349662488465,-31.));
#19008=CARTESIAN_POINT('Ctrl Pts',(1.14249688454736,-3.14398682690968,-31.));
#19009=CARTESIAN_POINT('Ctrl Pts',(1.17955536555834,-3.13383309957192,-31.));
#19010=CARTESIAN_POINT('Ctrl Pts',(1.19611854884196,-3.12929491985383,-31.));
#19011=CARTESIAN_POINT('Ctrl Pts',(1.21265672752102,-3.12462809653692,-31.));
#19012=CARTESIAN_POINT('Ctrl Pts',(1.22916857715676,-3.11983335183728,-31.));
#19013=CARTESIAN_POINT('Ctrl Pts',(1.24405309889832,-3.11551115394295,-31.));
#19014=CARTESIAN_POINT('Ctrl Pts',(1.2589070195229,-3.11108767246599,-31.));
#19015=CARTESIAN_POINT('Ctrl Pts',(1.2737279671354,-3.10656427085961,-31.));
#19016=CARTESIAN_POINT('Ctrl Pts',(1.37803722183118,-3.07472874572406,-31.));
#19017=CARTESIAN_POINT('Ctrl Pts',(1.48073557027737,-3.03794162316132,-31.));
#19018=CARTESIAN_POINT('Ctrl Pts',(1.58149763038563,-2.99650306755549,-31.));
#19019=CARTESIAN_POINT('Ctrl Pts',(1.68389159427881,-2.95439338895295,-31.));
#19020=CARTESIAN_POINT('Ctrl Pts',(1.78428684038955,-2.90748021838541,-31.));
#19021=CARTESIAN_POINT('Ctrl Pts',(1.88234521022483,-2.85602367353166,-31.));
#19022=CARTESIAN_POINT('Ctrl Pts',(1.98123876893857,-2.80412885977686,-31.));
#19023=CARTESIAN_POINT('Ctrl Pts',(2.07775635551852,-2.7476126815164,-31.));
#19024=CARTESIAN_POINT('Ctrl Pts',(2.17154166571046,-2.6866900413243,-31.));
#19025=CARTESIAN_POINT('Ctrl Pts',(2.24919685881724,-2.63624547405667,-31.));
#19026=CARTESIAN_POINT('Ctrl Pts',(2.32497887842971,-2.58277880173925,-31.));
#19027=CARTESIAN_POINT('Ctrl Pts',(2.398673972733,-2.52638751539726,-31.));
#19028=CARTESIAN_POINT('Ctrl Pts',(2.41107729107925,-2.51689652982941,-31.));
#19029=CARTESIAN_POINT('Ctrl Pts',(2.42341995870474,-2.50732373674807,-31.));
#19030=CARTESIAN_POINT('Ctrl Pts',(2.43569181428942,-2.49767698557919,-31.));
#19031=CARTESIAN_POINT('Ctrl Pts',(2.52604411377092,-2.42665218051856,-31.));
#19032=CARTESIAN_POINT('Ctrl Pts',(2.61269805739617,-2.35151645309661,-31.));
#19033=CARTESIAN_POINT('Ctrl Pts',(2.69530150548317,-2.27254862134861,-31.));
#19034=CARTESIAN_POINT('Ctrl Pts',(2.77921691691963,-2.19232656954756,-31.));
#19035=CARTESIAN_POINT('Ctrl Pts',(2.85895313717407,-2.10814944182442,-31.));
#19036=CARTESIAN_POINT('Ctrl Pts',(2.93412359511511,-2.02025777063396,-31.));
#19037=CARTESIAN_POINT('Ctrl Pts',(3.00929405305615,-1.93236609944351,-31.));
#19038=CARTESIAN_POINT('Ctrl Pts',(3.07989974015383,-1.84075946109991,-31.));
#19039=CARTESIAN_POINT('Ctrl Pts',(3.14552194485315,-1.74563250373385,-31.));
#19040=CARTESIAN_POINT('Ctrl Pts',(3.14923670751426,-1.74024752663795,-31.));
#19041=CARTESIAN_POINT('Ctrl Pts',(3.15293548965499,-1.73485125747499,-31.));
#19042=CARTESIAN_POINT('Ctrl Pts',(3.15661821120802,-1.72944372759524,-31.));
#19043=CARTESIAN_POINT('Ctrl Pts',(3.19985700463249,-1.6659539784952,-31.));
#19044=CARTESIAN_POINT('Ctrl Pts',(3.24088262168145,-1.60091250612483,-31.));
#19045=CARTESIAN_POINT('Ctrl Pts',(3.27969752040755,-1.53443522991608,-31.));
#19046=CARTESIAN_POINT('Ctrl Pts',(3.28816156612781,-1.5199390770558,-31.));
#19047=CARTESIAN_POINT('Ctrl Pts',(3.29652094980811,-1.50537374488921,-31.));
#19048=CARTESIAN_POINT('Ctrl Pts',(3.3047740963749,-1.49074312709972,-31.));
#19049=CARTESIAN_POINT('Ctrl Pts',(3.31263779296697,-1.47680289977913,-31.));
#19050=CARTESIAN_POINT('Ctrl Pts',(3.32040197057988,-1.46280884199712,-31.));
#19051=CARTESIAN_POINT('Ctrl Pts',(3.32806517242938,-1.44876535269138,-31.));
#19052=CARTESIAN_POINT('Ctrl Pts',(3.38197815672864,-1.34996508182343,-31.));
#19053=CARTESIAN_POINT('Ctrl Pts',(3.43092600979739,-1.24866875081712,-31.));
#19054=CARTESIAN_POINT('Ctrl Pts',(3.4749924224499,-1.14529854716208,-31.));
#19055=CARTESIAN_POINT('Ctrl Pts',(3.51987212649102,-1.04002053909523,-31.));
#19056=CARTESIAN_POINT('Ctrl Pts',(3.55968881815558,-0.932590809276557,
-31.));
#19057=CARTESIAN_POINT('Ctrl Pts',(3.59449143272375,-0.823416466411623,
-31.));
#19058=CARTESIAN_POINT('Ctrl Pts',(3.62999642302698,-0.712038800311621,
-31.));
#19059=CARTESIAN_POINT('Ctrl Pts',(3.66028323731959,-0.598844700472671,
-31.));
#19060=CARTESIAN_POINT('Ctrl Pts',(3.68535848353317,-0.484236133285269,
-31.));
#19061=CARTESIAN_POINT('Ctrl Pts',(3.70593368219157,-0.390195420075543,
-31.));
#19062=CARTESIAN_POINT('Ctrl Pts',(3.72299923124982,-0.295201598735365,
-31.));
#19063=CARTESIAN_POINT('Ctrl Pts',(3.73653440245394,-0.199467195515414,
-31.));
#19064=CARTESIAN_POINT('Ctrl Pts',(3.73902614120766,-0.18184310203554,-31.));
#19065=CARTESIAN_POINT('Ctrl Pts',(3.74139817189912,-0.164193894712116,
-31.));
#19066=CARTESIAN_POINT('Ctrl Pts',(3.74365028064763,-0.146520881969029,
-31.));
#19067=CARTESIAN_POINT('Ctrl Pts',(3.745903251544,-0.128841103677876,-31.));
#19068=CARTESIAN_POINT('Ctrl Pts',(3.7480351141005,-0.111145974267687,-31.));
#19069=CARTESIAN_POINT('Ctrl Pts',(3.75004565109281,-0.0934400925234178,
-31.));
#19070=CARTESIAN_POINT('Ctrl Pts',(3.76361018597104,0.0260165757139654,
-31.));
#19071=CARTESIAN_POINT('Ctrl Pts',(3.77166191629321,0.146007054496315,-31.));
#19072=CARTESIAN_POINT('Ctrl Pts',(3.77423118674206,0.26610109164289,-31.));
#19073=CARTESIAN_POINT('Ctrl Pts',(3.7768208619918,0.387148899505717,-31.));
#19074=CARTESIAN_POINT('Ctrl Pts',(3.77384088651866,0.508302769592539,-31.));
#19075=CARTESIAN_POINT('Ctrl Pts',(3.76527303135289,0.629140236416144,-31.));
#19076=CARTESIAN_POINT('Ctrl Pts',(3.76143457294323,0.683276257830769,-31.));
#19077=CARTESIAN_POINT('Ctrl Pts',(3.75647389257586,0.737348936727639,-31.));
#19078=CARTESIAN_POINT('Ctrl Pts',(3.75038598358214,0.791320743572583,-31.));
#19079=CARTESIAN_POINT('Ctrl Pts',(3.74803679376988,0.812147273489508,-31.));
#19080=CARTESIAN_POINT('Ctrl Pts',(3.74551942283083,0.832961176947892,-31.));
#19081=CARTESIAN_POINT('Ctrl Pts',(3.74283451253955,0.853752515419332,-31.));
#19082=CARTESIAN_POINT('Ctrl Pts',(3.72703504525638,0.976100019177537,-31.));
#19083=CARTESIAN_POINT('Ctrl Pts',(3.70546540675222,1.09746515777843,-31.));
#19084=CARTESIAN_POINT('Ctrl Pts',(3.6781322195357,1.21740997293571,-31.));
#19085=CARTESIAN_POINT('Ctrl Pts',(3.65111210442695,1.33598094991597,-31.));
#19086=CARTESIAN_POINT('Ctrl Pts',(3.61845977551099,1.45316484915809,-31.));
#19087=CARTESIAN_POINT('Ctrl Pts',(3.58013170248686,1.56854374917087,-31.));
#19088=CARTESIAN_POINT('Ctrl Pts',(3.55169508562206,1.65414642405306,-31.));
#19089=CARTESIAN_POINT('Ctrl Pts',(3.52013321748227,1.73875570516642,-31.));
#19090=CARTESIAN_POINT('Ctrl Pts',(3.48540987471234,1.82219839898341,-31.));
#19091=CARTESIAN_POINT('Ctrl Pts',(-0.065570273740064,-3.22208288250033,
-31.));
#19092=CARTESIAN_POINT('Ctrl Pts',(-0.0525672847650432,-3.22234749690587,
-30.9995671131056));
#19093=CARTESIAN_POINT('Ctrl Pts',(-0.0395626939642705,-3.22253339835127,
-30.9991342262113));
#19094=CARTESIAN_POINT('Ctrl Pts',(-0.026557454381041,-3.22264057321272,
-30.9987013393169));
#19095=CARTESIAN_POINT('Ctrl Pts',(-1.75281221119047,-3.52691927538468,
-39.));
#19096=CARTESIAN_POINT('Ctrl Pts',(-1.85924677934811,-3.46275184993558,
-39.));
#19097=CARTESIAN_POINT('Ctrl Pts',(-1.96213599398535,-3.3934582774933,-39.));
#19098=CARTESIAN_POINT('Ctrl Pts',(-2.06105560704088,-3.31905293948038,
-39.));
#19099=CARTESIAN_POINT('Ctrl Pts',(-2.15734339103454,-3.24662721021129,
-39.));
#19100=CARTESIAN_POINT('Ctrl Pts',(-2.24987036069143,-3.16935730201866,
-39.));
#19101=CARTESIAN_POINT('Ctrl Pts',(-2.33847820579006,-3.08765584052718,
-39.));
#19102=CARTESIAN_POINT('Ctrl Pts',(-2.42826178589376,-3.00487028464052,
-39.));
#19103=CARTESIAN_POINT('Ctrl Pts',(-2.51402198065837,-2.91753393939187,
-39.));
#19104=CARTESIAN_POINT('Ctrl Pts',(-2.59554934753375,-2.82604649297915,
-39.));
#19105=CARTESIAN_POINT('Ctrl Pts',(-2.67707671440914,-2.73455904656643,
-39.));
#19106=CARTESIAN_POINT('Ctrl Pts',(-2.75437159913114,-2.6389195840714,-39.));
#19107=CARTESIAN_POINT('Ctrl Pts',(-2.82717436902469,-2.53951181872049,
-39.));
#19108=CARTESIAN_POINT('Ctrl Pts',(-2.83965430798123,-2.52247121923232,
-39.));
#19109=CARTESIAN_POINT('Ctrl Pts',(-2.8520040143943,-2.5053170440578,-39.));
#19110=CARTESIAN_POINT('Ctrl Pts',(-2.86420738431601,-2.4880723282558,-39.));
#19111=CARTESIAN_POINT('Ctrl Pts',(-2.93338468399664,-2.39031712779931,
-39.));
#19112=CARTESIAN_POINT('Ctrl Pts',(-2.99796046584097,-2.28952514865008,
-39.));
#19113=CARTESIAN_POINT('Ctrl Pts',(-3.05778195366412,-2.18609573317179,
-39.));
#19114=CARTESIAN_POINT('Ctrl Pts',(-3.11753452619717,-2.08278546999867,
-39.));
#19115=CARTESIAN_POINT('Ctrl Pts',(-3.17254403905503,-1.97684294431477,
-39.));
#19116=CARTESIAN_POINT('Ctrl Pts',(-3.22261026970107,-1.86864638142994,
-39.));
#19117=CARTESIAN_POINT('Ctrl Pts',(-3.271620158212,-1.76273264644676,-39.));
#19118=CARTESIAN_POINT('Ctrl Pts',(-3.31589325903411,-1.65465815862718,
-39.));
#19119=CARTESIAN_POINT('Ctrl Pts',(-3.35519317305696,-1.54477157537668,
-39.));
#19120=CARTESIAN_POINT('Ctrl Pts',(-3.39058551444191,-1.44581096529071,
-39.));
#19121=CARTESIAN_POINT('Ctrl Pts',(-3.4219439883879,-1.34538022953061,-39.));
#19122=CARTESIAN_POINT('Ctrl Pts',(-3.44905986541963,-1.24373767821722,
-39.));
#19123=CARTESIAN_POINT('Ctrl Pts',(-3.45507889936618,-1.22117562108541,
-39.));
#19124=CARTESIAN_POINT('Ctrl Pts',(-3.46089005423046,-1.19854820161701,
-39.));
#19125=CARTESIAN_POINT('Ctrl Pts',(-3.46648322368768,-1.17589021910338,
-39.));
#19126=CARTESIAN_POINT('Ctrl Pts',(-3.49403430178266,-1.06428054046186,
-39.));
#19127=CARTESIAN_POINT('Ctrl Pts',(-3.51633488607024,-0.951810304057931,
-39.));
#19128=CARTESIAN_POINT('Ctrl Pts',(-3.53320430915353,-0.838823268609796,
-39.));
#19129=CARTESIAN_POINT('Ctrl Pts',(-3.54982973534889,-0.727470461249351,
-39.));
#19130=CARTESIAN_POINT('Ctrl Pts',(-3.5611800757903,-0.615614942649066,
-39.));
#19131=CARTESIAN_POINT('Ctrl Pts',(-3.56703215600623,-0.503586796080013,
-39.));
#19132=CARTESIAN_POINT('Ctrl Pts',(-3.57272988890964,-0.394513366929766,
-39.));
#19133=CARTESIAN_POINT('Ctrl Pts',(-3.57321554812162,-0.285275688187582,
-39.));
#19134=CARTESIAN_POINT('Ctrl Pts',(-3.56823476358766,-0.176189271538187,
-39.));
#19135=CARTESIAN_POINT('Ctrl Pts',(-3.56727789656693,-0.155232493787625,
-39.));
#19136=CARTESIAN_POINT('Ctrl Pts',(-3.56611913357304,-0.134281346867122,
-39.));
#19137=CARTESIAN_POINT('Ctrl Pts',(-3.56475645999484,-0.113338143574554,
-39.));
#19138=CARTESIAN_POINT('Ctrl Pts',(-3.56024904482747,-0.0440627766162007,
-39.));
#19139=CARTESIAN_POINT('Ctrl Pts',(-3.55351098219617,0.0251259798909786,
-39.));
#19140=CARTESIAN_POINT('Ctrl Pts',(-3.54458068183499,0.0941423097710962,
-39.));
#19141=CARTESIAN_POINT('Ctrl Pts',(-3.54202177207861,0.113918415023707,
-39.));
#19142=CARTESIAN_POINT('Ctrl Pts',(-3.53928283006026,0.133680337115747,
-39.));
#19143=CARTESIAN_POINT('Ctrl Pts',(-3.53636467707845,0.15342599149552,-39.));
#19144=CARTESIAN_POINT('Ctrl Pts',(-3.53393720844056,0.16985143493198,-39.));
#19145=CARTESIAN_POINT('Ctrl Pts',(-3.53138560410875,0.186265940392125,
-39.));
#19146=CARTESIAN_POINT('Ctrl Pts',(-3.52871303514421,0.202652981912964,
-39.));
#19147=CARTESIAN_POINT('Ctrl Pts',(-3.52789260432643,0.207683510237725,
-39.));
#19148=CARTESIAN_POINT('Ctrl Pts',(-3.52706072562481,0.21271179145904,-39.));
#19149=CARTESIAN_POINT('Ctrl Pts',(-3.5262174297509,0.217737774115531,-39.));
#19150=CARTESIAN_POINT('Ctrl Pts',(-3.50784848795626,0.327215343891981,
-39.));
#19151=CARTESIAN_POINT('Ctrl Pts',(-3.48406506021569,0.435613933294974,
-39.));
#19152=CARTESIAN_POINT('Ctrl Pts',(-3.45511869430776,0.542614318777618,
-39.));
#19153=CARTESIAN_POINT('Ctrl Pts',(-3.42583968563334,0.650844319900267,
-39.));
#19154=CARTESIAN_POINT('Ctrl Pts',(-3.39127789178026,0.757644593911477,
-39.));
#19155=CARTESIAN_POINT('Ctrl Pts',(-3.35164455227839,0.862663619089397,
-39.));
#19156=CARTESIAN_POINT('Ctrl Pts',(-3.31212647970358,0.967377214029349,
-39.));
#19157=CARTESIAN_POINT('Ctrl Pts',(-3.26756572112307,1.07032063431149,-39.));
#19158=CARTESIAN_POINT('Ctrl Pts',(-3.21813160441969,1.17111310733081,-39.));
#19159=CARTESIAN_POINT('Ctrl Pts',(-3.19429583585514,1.21971245976496,-39.));
#19160=CARTESIAN_POINT('Ctrl Pts',(-3.16932651798421,1.26781118858304,-39.));
#19161=CARTESIAN_POINT('Ctrl Pts',(-3.14323990782853,1.31536315285873,-39.));
#19162=CARTESIAN_POINT('Ctrl Pts',(-3.12740697868958,1.3442241998212,-39.));
#19163=CARTESIAN_POINT('Ctrl Pts',(-3.11116300262372,1.3728828286187,-39.));
#19164=CARTESIAN_POINT('Ctrl Pts',(-3.09450947007563,1.401331437924,-39.));
#19165=CARTESIAN_POINT('Ctrl Pts',(-3.08121617070089,1.42403988606846,-39.));
#19166=CARTESIAN_POINT('Ctrl Pts',(-3.06766332150694,1.44661163127224,-39.));
#19167=CARTESIAN_POINT('Ctrl Pts',(-3.05386840941538,1.46901669000711,-39.));
#19168=CARTESIAN_POINT('Ctrl Pts',(-2.99619963659367,1.56267964586087,-39.));
#19169=CARTESIAN_POINT('Ctrl Pts',(-2.93424670289176,1.65353184103952,-39.));
#19170=CARTESIAN_POINT('Ctrl Pts',(-2.86819294799962,1.74122159681554,-39.));
#19171=CARTESIAN_POINT('Ctrl Pts',(-2.80342392707767,1.82720580219149,-39.));
#19172=CARTESIAN_POINT('Ctrl Pts',(-2.73471142703462,1.91014989765233,-39.));
#19173=CARTESIAN_POINT('Ctrl Pts',(-2.66219917441839,1.98968213489971,-39.));
#19174=CARTESIAN_POINT('Ctrl Pts',(-2.62723747571619,2.02802851106971,-39.));
#19175=CARTESIAN_POINT('Ctrl Pts',(-2.59139207824707,2.06558109012876,-39.));
#19176=CARTESIAN_POINT('Ctrl Pts',(-2.55467723691739,2.102294244759,-39.));
#19177=CARTESIAN_POINT('Ctrl Pts',(-2.54276804759259,2.11420288696928,-39.));
#19178=CARTESIAN_POINT('Ctrl Pts',(-2.53076810266377,2.1260223834559,-39.));
#19179=CARTESIAN_POINT('Ctrl Pts',(-2.51868516007585,2.13774431665332,-39.));
#19180=CARTESIAN_POINT('Ctrl Pts',(-2.44276707797251,2.21139414825824,-39.));
#19181=CARTESIAN_POINT('Ctrl Pts',(-2.36349897831715,2.28127220136821,-39.));
#19182=CARTESIAN_POINT('Ctrl Pts',(-2.28103031984326,2.34703489324668,-39.));
#19183=CARTESIAN_POINT('Ctrl Pts',(-2.20080167582135,2.41101133828986,-39.));
#19184=CARTESIAN_POINT('Ctrl Pts',(-2.11754342366811,2.4710932686734,-39.));
#19185=CARTESIAN_POINT('Ctrl Pts',(-2.03137376194493,2.52691956397708,-39.));
#19186=CARTESIAN_POINT('Ctrl Pts',(-1.97917218845064,2.56073912876277,-39.));
#19187=CARTESIAN_POINT('Ctrl Pts',(-1.92590180692628,2.59299601272173,-39.));
#19188=CARTESIAN_POINT('Ctrl Pts',(-1.87158653173895,2.62360084935064,-39.));
#19189=CARTESIAN_POINT('Origin',(0.,0.,-31.));
#19190=CARTESIAN_POINT('Origin',(0.,0.,-39.));
#34389=UNCERTAINTY_MEASURE_WITH_UNIT(LENGTH_MEASURE(0.01),#34404,
'DISTANCE_ACCURACY_VALUE',
'Maximum model space distance between geometric entities at asserted c
onnectivities');
#34393=UNCERTAINTY_MEASURE_WITH_UNIT(LENGTH_MEASURE(0.01),#34404,
'DISTANCE_ACCURACY_VALUE',
'Maximum model space distance between geometric entities at asserted c
onnectivities');
#34399=(
GEOMETRIC_REPRESENTATION_CONTEXT(3)
GLOBAL_UNCERTAINTY_ASSIGNED_CONTEXT((#34389))
GLOBAL_UNIT_ASSIGNED_CONTEXT((#34404,#34406,#34407))
REPRESENTATION_CONTEXT('','3D')
);
#34403=(
GEOMETRIC_REPRESENTATION_CONTEXT(3)
GLOBAL_UNCERTAINTY_ASSIGNED_CONTEXT((#34393))
GLOBAL_UNIT_ASSIGNED_CONTEXT((#34404,#34406,#34407))
REPRESENTATION_CONTEXT('','3D')
);
#34404=(
LENGTH_UNIT()
NAMED_UNIT(*)
SI_UNIT(.MILLI.,.METRE.)
);
#34406=(
NAMED_UNIT(*)
PLANE_ANGLE_UNIT()
SI_UNIT($,.RADIAN.)
);
#34407=(
NAMED_UNIT(*)
SI_UNIT($,.STERADIAN.)
SOLID_ANGLE_UNIT()
);
#34413=SHAPE_DEFINITION_REPRESENTATION(#34422,#34439);
#34422=PRODUCT_DEFINITION_SHAPE('',$,#34449);
#34439=SHAPE_REPRESENTATION('',(#4557),#34399);
#34443=PRODUCT_DEFINITION_CONTEXT('part definition',#34472,'design');
#34449=PRODUCT_DEFINITION('Bushing_01','Bushing_01',#34458,#34443);
#34458=PRODUCT_DEFINITION_FORMATION('',$,#34479);
#34472=APPLICATION_CONTEXT(
'Core Data for Automotive Mechanical Design Process');
#34473=PRODUCT_CONTEXT('part definition',#34472,'mechanical');
#34479=PRODUCT('Bushing_01','Bushing_01',$,(#34473));
#34484=PRESENTATION_STYLE_ASSIGNMENT((#34486));
#34486=SURFACE_STYLE_USAGE(.BOTH.,#34488);
#34488=SURFACE_SIDE_STYLE('',(#34490));
#34490=SURFACE_STYLE_FILL_AREA(#34492);
#34492=FILL_AREA_STYLE('Opaque(160,160,160)',(#34494));
#34494=FILL_AREA_STYLE_COLOUR('Opaque(160,160,160)',#34496);
#34496=COLOUR_RGB('Opaque(160,160,160)', 0.09019608, 0.27058824, 0.51372549);
ENDSEC;
END-ISO-10303-21;
